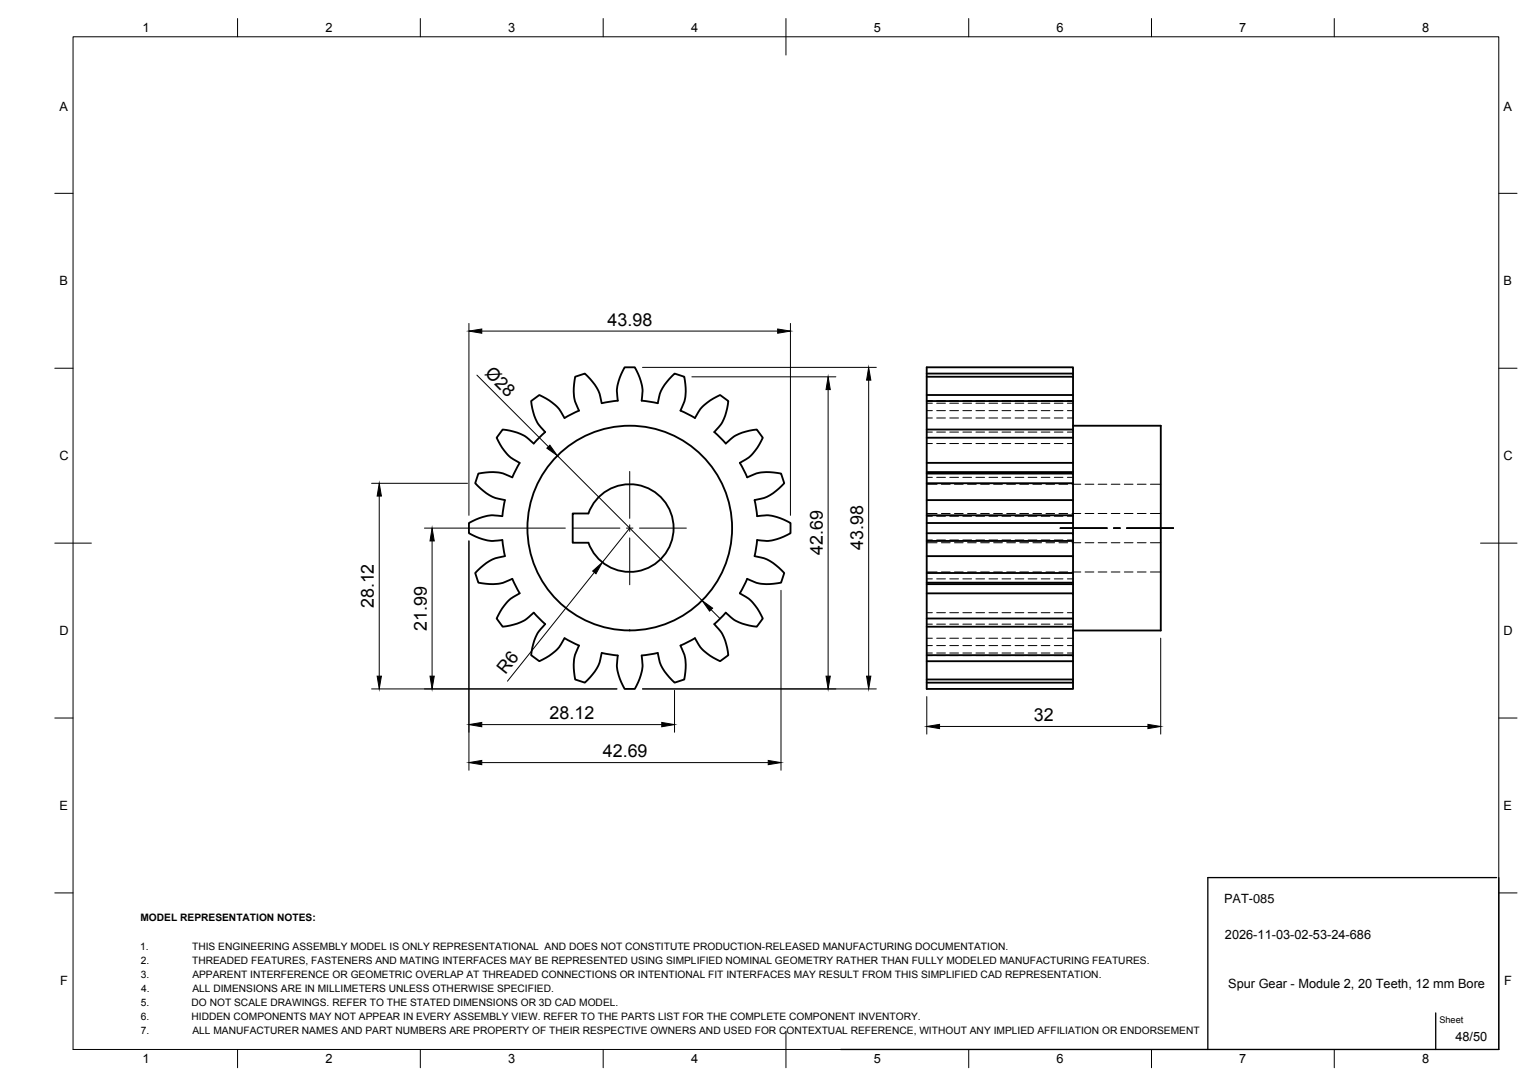
ISO-10303-21;
HEADER;
/* Generated by software containing ST-Developer
 * from STEP Tools, Inc. (www.steptools.com) 
 */

FILE_DESCRIPTION(
/* description */ ('Rack and pinion manual slide'),
/* implementation_level */ '2;1');

FILE_NAME(
/* name */ 'Spur Gear - Module 2, 20 Teeth, 12 mm Bore.step',
/* time_stamp */ '2026-10-28T03:22:49-07:00',
/* author */ (''),
/* organization */ (''),
/* preprocessor_version */ 'ST-DEVELOPER v20.2',
/* originating_system */ 'Autodesk Translation Framework v15.17.0.0',
/* authorisation */ '');

FILE_SCHEMA (('AUTOMOTIVE_DESIGN { 1 0 10303 214 3 1 1 }'));
ENDSEC;

DATA;
#10=MECHANICAL_DESIGN_GEOMETRIC_PRESENTATION_REPRESENTATION('',(#779),#34851);
#11=(
BOUNDED_SURFACE()
B_SPLINE_SURFACE(5,1,((#25778,#25779),(#25780,#25781),(#25782,#25783),(#25784,
#25785),(#25786,#25787),(#25788,#25789),(#25790,#25791),(#25792,#25793),
(#25794,#25795),(#25796,#25797),(#25798,#25799),(#25800,#25801),(#25802,
#25803),(#25804,#25805),(#25806,#25807),(#25808,#25809),(#25810,#25811),
(#25812,#25813),(#25814,#25815),(#25816,#25817),(#25818,#25819),(#25820,
#25821),(#25822,#25823),(#25824,#25825),(#25826,#25827),(#25828,#25829),
(#25830,#25831),(#25832,#25833),(#25834,#25835),(#25836,#25837),(#25838,
#25839),(#25840,#25841),(#25842,#25843),(#25844,#25845),(#25846,#25847),
(#25848,#25849),(#25850,#25851),(#25852,#25853),(#25854,#25855),(#25856,
#25857),(#25858,#25859),(#25860,#25861),(#25862,#25863),(#25864,#25865),
(#25866,#25867),(#25868,#25869),(#25870,#25871),(#25872,#25873),(#25874,
#25875),(#25876,#25877),(#25878,#25879),(#25880,#25881),(#25882,#25883),
(#25884,#25885),(#25886,#25887),(#25888,#25889),(#25890,#25891),(#25892,
#25893),(#25894,#25895),(#25896,#25897),(#25898,#25899),(#25900,#25901),
(#25902,#25903),(#25904,#25905),(#25906,#25907),(#25908,#25909),(#25910,
#25911),(#25912,#25913),(#25914,#25915),(#25916,#25917)),.UNSPECIFIED.,
 .F.,.F.,.F.)
B_SPLINE_SURFACE_WITH_KNOTS((6,1,1,1,1,1,1,1,1,1,1,1,1,1,1,1,1,1,1,1,1,
1,1,1,1,1,1,1,1,1,1,1,1,1,1,1,1,1,1,1,1,1,1,1,1,1,1,1,1,1,1,1,1,1,1,1,1,
1,1,1,1,1,1,1,1,6),(2,2),(-1.,-0.984615384615383,-0.969230769230768,-0.953846153846152,
-0.938461538461537,-0.923076923076922,-0.907692307692306,-0.892307692307691,
-0.876923076923076,-0.86153846153846,-0.846153846153845,-0.83076923076923,
-0.815384615384614,-0.799999999999999,-0.784615384615384,-0.769230769230768,
-0.753846153846153,-0.738461538461538,-0.723076923076922,-0.707692307692307,
-0.692307692307692,-0.676923076923076,-0.661538461538461,-0.646153846153846,
-0.63076923076923,-0.615384615384615,-0.6,-0.584615384615384,-0.569230769230769,
-0.553846153846154,-0.538461538461538,-0.523076923076923,-0.507692307692308,
-0.492307692307692,-0.476923076923077,-0.461538461538462,-0.446153846153846,
-0.430769230769231,-0.415384615384615,-0.4,-0.384615384615385,-0.369230769230769,
-0.353846153846154,-0.338461538461538,-0.323076923076923,-0.307692307692308,
-0.292307692307692,-0.276923076923077,-0.261538461538462,-0.246153846153846,
-0.230769230769231,-0.215384615384615,-0.2,-0.184615384615385,-0.169230769230769,
-0.153846153846154,-0.138461538461538,-0.123076923076923,-0.107692307692308,
-0.0923076923076923,-0.0769230769230769,-0.0615384615384615,-0.0461538461538462,
-0.0307692307692308,-0.0153846153846154,0.),(-1.,1.),.UNSPECIFIED.)
GEOMETRIC_REPRESENTATION_ITEM()
RATIONAL_B_SPLINE_SURFACE(((1.,1.),(1.,1.),(1.,1.),(1.,1.),(1.,1.),(1.,
1.),(1.,1.),(1.,1.),(1.,1.),(1.,1.),(1.,1.),(1.,1.),(1.,1.),(1.,1.),(1.,
1.),(1.,1.),(1.,1.),(1.,1.),(1.,1.),(1.,1.),(1.,1.),(1.,1.),(1.,1.),(1.,
1.),(1.,1.),(1.,1.),(1.,1.),(1.,1.),(1.,1.),(1.,1.),(1.,1.),(1.,1.),(1.,
1.),(1.,1.),(1.,1.),(1.,1.),(1.,1.),(1.,1.),(1.,1.),(1.,1.),(1.,1.),(1.,
1.),(1.,1.),(1.,1.),(1.,1.),(1.,1.),(1.,1.),(1.,1.),(1.,1.),(1.,1.),(1.,
1.),(1.,1.),(1.,1.),(1.,1.),(1.,1.),(1.,1.),(1.,1.),(1.,1.),(1.,1.),(1.,
1.),(1.,1.),(1.,1.),(1.,1.),(1.,1.),(1.,1.),(1.,1.),(1.,1.),(1.,1.),(1.,
1.),(1.,1.)))
REPRESENTATION_ITEM('')
SURFACE()
);
#12=(
BOUNDED_SURFACE()
B_SPLINE_SURFACE(5,1,((#25996,#25997),(#25998,#25999),(#26000,#26001),(#26002,
#26003),(#26004,#26005),(#26006,#26007),(#26008,#26009),(#26010,#26011),
(#26012,#26013),(#26014,#26015),(#26016,#26017),(#26018,#26019),(#26020,
#26021),(#26022,#26023),(#26024,#26025),(#26026,#26027),(#26028,#26029),
(#26030,#26031),(#26032,#26033),(#26034,#26035),(#26036,#26037),(#26038,
#26039),(#26040,#26041),(#26042,#26043),(#26044,#26045),(#26046,#26047),
(#26048,#26049),(#26050,#26051),(#26052,#26053),(#26054,#26055),(#26056,
#26057),(#26058,#26059),(#26060,#26061),(#26062,#26063),(#26064,#26065),
(#26066,#26067),(#26068,#26069),(#26070,#26071),(#26072,#26073),(#26074,
#26075),(#26076,#26077),(#26078,#26079),(#26080,#26081),(#26082,#26083),
(#26084,#26085),(#26086,#26087),(#26088,#26089),(#26090,#26091),(#26092,
#26093),(#26094,#26095),(#26096,#26097),(#26098,#26099),(#26100,#26101),
(#26102,#26103),(#26104,#26105),(#26106,#26107),(#26108,#26109),(#26110,
#26111),(#26112,#26113),(#26114,#26115),(#26116,#26117),(#26118,#26119),
(#26120,#26121),(#26122,#26123),(#26124,#26125),(#26126,#26127),(#26128,
#26129),(#26130,#26131),(#26132,#26133),(#26134,#26135)),.UNSPECIFIED.,
 .F.,.F.,.F.)
B_SPLINE_SURFACE_WITH_KNOTS((6,1,1,1,1,1,1,1,1,1,1,1,1,1,1,1,1,1,1,1,1,
1,1,1,1,1,1,1,1,1,1,1,1,1,1,1,1,1,1,1,1,1,1,1,1,1,1,1,1,1,1,1,1,1,1,1,1,
1,1,1,1,1,1,1,1,6),(2,2),(-1.,-0.984615384615383,-0.969230769230768,-0.953846153846152,
-0.938461538461537,-0.923076923076922,-0.907692307692306,-0.892307692307691,
-0.876923076923076,-0.86153846153846,-0.846153846153845,-0.83076923076923,
-0.815384615384614,-0.799999999999999,-0.784615384615384,-0.769230769230768,
-0.753846153846153,-0.738461538461538,-0.723076923076922,-0.707692307692307,
-0.692307692307692,-0.676923076923076,-0.661538461538461,-0.646153846153846,
-0.63076923076923,-0.615384615384615,-0.6,-0.584615384615384,-0.569230769230769,
-0.553846153846154,-0.538461538461538,-0.523076923076923,-0.507692307692308,
-0.492307692307692,-0.476923076923077,-0.461538461538462,-0.446153846153846,
-0.430769230769231,-0.415384615384615,-0.4,-0.384615384615385,-0.369230769230769,
-0.353846153846154,-0.338461538461538,-0.323076923076923,-0.307692307692308,
-0.292307692307692,-0.276923076923077,-0.261538461538462,-0.246153846153846,
-0.230769230769231,-0.215384615384615,-0.2,-0.184615384615385,-0.169230769230769,
-0.153846153846154,-0.138461538461538,-0.123076923076923,-0.107692307692308,
-0.0923076923076923,-0.0769230769230769,-0.0615384615384615,-0.0461538461538462,
-0.0307692307692308,-0.0153846153846154,0.),(-1.,1.),.UNSPECIFIED.)
GEOMETRIC_REPRESENTATION_ITEM()
RATIONAL_B_SPLINE_SURFACE(((1.,1.),(1.,1.),(1.,1.),(1.,1.),(1.,1.),(1.,
1.),(1.,1.),(1.,1.),(1.,1.),(1.,1.),(1.,1.),(1.,1.),(1.,1.),(1.,1.),(1.,
1.),(1.,1.),(1.,1.),(1.,1.),(1.,1.),(1.,1.),(1.,1.),(1.,1.),(1.,1.),(1.,
1.),(1.,1.),(1.,1.),(1.,1.),(1.,1.),(1.,1.),(1.,1.),(1.,1.),(1.,1.),(1.,
1.),(1.,1.),(1.,1.),(1.,1.),(1.,1.),(1.,1.),(1.,1.),(1.,1.),(1.,1.),(1.,
1.),(1.,1.),(1.,1.),(1.,1.),(1.,1.),(1.,1.),(1.,1.),(1.,1.),(1.,1.),(1.,
1.),(1.,1.),(1.,1.),(1.,1.),(1.,1.),(1.,1.),(1.,1.),(1.,1.),(1.,1.),(1.,
1.),(1.,1.),(1.,1.),(1.,1.),(1.,1.),(1.,1.),(1.,1.),(1.,1.),(1.,1.),(1.,
1.),(1.,1.)))
REPRESENTATION_ITEM('')
SURFACE()
);
#13=(
BOUNDED_SURFACE()
B_SPLINE_SURFACE(5,1,((#26212,#26213),(#26214,#26215),(#26216,#26217),(#26218,
#26219),(#26220,#26221),(#26222,#26223),(#26224,#26225),(#26226,#26227),
(#26228,#26229),(#26230,#26231),(#26232,#26233),(#26234,#26235),(#26236,
#26237),(#26238,#26239),(#26240,#26241),(#26242,#26243),(#26244,#26245),
(#26246,#26247),(#26248,#26249),(#26250,#26251),(#26252,#26253),(#26254,
#26255),(#26256,#26257),(#26258,#26259),(#26260,#26261),(#26262,#26263),
(#26264,#26265),(#26266,#26267),(#26268,#26269),(#26270,#26271),(#26272,
#26273),(#26274,#26275),(#26276,#26277),(#26278,#26279),(#26280,#26281),
(#26282,#26283),(#26284,#26285),(#26286,#26287),(#26288,#26289),(#26290,
#26291),(#26292,#26293),(#26294,#26295),(#26296,#26297),(#26298,#26299),
(#26300,#26301),(#26302,#26303),(#26304,#26305),(#26306,#26307),(#26308,
#26309),(#26310,#26311),(#26312,#26313),(#26314,#26315),(#26316,#26317),
(#26318,#26319),(#26320,#26321),(#26322,#26323),(#26324,#26325),(#26326,
#26327),(#26328,#26329),(#26330,#26331),(#26332,#26333),(#26334,#26335),
(#26336,#26337),(#26338,#26339),(#26340,#26341),(#26342,#26343),(#26344,
#26345),(#26346,#26347),(#26348,#26349),(#26350,#26351)),.UNSPECIFIED.,
 .F.,.F.,.F.)
B_SPLINE_SURFACE_WITH_KNOTS((6,1,1,1,1,1,1,1,1,1,1,1,1,1,1,1,1,1,1,1,1,
1,1,1,1,1,1,1,1,1,1,1,1,1,1,1,1,1,1,1,1,1,1,1,1,1,1,1,1,1,1,1,1,1,1,1,1,
1,1,1,1,1,1,1,1,6),(2,2),(-1.,-0.984615384615383,-0.969230769230768,-0.953846153846152,
-0.938461538461537,-0.923076923076922,-0.907692307692306,-0.892307692307691,
-0.876923076923076,-0.86153846153846,-0.846153846153845,-0.83076923076923,
-0.815384615384614,-0.799999999999999,-0.784615384615384,-0.769230769230768,
-0.753846153846153,-0.738461538461538,-0.723076923076922,-0.707692307692307,
-0.692307692307692,-0.676923076923076,-0.661538461538461,-0.646153846153846,
-0.63076923076923,-0.615384615384615,-0.6,-0.584615384615384,-0.569230769230769,
-0.553846153846154,-0.538461538461538,-0.523076923076923,-0.507692307692308,
-0.492307692307692,-0.476923076923077,-0.461538461538462,-0.446153846153846,
-0.430769230769231,-0.415384615384615,-0.4,-0.384615384615385,-0.369230769230769,
-0.353846153846154,-0.338461538461538,-0.323076923076923,-0.307692307692308,
-0.292307692307692,-0.276923076923077,-0.261538461538462,-0.246153846153846,
-0.230769230769231,-0.215384615384615,-0.2,-0.184615384615385,-0.169230769230769,
-0.153846153846154,-0.138461538461538,-0.123076923076923,-0.107692307692308,
-0.0923076923076923,-0.0769230769230769,-0.0615384615384615,-0.0461538461538462,
-0.0307692307692308,-0.0153846153846154,0.),(-1.,1.),.UNSPECIFIED.)
GEOMETRIC_REPRESENTATION_ITEM()
RATIONAL_B_SPLINE_SURFACE(((1.,1.),(1.,1.),(1.,1.),(1.,1.),(1.,1.),(1.,
1.),(1.,1.),(1.,1.),(1.,1.),(1.,1.),(1.,1.),(1.,1.),(1.,1.),(1.,1.),(1.,
1.),(1.,1.),(1.,1.),(1.,1.),(1.,1.),(1.,1.),(1.,1.),(1.,1.),(1.,1.),(1.,
1.),(1.,1.),(1.,1.),(1.,1.),(1.,1.),(1.,1.),(1.,1.),(1.,1.),(1.,1.),(1.,
1.),(1.,1.),(1.,1.),(1.,1.),(1.,1.),(1.,1.),(1.,1.),(1.,1.),(1.,1.),(1.,
1.),(1.,1.),(1.,1.),(1.,1.),(1.,1.),(1.,1.),(1.,1.),(1.,1.),(1.,1.),(1.,
1.),(1.,1.),(1.,1.),(1.,1.),(1.,1.),(1.,1.),(1.,1.),(1.,1.),(1.,1.),(1.,
1.),(1.,1.),(1.,1.),(1.,1.),(1.,1.),(1.,1.),(1.,1.),(1.,1.),(1.,1.),(1.,
1.),(1.,1.)))
REPRESENTATION_ITEM('')
SURFACE()
);
#14=(
BOUNDED_SURFACE()
B_SPLINE_SURFACE(5,1,((#26428,#26429),(#26430,#26431),(#26432,#26433),(#26434,
#26435),(#26436,#26437),(#26438,#26439),(#26440,#26441),(#26442,#26443),
(#26444,#26445),(#26446,#26447),(#26448,#26449),(#26450,#26451),(#26452,
#26453),(#26454,#26455),(#26456,#26457),(#26458,#26459),(#26460,#26461),
(#26462,#26463),(#26464,#26465),(#26466,#26467),(#26468,#26469),(#26470,
#26471),(#26472,#26473),(#26474,#26475),(#26476,#26477),(#26478,#26479),
(#26480,#26481),(#26482,#26483),(#26484,#26485),(#26486,#26487),(#26488,
#26489),(#26490,#26491),(#26492,#26493),(#26494,#26495),(#26496,#26497),
(#26498,#26499),(#26500,#26501),(#26502,#26503),(#26504,#26505),(#26506,
#26507),(#26508,#26509),(#26510,#26511),(#26512,#26513),(#26514,#26515),
(#26516,#26517),(#26518,#26519),(#26520,#26521),(#26522,#26523),(#26524,
#26525),(#26526,#26527),(#26528,#26529),(#26530,#26531),(#26532,#26533),
(#26534,#26535),(#26536,#26537),(#26538,#26539),(#26540,#26541),(#26542,
#26543),(#26544,#26545),(#26546,#26547),(#26548,#26549),(#26550,#26551),
(#26552,#26553),(#26554,#26555),(#26556,#26557),(#26558,#26559),(#26560,
#26561),(#26562,#26563),(#26564,#26565),(#26566,#26567)),.UNSPECIFIED.,
 .F.,.F.,.F.)
B_SPLINE_SURFACE_WITH_KNOTS((6,1,1,1,1,1,1,1,1,1,1,1,1,1,1,1,1,1,1,1,1,
1,1,1,1,1,1,1,1,1,1,1,1,1,1,1,1,1,1,1,1,1,1,1,1,1,1,1,1,1,1,1,1,1,1,1,1,
1,1,1,1,1,1,1,1,6),(2,2),(-1.,-0.984615384615383,-0.969230769230768,-0.953846153846152,
-0.938461538461537,-0.923076923076922,-0.907692307692306,-0.892307692307691,
-0.876923076923076,-0.86153846153846,-0.846153846153845,-0.83076923076923,
-0.815384615384614,-0.799999999999999,-0.784615384615384,-0.769230769230768,
-0.753846153846153,-0.738461538461538,-0.723076923076922,-0.707692307692307,
-0.692307692307692,-0.676923076923076,-0.661538461538461,-0.646153846153846,
-0.63076923076923,-0.615384615384615,-0.6,-0.584615384615384,-0.569230769230769,
-0.553846153846154,-0.538461538461538,-0.523076923076923,-0.507692307692308,
-0.492307692307692,-0.476923076923077,-0.461538461538462,-0.446153846153846,
-0.430769230769231,-0.415384615384615,-0.4,-0.384615384615385,-0.369230769230769,
-0.353846153846154,-0.338461538461538,-0.323076923076923,-0.307692307692308,
-0.292307692307692,-0.276923076923077,-0.261538461538462,-0.246153846153846,
-0.230769230769231,-0.215384615384615,-0.2,-0.184615384615385,-0.169230769230769,
-0.153846153846154,-0.138461538461538,-0.123076923076923,-0.107692307692308,
-0.0923076923076923,-0.0769230769230769,-0.0615384615384615,-0.0461538461538462,
-0.0307692307692308,-0.0153846153846154,0.),(-1.,1.),.UNSPECIFIED.)
GEOMETRIC_REPRESENTATION_ITEM()
RATIONAL_B_SPLINE_SURFACE(((1.,1.),(1.,1.),(1.,1.),(1.,1.),(1.,1.),(1.,
1.),(1.,1.),(1.,1.),(1.,1.),(1.,1.),(1.,1.),(1.,1.),(1.,1.),(1.,1.),(1.,
1.),(1.,1.),(1.,1.),(1.,1.),(1.,1.),(1.,1.),(1.,1.),(1.,1.),(1.,1.),(1.,
1.),(1.,1.),(1.,1.),(1.,1.),(1.,1.),(1.,1.),(1.,1.),(1.,1.),(1.,1.),(1.,
1.),(1.,1.),(1.,1.),(1.,1.),(1.,1.),(1.,1.),(1.,1.),(1.,1.),(1.,1.),(1.,
1.),(1.,1.),(1.,1.),(1.,1.),(1.,1.),(1.,1.),(1.,1.),(1.,1.),(1.,1.),(1.,
1.),(1.,1.),(1.,1.),(1.,1.),(1.,1.),(1.,1.),(1.,1.),(1.,1.),(1.,1.),(1.,
1.),(1.,1.),(1.,1.),(1.,1.),(1.,1.),(1.,1.),(1.,1.),(1.,1.),(1.,1.),(1.,
1.),(1.,1.)))
REPRESENTATION_ITEM('')
SURFACE()
);
#15=(
BOUNDED_SURFACE()
B_SPLINE_SURFACE(5,1,((#26644,#26645),(#26646,#26647),(#26648,#26649),(#26650,
#26651),(#26652,#26653),(#26654,#26655),(#26656,#26657),(#26658,#26659),
(#26660,#26661),(#26662,#26663),(#26664,#26665),(#26666,#26667),(#26668,
#26669),(#26670,#26671),(#26672,#26673),(#26674,#26675),(#26676,#26677),
(#26678,#26679),(#26680,#26681),(#26682,#26683),(#26684,#26685),(#26686,
#26687),(#26688,#26689),(#26690,#26691),(#26692,#26693),(#26694,#26695),
(#26696,#26697),(#26698,#26699),(#26700,#26701),(#26702,#26703),(#26704,
#26705),(#26706,#26707),(#26708,#26709),(#26710,#26711),(#26712,#26713),
(#26714,#26715),(#26716,#26717),(#26718,#26719),(#26720,#26721),(#26722,
#26723),(#26724,#26725),(#26726,#26727),(#26728,#26729),(#26730,#26731),
(#26732,#26733),(#26734,#26735),(#26736,#26737),(#26738,#26739),(#26740,
#26741),(#26742,#26743),(#26744,#26745),(#26746,#26747),(#26748,#26749),
(#26750,#26751),(#26752,#26753),(#26754,#26755),(#26756,#26757),(#26758,
#26759),(#26760,#26761),(#26762,#26763),(#26764,#26765),(#26766,#26767),
(#26768,#26769),(#26770,#26771),(#26772,#26773),(#26774,#26775),(#26776,
#26777),(#26778,#26779),(#26780,#26781),(#26782,#26783)),.UNSPECIFIED.,
 .F.,.F.,.F.)
B_SPLINE_SURFACE_WITH_KNOTS((6,1,1,1,1,1,1,1,1,1,1,1,1,1,1,1,1,1,1,1,1,
1,1,1,1,1,1,1,1,1,1,1,1,1,1,1,1,1,1,1,1,1,1,1,1,1,1,1,1,1,1,1,1,1,1,1,1,
1,1,1,1,1,1,1,1,6),(2,2),(-1.,-0.984615384615383,-0.969230769230768,-0.953846153846152,
-0.938461538461537,-0.923076923076922,-0.907692307692306,-0.892307692307691,
-0.876923076923076,-0.86153846153846,-0.846153846153845,-0.83076923076923,
-0.815384615384614,-0.799999999999999,-0.784615384615384,-0.769230769230768,
-0.753846153846153,-0.738461538461538,-0.723076923076922,-0.707692307692307,
-0.692307692307692,-0.676923076923076,-0.661538461538461,-0.646153846153846,
-0.63076923076923,-0.615384615384615,-0.6,-0.584615384615384,-0.569230769230769,
-0.553846153846154,-0.538461538461538,-0.523076923076923,-0.507692307692308,
-0.492307692307692,-0.476923076923077,-0.461538461538462,-0.446153846153846,
-0.430769230769231,-0.415384615384615,-0.4,-0.384615384615385,-0.369230769230769,
-0.353846153846154,-0.338461538461538,-0.323076923076923,-0.307692307692308,
-0.292307692307692,-0.276923076923077,-0.261538461538462,-0.246153846153846,
-0.230769230769231,-0.215384615384615,-0.2,-0.184615384615385,-0.169230769230769,
-0.153846153846154,-0.138461538461538,-0.123076923076923,-0.107692307692308,
-0.0923076923076923,-0.0769230769230769,-0.0615384615384615,-0.0461538461538462,
-0.0307692307692308,-0.0153846153846154,0.),(-1.,1.),.UNSPECIFIED.)
GEOMETRIC_REPRESENTATION_ITEM()
RATIONAL_B_SPLINE_SURFACE(((1.,1.),(1.,1.),(1.,1.),(1.,1.),(1.,1.),(1.,
1.),(1.,1.),(1.,1.),(1.,1.),(1.,1.),(1.,1.),(1.,1.),(1.,1.),(1.,1.),(1.,
1.),(1.,1.),(1.,1.),(1.,1.),(1.,1.),(1.,1.),(1.,1.),(1.,1.),(1.,1.),(1.,
1.),(1.,1.),(1.,1.),(1.,1.),(1.,1.),(1.,1.),(1.,1.),(1.,1.),(1.,1.),(1.,
1.),(1.,1.),(1.,1.),(1.,1.),(1.,1.),(1.,1.),(1.,1.),(1.,1.),(1.,1.),(1.,
1.),(1.,1.),(1.,1.),(1.,1.),(1.,1.),(1.,1.),(1.,1.),(1.,1.),(1.,1.),(1.,
1.),(1.,1.),(1.,1.),(1.,1.),(1.,1.),(1.,1.),(1.,1.),(1.,1.),(1.,1.),(1.,
1.),(1.,1.),(1.,1.),(1.,1.),(1.,1.),(1.,1.),(1.,1.),(1.,1.),(1.,1.),(1.,
1.),(1.,1.)))
REPRESENTATION_ITEM('')
SURFACE()
);
#16=(
BOUNDED_SURFACE()
B_SPLINE_SURFACE(5,1,((#26860,#26861),(#26862,#26863),(#26864,#26865),(#26866,
#26867),(#26868,#26869),(#26870,#26871),(#26872,#26873),(#26874,#26875),
(#26876,#26877),(#26878,#26879),(#26880,#26881),(#26882,#26883),(#26884,
#26885),(#26886,#26887),(#26888,#26889),(#26890,#26891),(#26892,#26893),
(#26894,#26895),(#26896,#26897),(#26898,#26899),(#26900,#26901),(#26902,
#26903),(#26904,#26905),(#26906,#26907),(#26908,#26909),(#26910,#26911),
(#26912,#26913),(#26914,#26915),(#26916,#26917),(#26918,#26919),(#26920,
#26921),(#26922,#26923),(#26924,#26925),(#26926,#26927),(#26928,#26929),
(#26930,#26931),(#26932,#26933),(#26934,#26935),(#26936,#26937),(#26938,
#26939),(#26940,#26941),(#26942,#26943),(#26944,#26945),(#26946,#26947),
(#26948,#26949),(#26950,#26951),(#26952,#26953),(#26954,#26955),(#26956,
#26957),(#26958,#26959),(#26960,#26961),(#26962,#26963),(#26964,#26965),
(#26966,#26967),(#26968,#26969),(#26970,#26971),(#26972,#26973),(#26974,
#26975),(#26976,#26977),(#26978,#26979),(#26980,#26981),(#26982,#26983),
(#26984,#26985),(#26986,#26987),(#26988,#26989),(#26990,#26991),(#26992,
#26993),(#26994,#26995),(#26996,#26997),(#26998,#26999)),.UNSPECIFIED.,
 .F.,.F.,.F.)
B_SPLINE_SURFACE_WITH_KNOTS((6,1,1,1,1,1,1,1,1,1,1,1,1,1,1,1,1,1,1,1,1,
1,1,1,1,1,1,1,1,1,1,1,1,1,1,1,1,1,1,1,1,1,1,1,1,1,1,1,1,1,1,1,1,1,1,1,1,
1,1,1,1,1,1,1,1,6),(2,2),(-1.,-0.984615384615383,-0.969230769230768,-0.953846153846152,
-0.938461538461537,-0.923076923076922,-0.907692307692306,-0.892307692307691,
-0.876923076923076,-0.86153846153846,-0.846153846153845,-0.83076923076923,
-0.815384615384614,-0.799999999999999,-0.784615384615384,-0.769230769230768,
-0.753846153846153,-0.738461538461538,-0.723076923076922,-0.707692307692307,
-0.692307692307692,-0.676923076923076,-0.661538461538461,-0.646153846153846,
-0.63076923076923,-0.615384615384615,-0.6,-0.584615384615384,-0.569230769230769,
-0.553846153846154,-0.538461538461538,-0.523076923076923,-0.507692307692308,
-0.492307692307692,-0.476923076923077,-0.461538461538462,-0.446153846153846,
-0.430769230769231,-0.415384615384615,-0.4,-0.384615384615385,-0.369230769230769,
-0.353846153846154,-0.338461538461538,-0.323076923076923,-0.307692307692308,
-0.292307692307692,-0.276923076923077,-0.261538461538462,-0.246153846153846,
-0.230769230769231,-0.215384615384615,-0.2,-0.184615384615385,-0.169230769230769,
-0.153846153846154,-0.138461538461538,-0.123076923076923,-0.107692307692308,
-0.0923076923076923,-0.0769230769230769,-0.0615384615384615,-0.0461538461538462,
-0.0307692307692308,-0.0153846153846154,0.),(-1.,1.),.UNSPECIFIED.)
GEOMETRIC_REPRESENTATION_ITEM()
RATIONAL_B_SPLINE_SURFACE(((1.,1.),(1.,1.),(1.,1.),(1.,1.),(1.,1.),(1.,
1.),(1.,1.),(1.,1.),(1.,1.),(1.,1.),(1.,1.),(1.,1.),(1.,1.),(1.,1.),(1.,
1.),(1.,1.),(1.,1.),(1.,1.),(1.,1.),(1.,1.),(1.,1.),(1.,1.),(1.,1.),(1.,
1.),(1.,1.),(1.,1.),(1.,1.),(1.,1.),(1.,1.),(1.,1.),(1.,1.),(1.,1.),(1.,
1.),(1.,1.),(1.,1.),(1.,1.),(1.,1.),(1.,1.),(1.,1.),(1.,1.),(1.,1.),(1.,
1.),(1.,1.),(1.,1.),(1.,1.),(1.,1.),(1.,1.),(1.,1.),(1.,1.),(1.,1.),(1.,
1.),(1.,1.),(1.,1.),(1.,1.),(1.,1.),(1.,1.),(1.,1.),(1.,1.),(1.,1.),(1.,
1.),(1.,1.),(1.,1.),(1.,1.),(1.,1.),(1.,1.),(1.,1.),(1.,1.),(1.,1.),(1.,
1.),(1.,1.)))
REPRESENTATION_ITEM('')
SURFACE()
);
#17=(
BOUNDED_SURFACE()
B_SPLINE_SURFACE(5,1,((#27076,#27077),(#27078,#27079),(#27080,#27081),(#27082,
#27083),(#27084,#27085),(#27086,#27087),(#27088,#27089),(#27090,#27091),
(#27092,#27093),(#27094,#27095),(#27096,#27097),(#27098,#27099),(#27100,
#27101),(#27102,#27103),(#27104,#27105),(#27106,#27107),(#27108,#27109),
(#27110,#27111),(#27112,#27113),(#27114,#27115),(#27116,#27117),(#27118,
#27119),(#27120,#27121),(#27122,#27123),(#27124,#27125),(#27126,#27127),
(#27128,#27129),(#27130,#27131),(#27132,#27133),(#27134,#27135),(#27136,
#27137),(#27138,#27139),(#27140,#27141),(#27142,#27143),(#27144,#27145),
(#27146,#27147),(#27148,#27149),(#27150,#27151),(#27152,#27153),(#27154,
#27155),(#27156,#27157),(#27158,#27159),(#27160,#27161),(#27162,#27163),
(#27164,#27165),(#27166,#27167),(#27168,#27169),(#27170,#27171),(#27172,
#27173),(#27174,#27175),(#27176,#27177),(#27178,#27179),(#27180,#27181),
(#27182,#27183),(#27184,#27185),(#27186,#27187),(#27188,#27189),(#27190,
#27191),(#27192,#27193),(#27194,#27195),(#27196,#27197),(#27198,#27199),
(#27200,#27201),(#27202,#27203),(#27204,#27205),(#27206,#27207),(#27208,
#27209),(#27210,#27211),(#27212,#27213),(#27214,#27215)),.UNSPECIFIED.,
 .F.,.F.,.F.)
B_SPLINE_SURFACE_WITH_KNOTS((6,1,1,1,1,1,1,1,1,1,1,1,1,1,1,1,1,1,1,1,1,
1,1,1,1,1,1,1,1,1,1,1,1,1,1,1,1,1,1,1,1,1,1,1,1,1,1,1,1,1,1,1,1,1,1,1,1,
1,1,1,1,1,1,1,1,6),(2,2),(-1.,-0.984615384615383,-0.969230769230768,-0.953846153846152,
-0.938461538461537,-0.923076923076922,-0.907692307692306,-0.892307692307691,
-0.876923076923076,-0.86153846153846,-0.846153846153845,-0.83076923076923,
-0.815384615384614,-0.799999999999999,-0.784615384615384,-0.769230769230768,
-0.753846153846153,-0.738461538461538,-0.723076923076922,-0.707692307692307,
-0.692307692307692,-0.676923076923076,-0.661538461538461,-0.646153846153846,
-0.63076923076923,-0.615384615384615,-0.6,-0.584615384615384,-0.569230769230769,
-0.553846153846154,-0.538461538461538,-0.523076923076923,-0.507692307692308,
-0.492307692307692,-0.476923076923077,-0.461538461538462,-0.446153846153846,
-0.430769230769231,-0.415384615384615,-0.4,-0.384615384615385,-0.369230769230769,
-0.353846153846154,-0.338461538461538,-0.323076923076923,-0.307692307692308,
-0.292307692307692,-0.276923076923077,-0.261538461538462,-0.246153846153846,
-0.230769230769231,-0.215384615384615,-0.2,-0.184615384615385,-0.169230769230769,
-0.153846153846154,-0.138461538461538,-0.123076923076923,-0.107692307692308,
-0.0923076923076923,-0.0769230769230769,-0.0615384615384615,-0.0461538461538462,
-0.0307692307692308,-0.0153846153846154,0.),(-1.,1.),.UNSPECIFIED.)
GEOMETRIC_REPRESENTATION_ITEM()
RATIONAL_B_SPLINE_SURFACE(((1.,1.),(1.,1.),(1.,1.),(1.,1.),(1.,1.),(1.,
1.),(1.,1.),(1.,1.),(1.,1.),(1.,1.),(1.,1.),(1.,1.),(1.,1.),(1.,1.),(1.,
1.),(1.,1.),(1.,1.),(1.,1.),(1.,1.),(1.,1.),(1.,1.),(1.,1.),(1.,1.),(1.,
1.),(1.,1.),(1.,1.),(1.,1.),(1.,1.),(1.,1.),(1.,1.),(1.,1.),(1.,1.),(1.,
1.),(1.,1.),(1.,1.),(1.,1.),(1.,1.),(1.,1.),(1.,1.),(1.,1.),(1.,1.),(1.,
1.),(1.,1.),(1.,1.),(1.,1.),(1.,1.),(1.,1.),(1.,1.),(1.,1.),(1.,1.),(1.,
1.),(1.,1.),(1.,1.),(1.,1.),(1.,1.),(1.,1.),(1.,1.),(1.,1.),(1.,1.),(1.,
1.),(1.,1.),(1.,1.),(1.,1.),(1.,1.),(1.,1.),(1.,1.),(1.,1.),(1.,1.),(1.,
1.),(1.,1.)))
REPRESENTATION_ITEM('')
SURFACE()
);
#18=(
BOUNDED_SURFACE()
B_SPLINE_SURFACE(5,1,((#27292,#27293),(#27294,#27295),(#27296,#27297),(#27298,
#27299),(#27300,#27301),(#27302,#27303),(#27304,#27305),(#27306,#27307),
(#27308,#27309),(#27310,#27311),(#27312,#27313),(#27314,#27315),(#27316,
#27317),(#27318,#27319),(#27320,#27321),(#27322,#27323),(#27324,#27325),
(#27326,#27327),(#27328,#27329),(#27330,#27331),(#27332,#27333),(#27334,
#27335),(#27336,#27337),(#27338,#27339),(#27340,#27341),(#27342,#27343),
(#27344,#27345),(#27346,#27347),(#27348,#27349),(#27350,#27351),(#27352,
#27353),(#27354,#27355),(#27356,#27357),(#27358,#27359),(#27360,#27361),
(#27362,#27363),(#27364,#27365),(#27366,#27367),(#27368,#27369),(#27370,
#27371),(#27372,#27373),(#27374,#27375),(#27376,#27377),(#27378,#27379),
(#27380,#27381),(#27382,#27383),(#27384,#27385),(#27386,#27387),(#27388,
#27389),(#27390,#27391),(#27392,#27393),(#27394,#27395),(#27396,#27397),
(#27398,#27399),(#27400,#27401),(#27402,#27403),(#27404,#27405),(#27406,
#27407),(#27408,#27409),(#27410,#27411),(#27412,#27413),(#27414,#27415),
(#27416,#27417),(#27418,#27419),(#27420,#27421),(#27422,#27423),(#27424,
#27425),(#27426,#27427),(#27428,#27429),(#27430,#27431)),.UNSPECIFIED.,
 .F.,.F.,.F.)
B_SPLINE_SURFACE_WITH_KNOTS((6,1,1,1,1,1,1,1,1,1,1,1,1,1,1,1,1,1,1,1,1,
1,1,1,1,1,1,1,1,1,1,1,1,1,1,1,1,1,1,1,1,1,1,1,1,1,1,1,1,1,1,1,1,1,1,1,1,
1,1,1,1,1,1,1,1,6),(2,2),(-1.,-0.984615384615383,-0.969230769230768,-0.953846153846152,
-0.938461538461537,-0.923076923076922,-0.907692307692306,-0.892307692307691,
-0.876923076923076,-0.86153846153846,-0.846153846153845,-0.83076923076923,
-0.815384615384614,-0.799999999999999,-0.784615384615384,-0.769230769230768,
-0.753846153846153,-0.738461538461538,-0.723076923076922,-0.707692307692307,
-0.692307692307692,-0.676923076923076,-0.661538461538461,-0.646153846153846,
-0.63076923076923,-0.615384615384615,-0.6,-0.584615384615384,-0.569230769230769,
-0.553846153846154,-0.538461538461538,-0.523076923076923,-0.507692307692308,
-0.492307692307692,-0.476923076923077,-0.461538461538462,-0.446153846153846,
-0.430769230769231,-0.415384615384615,-0.4,-0.384615384615385,-0.369230769230769,
-0.353846153846154,-0.338461538461538,-0.323076923076923,-0.307692307692308,
-0.292307692307692,-0.276923076923077,-0.261538461538462,-0.246153846153846,
-0.230769230769231,-0.215384615384615,-0.2,-0.184615384615385,-0.169230769230769,
-0.153846153846154,-0.138461538461538,-0.123076923076923,-0.107692307692308,
-0.0923076923076923,-0.0769230769230769,-0.0615384615384615,-0.0461538461538462,
-0.0307692307692308,-0.0153846153846154,0.),(-1.,1.),.UNSPECIFIED.)
GEOMETRIC_REPRESENTATION_ITEM()
RATIONAL_B_SPLINE_SURFACE(((1.,1.),(1.,1.),(1.,1.),(1.,1.),(1.,1.),(1.,
1.),(1.,1.),(1.,1.),(1.,1.),(1.,1.),(1.,1.),(1.,1.),(1.,1.),(1.,1.),(1.,
1.),(1.,1.),(1.,1.),(1.,1.),(1.,1.),(1.,1.),(1.,1.),(1.,1.),(1.,1.),(1.,
1.),(1.,1.),(1.,1.),(1.,1.),(1.,1.),(1.,1.),(1.,1.),(1.,1.),(1.,1.),(1.,
1.),(1.,1.),(1.,1.),(1.,1.),(1.,1.),(1.,1.),(1.,1.),(1.,1.),(1.,1.),(1.,
1.),(1.,1.),(1.,1.),(1.,1.),(1.,1.),(1.,1.),(1.,1.),(1.,1.),(1.,1.),(1.,
1.),(1.,1.),(1.,1.),(1.,1.),(1.,1.),(1.,1.),(1.,1.),(1.,1.),(1.,1.),(1.,
1.),(1.,1.),(1.,1.),(1.,1.),(1.,1.),(1.,1.),(1.,1.),(1.,1.),(1.,1.),(1.,
1.),(1.,1.)))
REPRESENTATION_ITEM('')
SURFACE()
);
#19=(
BOUNDED_SURFACE()
B_SPLINE_SURFACE(5,1,((#27508,#27509),(#27510,#27511),(#27512,#27513),(#27514,
#27515),(#27516,#27517),(#27518,#27519),(#27520,#27521),(#27522,#27523),
(#27524,#27525),(#27526,#27527),(#27528,#27529),(#27530,#27531),(#27532,
#27533),(#27534,#27535),(#27536,#27537),(#27538,#27539),(#27540,#27541),
(#27542,#27543),(#27544,#27545),(#27546,#27547),(#27548,#27549),(#27550,
#27551),(#27552,#27553),(#27554,#27555),(#27556,#27557),(#27558,#27559),
(#27560,#27561),(#27562,#27563),(#27564,#27565),(#27566,#27567),(#27568,
#27569),(#27570,#27571),(#27572,#27573),(#27574,#27575),(#27576,#27577),
(#27578,#27579),(#27580,#27581),(#27582,#27583),(#27584,#27585),(#27586,
#27587),(#27588,#27589),(#27590,#27591),(#27592,#27593),(#27594,#27595),
(#27596,#27597),(#27598,#27599),(#27600,#27601),(#27602,#27603),(#27604,
#27605),(#27606,#27607),(#27608,#27609),(#27610,#27611),(#27612,#27613),
(#27614,#27615),(#27616,#27617),(#27618,#27619),(#27620,#27621),(#27622,
#27623),(#27624,#27625),(#27626,#27627),(#27628,#27629),(#27630,#27631),
(#27632,#27633),(#27634,#27635),(#27636,#27637),(#27638,#27639),(#27640,
#27641),(#27642,#27643),(#27644,#27645),(#27646,#27647)),.UNSPECIFIED.,
 .F.,.F.,.F.)
B_SPLINE_SURFACE_WITH_KNOTS((6,1,1,1,1,1,1,1,1,1,1,1,1,1,1,1,1,1,1,1,1,
1,1,1,1,1,1,1,1,1,1,1,1,1,1,1,1,1,1,1,1,1,1,1,1,1,1,1,1,1,1,1,1,1,1,1,1,
1,1,1,1,1,1,1,1,6),(2,2),(-1.,-0.984615384615383,-0.969230769230768,-0.953846153846152,
-0.938461538461537,-0.923076923076922,-0.907692307692306,-0.892307692307691,
-0.876923076923076,-0.86153846153846,-0.846153846153845,-0.83076923076923,
-0.815384615384614,-0.799999999999999,-0.784615384615384,-0.769230769230768,
-0.753846153846153,-0.738461538461538,-0.723076923076922,-0.707692307692307,
-0.692307692307692,-0.676923076923076,-0.661538461538461,-0.646153846153846,
-0.63076923076923,-0.615384615384615,-0.6,-0.584615384615384,-0.569230769230769,
-0.553846153846154,-0.538461538461538,-0.523076923076923,-0.507692307692308,
-0.492307692307692,-0.476923076923077,-0.461538461538462,-0.446153846153846,
-0.430769230769231,-0.415384615384615,-0.4,-0.384615384615385,-0.369230769230769,
-0.353846153846154,-0.338461538461538,-0.323076923076923,-0.307692307692308,
-0.292307692307692,-0.276923076923077,-0.261538461538462,-0.246153846153846,
-0.230769230769231,-0.215384615384615,-0.2,-0.184615384615385,-0.169230769230769,
-0.153846153846154,-0.138461538461538,-0.123076923076923,-0.107692307692308,
-0.0923076923076923,-0.0769230769230769,-0.0615384615384615,-0.0461538461538462,
-0.0307692307692308,-0.0153846153846154,0.),(-1.,1.),.UNSPECIFIED.)
GEOMETRIC_REPRESENTATION_ITEM()
RATIONAL_B_SPLINE_SURFACE(((1.,1.),(1.,1.),(1.,1.),(1.,1.),(1.,1.),(1.,
1.),(1.,1.),(1.,1.),(1.,1.),(1.,1.),(1.,1.),(1.,1.),(1.,1.),(1.,1.),(1.,
1.),(1.,1.),(1.,1.),(1.,1.),(1.,1.),(1.,1.),(1.,1.),(1.,1.),(1.,1.),(1.,
1.),(1.,1.),(1.,1.),(1.,1.),(1.,1.),(1.,1.),(1.,1.),(1.,1.),(1.,1.),(1.,
1.),(1.,1.),(1.,1.),(1.,1.),(1.,1.),(1.,1.),(1.,1.),(1.,1.),(1.,1.),(1.,
1.),(1.,1.),(1.,1.),(1.,1.),(1.,1.),(1.,1.),(1.,1.),(1.,1.),(1.,1.),(1.,
1.),(1.,1.),(1.,1.),(1.,1.),(1.,1.),(1.,1.),(1.,1.),(1.,1.),(1.,1.),(1.,
1.),(1.,1.),(1.,1.),(1.,1.),(1.,1.),(1.,1.),(1.,1.),(1.,1.),(1.,1.),(1.,
1.),(1.,1.)))
REPRESENTATION_ITEM('')
SURFACE()
);
#20=(
BOUNDED_SURFACE()
B_SPLINE_SURFACE(5,1,((#27724,#27725),(#27726,#27727),(#27728,#27729),(#27730,
#27731),(#27732,#27733),(#27734,#27735),(#27736,#27737),(#27738,#27739),
(#27740,#27741),(#27742,#27743),(#27744,#27745),(#27746,#27747),(#27748,
#27749),(#27750,#27751),(#27752,#27753),(#27754,#27755),(#27756,#27757),
(#27758,#27759),(#27760,#27761),(#27762,#27763),(#27764,#27765),(#27766,
#27767),(#27768,#27769),(#27770,#27771),(#27772,#27773),(#27774,#27775),
(#27776,#27777),(#27778,#27779),(#27780,#27781),(#27782,#27783),(#27784,
#27785),(#27786,#27787),(#27788,#27789),(#27790,#27791),(#27792,#27793),
(#27794,#27795),(#27796,#27797),(#27798,#27799),(#27800,#27801),(#27802,
#27803),(#27804,#27805),(#27806,#27807),(#27808,#27809),(#27810,#27811),
(#27812,#27813),(#27814,#27815),(#27816,#27817),(#27818,#27819),(#27820,
#27821),(#27822,#27823),(#27824,#27825),(#27826,#27827),(#27828,#27829),
(#27830,#27831),(#27832,#27833),(#27834,#27835),(#27836,#27837),(#27838,
#27839),(#27840,#27841),(#27842,#27843),(#27844,#27845),(#27846,#27847),
(#27848,#27849),(#27850,#27851),(#27852,#27853),(#27854,#27855),(#27856,
#27857),(#27858,#27859),(#27860,#27861),(#27862,#27863)),.UNSPECIFIED.,
 .F.,.F.,.F.)
B_SPLINE_SURFACE_WITH_KNOTS((6,1,1,1,1,1,1,1,1,1,1,1,1,1,1,1,1,1,1,1,1,
1,1,1,1,1,1,1,1,1,1,1,1,1,1,1,1,1,1,1,1,1,1,1,1,1,1,1,1,1,1,1,1,1,1,1,1,
1,1,1,1,1,1,1,1,6),(2,2),(-1.,-0.984615384615383,-0.969230769230768,-0.953846153846152,
-0.938461538461537,-0.923076923076922,-0.907692307692306,-0.892307692307691,
-0.876923076923076,-0.86153846153846,-0.846153846153845,-0.83076923076923,
-0.815384615384614,-0.799999999999999,-0.784615384615384,-0.769230769230768,
-0.753846153846153,-0.738461538461538,-0.723076923076922,-0.707692307692307,
-0.692307692307692,-0.676923076923076,-0.661538461538461,-0.646153846153846,
-0.63076923076923,-0.615384615384615,-0.6,-0.584615384615384,-0.569230769230769,
-0.553846153846154,-0.538461538461538,-0.523076923076923,-0.507692307692308,
-0.492307692307692,-0.476923076923077,-0.461538461538462,-0.446153846153846,
-0.430769230769231,-0.415384615384615,-0.4,-0.384615384615385,-0.369230769230769,
-0.353846153846154,-0.338461538461538,-0.323076923076923,-0.307692307692308,
-0.292307692307692,-0.276923076923077,-0.261538461538462,-0.246153846153846,
-0.230769230769231,-0.215384615384615,-0.2,-0.184615384615385,-0.169230769230769,
-0.153846153846154,-0.138461538461538,-0.123076923076923,-0.107692307692308,
-0.0923076923076923,-0.0769230769230769,-0.0615384615384615,-0.0461538461538462,
-0.0307692307692308,-0.0153846153846154,0.),(-1.,1.),.UNSPECIFIED.)
GEOMETRIC_REPRESENTATION_ITEM()
RATIONAL_B_SPLINE_SURFACE(((1.,1.),(1.,1.),(1.,1.),(1.,1.),(1.,1.),(1.,
1.),(1.,1.),(1.,1.),(1.,1.),(1.,1.),(1.,1.),(1.,1.),(1.,1.),(1.,1.),(1.,
1.),(1.,1.),(1.,1.),(1.,1.),(1.,1.),(1.,1.),(1.,1.),(1.,1.),(1.,1.),(1.,
1.),(1.,1.),(1.,1.),(1.,1.),(1.,1.),(1.,1.),(1.,1.),(1.,1.),(1.,1.),(1.,
1.),(1.,1.),(1.,1.),(1.,1.),(1.,1.),(1.,1.),(1.,1.),(1.,1.),(1.,1.),(1.,
1.),(1.,1.),(1.,1.),(1.,1.),(1.,1.),(1.,1.),(1.,1.),(1.,1.),(1.,1.),(1.,
1.),(1.,1.),(1.,1.),(1.,1.),(1.,1.),(1.,1.),(1.,1.),(1.,1.),(1.,1.),(1.,
1.),(1.,1.),(1.,1.),(1.,1.),(1.,1.),(1.,1.),(1.,1.),(1.,1.),(1.,1.),(1.,
1.),(1.,1.)))
REPRESENTATION_ITEM('')
SURFACE()
);
#21=(
BOUNDED_SURFACE()
B_SPLINE_SURFACE(5,1,((#27940,#27941),(#27942,#27943),(#27944,#27945),(#27946,
#27947),(#27948,#27949),(#27950,#27951),(#27952,#27953),(#27954,#27955),
(#27956,#27957),(#27958,#27959),(#27960,#27961),(#27962,#27963),(#27964,
#27965),(#27966,#27967),(#27968,#27969),(#27970,#27971),(#27972,#27973),
(#27974,#27975),(#27976,#27977),(#27978,#27979),(#27980,#27981),(#27982,
#27983),(#27984,#27985),(#27986,#27987),(#27988,#27989),(#27990,#27991),
(#27992,#27993),(#27994,#27995),(#27996,#27997),(#27998,#27999),(#28000,
#28001),(#28002,#28003),(#28004,#28005),(#28006,#28007),(#28008,#28009),
(#28010,#28011),(#28012,#28013),(#28014,#28015),(#28016,#28017),(#28018,
#28019),(#28020,#28021),(#28022,#28023),(#28024,#28025),(#28026,#28027),
(#28028,#28029),(#28030,#28031),(#28032,#28033),(#28034,#28035),(#28036,
#28037),(#28038,#28039),(#28040,#28041),(#28042,#28043),(#28044,#28045),
(#28046,#28047),(#28048,#28049),(#28050,#28051),(#28052,#28053),(#28054,
#28055),(#28056,#28057),(#28058,#28059),(#28060,#28061),(#28062,#28063),
(#28064,#28065),(#28066,#28067),(#28068,#28069),(#28070,#28071),(#28072,
#28073),(#28074,#28075),(#28076,#28077),(#28078,#28079)),.UNSPECIFIED.,
 .F.,.F.,.F.)
B_SPLINE_SURFACE_WITH_KNOTS((6,1,1,1,1,1,1,1,1,1,1,1,1,1,1,1,1,1,1,1,1,
1,1,1,1,1,1,1,1,1,1,1,1,1,1,1,1,1,1,1,1,1,1,1,1,1,1,1,1,1,1,1,1,1,1,1,1,
1,1,1,1,1,1,1,1,6),(2,2),(-1.,-0.984615384615383,-0.969230769230768,-0.953846153846152,
-0.938461538461537,-0.923076923076922,-0.907692307692306,-0.892307692307691,
-0.876923076923076,-0.86153846153846,-0.846153846153845,-0.83076923076923,
-0.815384615384614,-0.799999999999999,-0.784615384615384,-0.769230769230768,
-0.753846153846153,-0.738461538461538,-0.723076923076922,-0.707692307692307,
-0.692307692307692,-0.676923076923076,-0.661538461538461,-0.646153846153846,
-0.63076923076923,-0.615384615384615,-0.6,-0.584615384615384,-0.569230769230769,
-0.553846153846154,-0.538461538461538,-0.523076923076923,-0.507692307692308,
-0.492307692307692,-0.476923076923077,-0.461538461538462,-0.446153846153846,
-0.430769230769231,-0.415384615384615,-0.4,-0.384615384615385,-0.369230769230769,
-0.353846153846154,-0.338461538461538,-0.323076923076923,-0.307692307692308,
-0.292307692307692,-0.276923076923077,-0.261538461538462,-0.246153846153846,
-0.230769230769231,-0.215384615384615,-0.2,-0.184615384615385,-0.169230769230769,
-0.153846153846154,-0.138461538461538,-0.123076923076923,-0.107692307692308,
-0.0923076923076923,-0.0769230769230769,-0.0615384615384615,-0.0461538461538462,
-0.0307692307692308,-0.0153846153846154,0.),(-1.,1.),.UNSPECIFIED.)
GEOMETRIC_REPRESENTATION_ITEM()
RATIONAL_B_SPLINE_SURFACE(((1.,1.),(1.,1.),(1.,1.),(1.,1.),(1.,1.),(1.,
1.),(1.,1.),(1.,1.),(1.,1.),(1.,1.),(1.,1.),(1.,1.),(1.,1.),(1.,1.),(1.,
1.),(1.,1.),(1.,1.),(1.,1.),(1.,1.),(1.,1.),(1.,1.),(1.,1.),(1.,1.),(1.,
1.),(1.,1.),(1.,1.),(1.,1.),(1.,1.),(1.,1.),(1.,1.),(1.,1.),(1.,1.),(1.,
1.),(1.,1.),(1.,1.),(1.,1.),(1.,1.),(1.,1.),(1.,1.),(1.,1.),(1.,1.),(1.,
1.),(1.,1.),(1.,1.),(1.,1.),(1.,1.),(1.,1.),(1.,1.),(1.,1.),(1.,1.),(1.,
1.),(1.,1.),(1.,1.),(1.,1.),(1.,1.),(1.,1.),(1.,1.),(1.,1.),(1.,1.),(1.,
1.),(1.,1.),(1.,1.),(1.,1.),(1.,1.),(1.,1.),(1.,1.),(1.,1.),(1.,1.),(1.,
1.),(1.,1.)))
REPRESENTATION_ITEM('')
SURFACE()
);
#22=(
BOUNDED_SURFACE()
B_SPLINE_SURFACE(5,1,((#28156,#28157),(#28158,#28159),(#28160,#28161),(#28162,
#28163),(#28164,#28165),(#28166,#28167),(#28168,#28169),(#28170,#28171),
(#28172,#28173),(#28174,#28175),(#28176,#28177),(#28178,#28179),(#28180,
#28181),(#28182,#28183),(#28184,#28185),(#28186,#28187),(#28188,#28189),
(#28190,#28191),(#28192,#28193),(#28194,#28195),(#28196,#28197),(#28198,
#28199),(#28200,#28201),(#28202,#28203),(#28204,#28205),(#28206,#28207),
(#28208,#28209),(#28210,#28211),(#28212,#28213),(#28214,#28215),(#28216,
#28217),(#28218,#28219),(#28220,#28221),(#28222,#28223),(#28224,#28225),
(#28226,#28227),(#28228,#28229),(#28230,#28231),(#28232,#28233),(#28234,
#28235),(#28236,#28237),(#28238,#28239),(#28240,#28241),(#28242,#28243),
(#28244,#28245),(#28246,#28247),(#28248,#28249),(#28250,#28251),(#28252,
#28253),(#28254,#28255),(#28256,#28257),(#28258,#28259),(#28260,#28261),
(#28262,#28263),(#28264,#28265),(#28266,#28267),(#28268,#28269),(#28270,
#28271),(#28272,#28273),(#28274,#28275),(#28276,#28277),(#28278,#28279),
(#28280,#28281),(#28282,#28283),(#28284,#28285),(#28286,#28287),(#28288,
#28289),(#28290,#28291),(#28292,#28293),(#28294,#28295)),.UNSPECIFIED.,
 .F.,.F.,.F.)
B_SPLINE_SURFACE_WITH_KNOTS((6,1,1,1,1,1,1,1,1,1,1,1,1,1,1,1,1,1,1,1,1,
1,1,1,1,1,1,1,1,1,1,1,1,1,1,1,1,1,1,1,1,1,1,1,1,1,1,1,1,1,1,1,1,1,1,1,1,
1,1,1,1,1,1,1,1,6),(2,2),(-1.,-0.984615384615383,-0.969230769230768,-0.953846153846152,
-0.938461538461537,-0.923076923076922,-0.907692307692306,-0.892307692307691,
-0.876923076923076,-0.86153846153846,-0.846153846153845,-0.83076923076923,
-0.815384615384614,-0.799999999999999,-0.784615384615384,-0.769230769230768,
-0.753846153846153,-0.738461538461538,-0.723076923076922,-0.707692307692307,
-0.692307692307692,-0.676923076923076,-0.661538461538461,-0.646153846153846,
-0.63076923076923,-0.615384615384615,-0.6,-0.584615384615384,-0.569230769230769,
-0.553846153846154,-0.538461538461538,-0.523076923076923,-0.507692307692308,
-0.492307692307692,-0.476923076923077,-0.461538461538462,-0.446153846153846,
-0.430769230769231,-0.415384615384615,-0.4,-0.384615384615385,-0.369230769230769,
-0.353846153846154,-0.338461538461538,-0.323076923076923,-0.307692307692308,
-0.292307692307692,-0.276923076923077,-0.261538461538462,-0.246153846153846,
-0.230769230769231,-0.215384615384615,-0.2,-0.184615384615385,-0.169230769230769,
-0.153846153846154,-0.138461538461538,-0.123076923076923,-0.107692307692308,
-0.0923076923076923,-0.0769230769230769,-0.0615384615384615,-0.0461538461538462,
-0.0307692307692308,-0.0153846153846154,0.),(-1.,1.),.UNSPECIFIED.)
GEOMETRIC_REPRESENTATION_ITEM()
RATIONAL_B_SPLINE_SURFACE(((1.,1.),(1.,1.),(1.,1.),(1.,1.),(1.,1.),(1.,
1.),(1.,1.),(1.,1.),(1.,1.),(1.,1.),(1.,1.),(1.,1.),(1.,1.),(1.,1.),(1.,
1.),(1.,1.),(1.,1.),(1.,1.),(1.,1.),(1.,1.),(1.,1.),(1.,1.),(1.,1.),(1.,
1.),(1.,1.),(1.,1.),(1.,1.),(1.,1.),(1.,1.),(1.,1.),(1.,1.),(1.,1.),(1.,
1.),(1.,1.),(1.,1.),(1.,1.),(1.,1.),(1.,1.),(1.,1.),(1.,1.),(1.,1.),(1.,
1.),(1.,1.),(1.,1.),(1.,1.),(1.,1.),(1.,1.),(1.,1.),(1.,1.),(1.,1.),(1.,
1.),(1.,1.),(1.,1.),(1.,1.),(1.,1.),(1.,1.),(1.,1.),(1.,1.),(1.,1.),(1.,
1.),(1.,1.),(1.,1.),(1.,1.),(1.,1.),(1.,1.),(1.,1.),(1.,1.),(1.,1.),(1.,
1.),(1.,1.)))
REPRESENTATION_ITEM('')
SURFACE()
);
#23=(
BOUNDED_SURFACE()
B_SPLINE_SURFACE(5,1,((#28372,#28373),(#28374,#28375),(#28376,#28377),(#28378,
#28379),(#28380,#28381),(#28382,#28383),(#28384,#28385),(#28386,#28387),
(#28388,#28389),(#28390,#28391),(#28392,#28393),(#28394,#28395),(#28396,
#28397),(#28398,#28399),(#28400,#28401),(#28402,#28403),(#28404,#28405),
(#28406,#28407),(#28408,#28409),(#28410,#28411),(#28412,#28413),(#28414,
#28415),(#28416,#28417),(#28418,#28419),(#28420,#28421),(#28422,#28423),
(#28424,#28425),(#28426,#28427),(#28428,#28429),(#28430,#28431),(#28432,
#28433),(#28434,#28435),(#28436,#28437),(#28438,#28439),(#28440,#28441),
(#28442,#28443),(#28444,#28445),(#28446,#28447),(#28448,#28449),(#28450,
#28451),(#28452,#28453),(#28454,#28455),(#28456,#28457),(#28458,#28459),
(#28460,#28461),(#28462,#28463),(#28464,#28465),(#28466,#28467),(#28468,
#28469),(#28470,#28471),(#28472,#28473),(#28474,#28475),(#28476,#28477),
(#28478,#28479),(#28480,#28481),(#28482,#28483),(#28484,#28485),(#28486,
#28487),(#28488,#28489),(#28490,#28491),(#28492,#28493),(#28494,#28495),
(#28496,#28497),(#28498,#28499),(#28500,#28501),(#28502,#28503),(#28504,
#28505),(#28506,#28507),(#28508,#28509),(#28510,#28511)),.UNSPECIFIED.,
 .F.,.F.,.F.)
B_SPLINE_SURFACE_WITH_KNOTS((6,1,1,1,1,1,1,1,1,1,1,1,1,1,1,1,1,1,1,1,1,
1,1,1,1,1,1,1,1,1,1,1,1,1,1,1,1,1,1,1,1,1,1,1,1,1,1,1,1,1,1,1,1,1,1,1,1,
1,1,1,1,1,1,1,1,6),(2,2),(-1.,-0.984615384615383,-0.969230769230768,-0.953846153846152,
-0.938461538461537,-0.923076923076922,-0.907692307692306,-0.892307692307691,
-0.876923076923076,-0.86153846153846,-0.846153846153845,-0.83076923076923,
-0.815384615384614,-0.799999999999999,-0.784615384615384,-0.769230769230768,
-0.753846153846153,-0.738461538461538,-0.723076923076922,-0.707692307692307,
-0.692307692307692,-0.676923076923076,-0.661538461538461,-0.646153846153846,
-0.63076923076923,-0.615384615384615,-0.6,-0.584615384615384,-0.569230769230769,
-0.553846153846154,-0.538461538461538,-0.523076923076923,-0.507692307692308,
-0.492307692307692,-0.476923076923077,-0.461538461538462,-0.446153846153846,
-0.430769230769231,-0.415384615384615,-0.4,-0.384615384615385,-0.369230769230769,
-0.353846153846154,-0.338461538461538,-0.323076923076923,-0.307692307692308,
-0.292307692307692,-0.276923076923077,-0.261538461538462,-0.246153846153846,
-0.230769230769231,-0.215384615384615,-0.2,-0.184615384615385,-0.169230769230769,
-0.153846153846154,-0.138461538461538,-0.123076923076923,-0.107692307692308,
-0.0923076923076923,-0.0769230769230769,-0.0615384615384615,-0.0461538461538462,
-0.0307692307692308,-0.0153846153846154,0.),(-1.,1.),.UNSPECIFIED.)
GEOMETRIC_REPRESENTATION_ITEM()
RATIONAL_B_SPLINE_SURFACE(((1.,1.),(1.,1.),(1.,1.),(1.,1.),(1.,1.),(1.,
1.),(1.,1.),(1.,1.),(1.,1.),(1.,1.),(1.,1.),(1.,1.),(1.,1.),(1.,1.),(1.,
1.),(1.,1.),(1.,1.),(1.,1.),(1.,1.),(1.,1.),(1.,1.),(1.,1.),(1.,1.),(1.,
1.),(1.,1.),(1.,1.),(1.,1.),(1.,1.),(1.,1.),(1.,1.),(1.,1.),(1.,1.),(1.,
1.),(1.,1.),(1.,1.),(1.,1.),(1.,1.),(1.,1.),(1.,1.),(1.,1.),(1.,1.),(1.,
1.),(1.,1.),(1.,1.),(1.,1.),(1.,1.),(1.,1.),(1.,1.),(1.,1.),(1.,1.),(1.,
1.),(1.,1.),(1.,1.),(1.,1.),(1.,1.),(1.,1.),(1.,1.),(1.,1.),(1.,1.),(1.,
1.),(1.,1.),(1.,1.),(1.,1.),(1.,1.),(1.,1.),(1.,1.),(1.,1.),(1.,1.),(1.,
1.),(1.,1.)))
REPRESENTATION_ITEM('')
SURFACE()
);
#24=(
BOUNDED_SURFACE()
B_SPLINE_SURFACE(5,1,((#28588,#28589),(#28590,#28591),(#28592,#28593),(#28594,
#28595),(#28596,#28597),(#28598,#28599),(#28600,#28601),(#28602,#28603),
(#28604,#28605),(#28606,#28607),(#28608,#28609),(#28610,#28611),(#28612,
#28613),(#28614,#28615),(#28616,#28617),(#28618,#28619),(#28620,#28621),
(#28622,#28623),(#28624,#28625),(#28626,#28627),(#28628,#28629),(#28630,
#28631),(#28632,#28633),(#28634,#28635),(#28636,#28637),(#28638,#28639),
(#28640,#28641),(#28642,#28643),(#28644,#28645),(#28646,#28647),(#28648,
#28649),(#28650,#28651),(#28652,#28653),(#28654,#28655),(#28656,#28657),
(#28658,#28659),(#28660,#28661),(#28662,#28663),(#28664,#28665),(#28666,
#28667),(#28668,#28669),(#28670,#28671),(#28672,#28673),(#28674,#28675),
(#28676,#28677),(#28678,#28679),(#28680,#28681),(#28682,#28683),(#28684,
#28685),(#28686,#28687),(#28688,#28689),(#28690,#28691),(#28692,#28693),
(#28694,#28695),(#28696,#28697),(#28698,#28699),(#28700,#28701),(#28702,
#28703),(#28704,#28705),(#28706,#28707),(#28708,#28709),(#28710,#28711),
(#28712,#28713),(#28714,#28715),(#28716,#28717),(#28718,#28719),(#28720,
#28721),(#28722,#28723),(#28724,#28725),(#28726,#28727)),.UNSPECIFIED.,
 .F.,.F.,.F.)
B_SPLINE_SURFACE_WITH_KNOTS((6,1,1,1,1,1,1,1,1,1,1,1,1,1,1,1,1,1,1,1,1,
1,1,1,1,1,1,1,1,1,1,1,1,1,1,1,1,1,1,1,1,1,1,1,1,1,1,1,1,1,1,1,1,1,1,1,1,
1,1,1,1,1,1,1,1,6),(2,2),(-1.,-0.984615384615383,-0.969230769230768,-0.953846153846152,
-0.938461538461537,-0.923076923076922,-0.907692307692306,-0.892307692307691,
-0.876923076923076,-0.86153846153846,-0.846153846153845,-0.83076923076923,
-0.815384615384614,-0.799999999999999,-0.784615384615384,-0.769230769230768,
-0.753846153846153,-0.738461538461538,-0.723076923076922,-0.707692307692307,
-0.692307692307692,-0.676923076923076,-0.661538461538461,-0.646153846153846,
-0.63076923076923,-0.615384615384615,-0.6,-0.584615384615384,-0.569230769230769,
-0.553846153846154,-0.538461538461538,-0.523076923076923,-0.507692307692308,
-0.492307692307692,-0.476923076923077,-0.461538461538462,-0.446153846153846,
-0.430769230769231,-0.415384615384615,-0.4,-0.384615384615385,-0.369230769230769,
-0.353846153846154,-0.338461538461538,-0.323076923076923,-0.307692307692308,
-0.292307692307692,-0.276923076923077,-0.261538461538462,-0.246153846153846,
-0.230769230769231,-0.215384615384615,-0.2,-0.184615384615385,-0.169230769230769,
-0.153846153846154,-0.138461538461538,-0.123076923076923,-0.107692307692308,
-0.0923076923076923,-0.0769230769230769,-0.0615384615384615,-0.0461538461538462,
-0.0307692307692308,-0.0153846153846154,0.),(-1.,1.),.UNSPECIFIED.)
GEOMETRIC_REPRESENTATION_ITEM()
RATIONAL_B_SPLINE_SURFACE(((1.,1.),(1.,1.),(1.,1.),(1.,1.),(1.,1.),(1.,
1.),(1.,1.),(1.,1.),(1.,1.),(1.,1.),(1.,1.),(1.,1.),(1.,1.),(1.,1.),(1.,
1.),(1.,1.),(1.,1.),(1.,1.),(1.,1.),(1.,1.),(1.,1.),(1.,1.),(1.,1.),(1.,
1.),(1.,1.),(1.,1.),(1.,1.),(1.,1.),(1.,1.),(1.,1.),(1.,1.),(1.,1.),(1.,
1.),(1.,1.),(1.,1.),(1.,1.),(1.,1.),(1.,1.),(1.,1.),(1.,1.),(1.,1.),(1.,
1.),(1.,1.),(1.,1.),(1.,1.),(1.,1.),(1.,1.),(1.,1.),(1.,1.),(1.,1.),(1.,
1.),(1.,1.),(1.,1.),(1.,1.),(1.,1.),(1.,1.),(1.,1.),(1.,1.),(1.,1.),(1.,
1.),(1.,1.),(1.,1.),(1.,1.),(1.,1.),(1.,1.),(1.,1.),(1.,1.),(1.,1.),(1.,
1.),(1.,1.)))
REPRESENTATION_ITEM('')
SURFACE()
);
#25=(
BOUNDED_SURFACE()
B_SPLINE_SURFACE(5,1,((#28804,#28805),(#28806,#28807),(#28808,#28809),(#28810,
#28811),(#28812,#28813),(#28814,#28815),(#28816,#28817),(#28818,#28819),
(#28820,#28821),(#28822,#28823),(#28824,#28825),(#28826,#28827),(#28828,
#28829),(#28830,#28831),(#28832,#28833),(#28834,#28835),(#28836,#28837),
(#28838,#28839),(#28840,#28841),(#28842,#28843),(#28844,#28845),(#28846,
#28847),(#28848,#28849),(#28850,#28851),(#28852,#28853),(#28854,#28855),
(#28856,#28857),(#28858,#28859),(#28860,#28861),(#28862,#28863),(#28864,
#28865),(#28866,#28867),(#28868,#28869),(#28870,#28871),(#28872,#28873),
(#28874,#28875),(#28876,#28877),(#28878,#28879),(#28880,#28881),(#28882,
#28883),(#28884,#28885),(#28886,#28887),(#28888,#28889),(#28890,#28891),
(#28892,#28893),(#28894,#28895),(#28896,#28897),(#28898,#28899),(#28900,
#28901),(#28902,#28903),(#28904,#28905),(#28906,#28907),(#28908,#28909),
(#28910,#28911),(#28912,#28913),(#28914,#28915),(#28916,#28917),(#28918,
#28919),(#28920,#28921),(#28922,#28923),(#28924,#28925),(#28926,#28927),
(#28928,#28929),(#28930,#28931),(#28932,#28933),(#28934,#28935),(#28936,
#28937),(#28938,#28939),(#28940,#28941),(#28942,#28943)),.UNSPECIFIED.,
 .F.,.F.,.F.)
B_SPLINE_SURFACE_WITH_KNOTS((6,1,1,1,1,1,1,1,1,1,1,1,1,1,1,1,1,1,1,1,1,
1,1,1,1,1,1,1,1,1,1,1,1,1,1,1,1,1,1,1,1,1,1,1,1,1,1,1,1,1,1,1,1,1,1,1,1,
1,1,1,1,1,1,1,1,6),(2,2),(-1.,-0.984615384615383,-0.969230769230768,-0.953846153846152,
-0.938461538461537,-0.923076923076922,-0.907692307692306,-0.892307692307691,
-0.876923076923076,-0.86153846153846,-0.846153846153845,-0.83076923076923,
-0.815384615384614,-0.799999999999999,-0.784615384615384,-0.769230769230768,
-0.753846153846153,-0.738461538461538,-0.723076923076922,-0.707692307692307,
-0.692307692307692,-0.676923076923076,-0.661538461538461,-0.646153846153846,
-0.63076923076923,-0.615384615384615,-0.6,-0.584615384615384,-0.569230769230769,
-0.553846153846154,-0.538461538461538,-0.523076923076923,-0.507692307692308,
-0.492307692307692,-0.476923076923077,-0.461538461538462,-0.446153846153846,
-0.430769230769231,-0.415384615384615,-0.4,-0.384615384615385,-0.369230769230769,
-0.353846153846154,-0.338461538461538,-0.323076923076923,-0.307692307692308,
-0.292307692307692,-0.276923076923077,-0.261538461538462,-0.246153846153846,
-0.230769230769231,-0.215384615384615,-0.2,-0.184615384615385,-0.169230769230769,
-0.153846153846154,-0.138461538461538,-0.123076923076923,-0.107692307692308,
-0.0923076923076923,-0.0769230769230769,-0.0615384615384615,-0.0461538461538462,
-0.0307692307692308,-0.0153846153846154,0.),(-1.,1.),.UNSPECIFIED.)
GEOMETRIC_REPRESENTATION_ITEM()
RATIONAL_B_SPLINE_SURFACE(((1.,1.),(1.,1.),(1.,1.),(1.,1.),(1.,1.),(1.,
1.),(1.,1.),(1.,1.),(1.,1.),(1.,1.),(1.,1.),(1.,1.),(1.,1.),(1.,1.),(1.,
1.),(1.,1.),(1.,1.),(1.,1.),(1.,1.),(1.,1.),(1.,1.),(1.,1.),(1.,1.),(1.,
1.),(1.,1.),(1.,1.),(1.,1.),(1.,1.),(1.,1.),(1.,1.),(1.,1.),(1.,1.),(1.,
1.),(1.,1.),(1.,1.),(1.,1.),(1.,1.),(1.,1.),(1.,1.),(1.,1.),(1.,1.),(1.,
1.),(1.,1.),(1.,1.),(1.,1.),(1.,1.),(1.,1.),(1.,1.),(1.,1.),(1.,1.),(1.,
1.),(1.,1.),(1.,1.),(1.,1.),(1.,1.),(1.,1.),(1.,1.),(1.,1.),(1.,1.),(1.,
1.),(1.,1.),(1.,1.),(1.,1.),(1.,1.),(1.,1.),(1.,1.),(1.,1.),(1.,1.),(1.,
1.),(1.,1.)))
REPRESENTATION_ITEM('')
SURFACE()
);
#26=(
BOUNDED_SURFACE()
B_SPLINE_SURFACE(5,1,((#29020,#29021),(#29022,#29023),(#29024,#29025),(#29026,
#29027),(#29028,#29029),(#29030,#29031),(#29032,#29033),(#29034,#29035),
(#29036,#29037),(#29038,#29039),(#29040,#29041),(#29042,#29043),(#29044,
#29045),(#29046,#29047),(#29048,#29049),(#29050,#29051),(#29052,#29053),
(#29054,#29055),(#29056,#29057),(#29058,#29059),(#29060,#29061),(#29062,
#29063),(#29064,#29065),(#29066,#29067),(#29068,#29069),(#29070,#29071),
(#29072,#29073),(#29074,#29075),(#29076,#29077),(#29078,#29079),(#29080,
#29081),(#29082,#29083),(#29084,#29085),(#29086,#29087),(#29088,#29089),
(#29090,#29091),(#29092,#29093),(#29094,#29095),(#29096,#29097),(#29098,
#29099),(#29100,#29101),(#29102,#29103),(#29104,#29105),(#29106,#29107),
(#29108,#29109),(#29110,#29111),(#29112,#29113),(#29114,#29115),(#29116,
#29117),(#29118,#29119),(#29120,#29121),(#29122,#29123),(#29124,#29125),
(#29126,#29127),(#29128,#29129),(#29130,#29131),(#29132,#29133),(#29134,
#29135),(#29136,#29137),(#29138,#29139),(#29140,#29141),(#29142,#29143),
(#29144,#29145),(#29146,#29147),(#29148,#29149),(#29150,#29151),(#29152,
#29153),(#29154,#29155),(#29156,#29157),(#29158,#29159)),.UNSPECIFIED.,
 .F.,.F.,.F.)
B_SPLINE_SURFACE_WITH_KNOTS((6,1,1,1,1,1,1,1,1,1,1,1,1,1,1,1,1,1,1,1,1,
1,1,1,1,1,1,1,1,1,1,1,1,1,1,1,1,1,1,1,1,1,1,1,1,1,1,1,1,1,1,1,1,1,1,1,1,
1,1,1,1,1,1,1,1,6),(2,2),(-1.,-0.984615384615383,-0.969230769230768,-0.953846153846152,
-0.938461538461537,-0.923076923076922,-0.907692307692306,-0.892307692307691,
-0.876923076923076,-0.86153846153846,-0.846153846153845,-0.83076923076923,
-0.815384615384614,-0.799999999999999,-0.784615384615384,-0.769230769230768,
-0.753846153846153,-0.738461538461538,-0.723076923076922,-0.707692307692307,
-0.692307692307692,-0.676923076923076,-0.661538461538461,-0.646153846153846,
-0.63076923076923,-0.615384615384615,-0.6,-0.584615384615384,-0.569230769230769,
-0.553846153846154,-0.538461538461538,-0.523076923076923,-0.507692307692308,
-0.492307692307692,-0.476923076923077,-0.461538461538462,-0.446153846153846,
-0.430769230769231,-0.415384615384615,-0.4,-0.384615384615385,-0.369230769230769,
-0.353846153846154,-0.338461538461538,-0.323076923076923,-0.307692307692308,
-0.292307692307692,-0.276923076923077,-0.261538461538462,-0.246153846153846,
-0.230769230769231,-0.215384615384615,-0.2,-0.184615384615385,-0.169230769230769,
-0.153846153846154,-0.138461538461538,-0.123076923076923,-0.107692307692308,
-0.0923076923076923,-0.0769230769230769,-0.0615384615384615,-0.0461538461538462,
-0.0307692307692308,-0.0153846153846154,0.),(-1.,1.),.UNSPECIFIED.)
GEOMETRIC_REPRESENTATION_ITEM()
RATIONAL_B_SPLINE_SURFACE(((1.,1.),(1.,1.),(1.,1.),(1.,1.),(1.,1.),(1.,
1.),(1.,1.),(1.,1.),(1.,1.),(1.,1.),(1.,1.),(1.,1.),(1.,1.),(1.,1.),(1.,
1.),(1.,1.),(1.,1.),(1.,1.),(1.,1.),(1.,1.),(1.,1.),(1.,1.),(1.,1.),(1.,
1.),(1.,1.),(1.,1.),(1.,1.),(1.,1.),(1.,1.),(1.,1.),(1.,1.),(1.,1.),(1.,
1.),(1.,1.),(1.,1.),(1.,1.),(1.,1.),(1.,1.),(1.,1.),(1.,1.),(1.,1.),(1.,
1.),(1.,1.),(1.,1.),(1.,1.),(1.,1.),(1.,1.),(1.,1.),(1.,1.),(1.,1.),(1.,
1.),(1.,1.),(1.,1.),(1.,1.),(1.,1.),(1.,1.),(1.,1.),(1.,1.),(1.,1.),(1.,
1.),(1.,1.),(1.,1.),(1.,1.),(1.,1.),(1.,1.),(1.,1.),(1.,1.),(1.,1.),(1.,
1.),(1.,1.)))
REPRESENTATION_ITEM('')
SURFACE()
);
#27=(
BOUNDED_SURFACE()
B_SPLINE_SURFACE(5,1,((#29236,#29237),(#29238,#29239),(#29240,#29241),(#29242,
#29243),(#29244,#29245),(#29246,#29247),(#29248,#29249),(#29250,#29251),
(#29252,#29253),(#29254,#29255),(#29256,#29257),(#29258,#29259),(#29260,
#29261),(#29262,#29263),(#29264,#29265),(#29266,#29267),(#29268,#29269),
(#29270,#29271),(#29272,#29273),(#29274,#29275),(#29276,#29277),(#29278,
#29279),(#29280,#29281),(#29282,#29283),(#29284,#29285),(#29286,#29287),
(#29288,#29289),(#29290,#29291),(#29292,#29293),(#29294,#29295),(#29296,
#29297),(#29298,#29299),(#29300,#29301),(#29302,#29303),(#29304,#29305),
(#29306,#29307),(#29308,#29309),(#29310,#29311),(#29312,#29313),(#29314,
#29315),(#29316,#29317),(#29318,#29319),(#29320,#29321),(#29322,#29323),
(#29324,#29325),(#29326,#29327),(#29328,#29329),(#29330,#29331),(#29332,
#29333),(#29334,#29335),(#29336,#29337),(#29338,#29339),(#29340,#29341),
(#29342,#29343),(#29344,#29345),(#29346,#29347),(#29348,#29349),(#29350,
#29351),(#29352,#29353),(#29354,#29355),(#29356,#29357),(#29358,#29359),
(#29360,#29361),(#29362,#29363),(#29364,#29365),(#29366,#29367),(#29368,
#29369),(#29370,#29371),(#29372,#29373),(#29374,#29375)),.UNSPECIFIED.,
 .F.,.F.,.F.)
B_SPLINE_SURFACE_WITH_KNOTS((6,1,1,1,1,1,1,1,1,1,1,1,1,1,1,1,1,1,1,1,1,
1,1,1,1,1,1,1,1,1,1,1,1,1,1,1,1,1,1,1,1,1,1,1,1,1,1,1,1,1,1,1,1,1,1,1,1,
1,1,1,1,1,1,1,1,6),(2,2),(-1.,-0.984615384615383,-0.969230769230768,-0.953846153846152,
-0.938461538461537,-0.923076923076922,-0.907692307692306,-0.892307692307691,
-0.876923076923076,-0.86153846153846,-0.846153846153845,-0.83076923076923,
-0.815384615384614,-0.799999999999999,-0.784615384615384,-0.769230769230768,
-0.753846153846153,-0.738461538461538,-0.723076923076922,-0.707692307692307,
-0.692307692307692,-0.676923076923076,-0.661538461538461,-0.646153846153846,
-0.63076923076923,-0.615384615384615,-0.6,-0.584615384615384,-0.569230769230769,
-0.553846153846154,-0.538461538461538,-0.523076923076923,-0.507692307692308,
-0.492307692307692,-0.476923076923077,-0.461538461538462,-0.446153846153846,
-0.430769230769231,-0.415384615384615,-0.4,-0.384615384615385,-0.369230769230769,
-0.353846153846154,-0.338461538461538,-0.323076923076923,-0.307692307692308,
-0.292307692307692,-0.276923076923077,-0.261538461538462,-0.246153846153846,
-0.230769230769231,-0.215384615384615,-0.2,-0.184615384615385,-0.169230769230769,
-0.153846153846154,-0.138461538461538,-0.123076923076923,-0.107692307692308,
-0.0923076923076923,-0.0769230769230769,-0.0615384615384615,-0.0461538461538462,
-0.0307692307692308,-0.0153846153846154,0.),(-1.,1.),.UNSPECIFIED.)
GEOMETRIC_REPRESENTATION_ITEM()
RATIONAL_B_SPLINE_SURFACE(((1.,1.),(1.,1.),(1.,1.),(1.,1.),(1.,1.),(1.,
1.),(1.,1.),(1.,1.),(1.,1.),(1.,1.),(1.,1.),(1.,1.),(1.,1.),(1.,1.),(1.,
1.),(1.,1.),(1.,1.),(1.,1.),(1.,1.),(1.,1.),(1.,1.),(1.,1.),(1.,1.),(1.,
1.),(1.,1.),(1.,1.),(1.,1.),(1.,1.),(1.,1.),(1.,1.),(1.,1.),(1.,1.),(1.,
1.),(1.,1.),(1.,1.),(1.,1.),(1.,1.),(1.,1.),(1.,1.),(1.,1.),(1.,1.),(1.,
1.),(1.,1.),(1.,1.),(1.,1.),(1.,1.),(1.,1.),(1.,1.),(1.,1.),(1.,1.),(1.,
1.),(1.,1.),(1.,1.),(1.,1.),(1.,1.),(1.,1.),(1.,1.),(1.,1.),(1.,1.),(1.,
1.),(1.,1.),(1.,1.),(1.,1.),(1.,1.),(1.,1.),(1.,1.),(1.,1.),(1.,1.),(1.,
1.),(1.,1.)))
REPRESENTATION_ITEM('')
SURFACE()
);
#28=(
BOUNDED_SURFACE()
B_SPLINE_SURFACE(5,1,((#29452,#29453),(#29454,#29455),(#29456,#29457),(#29458,
#29459),(#29460,#29461),(#29462,#29463),(#29464,#29465),(#29466,#29467),
(#29468,#29469),(#29470,#29471),(#29472,#29473),(#29474,#29475),(#29476,
#29477),(#29478,#29479),(#29480,#29481),(#29482,#29483),(#29484,#29485),
(#29486,#29487),(#29488,#29489),(#29490,#29491),(#29492,#29493),(#29494,
#29495),(#29496,#29497),(#29498,#29499),(#29500,#29501),(#29502,#29503),
(#29504,#29505),(#29506,#29507),(#29508,#29509),(#29510,#29511),(#29512,
#29513),(#29514,#29515),(#29516,#29517),(#29518,#29519),(#29520,#29521),
(#29522,#29523),(#29524,#29525),(#29526,#29527),(#29528,#29529),(#29530,
#29531),(#29532,#29533),(#29534,#29535),(#29536,#29537),(#29538,#29539),
(#29540,#29541),(#29542,#29543),(#29544,#29545),(#29546,#29547),(#29548,
#29549),(#29550,#29551),(#29552,#29553),(#29554,#29555),(#29556,#29557),
(#29558,#29559),(#29560,#29561),(#29562,#29563),(#29564,#29565),(#29566,
#29567),(#29568,#29569),(#29570,#29571),(#29572,#29573),(#29574,#29575),
(#29576,#29577),(#29578,#29579),(#29580,#29581),(#29582,#29583),(#29584,
#29585),(#29586,#29587),(#29588,#29589),(#29590,#29591)),.UNSPECIFIED.,
 .F.,.F.,.F.)
B_SPLINE_SURFACE_WITH_KNOTS((6,1,1,1,1,1,1,1,1,1,1,1,1,1,1,1,1,1,1,1,1,
1,1,1,1,1,1,1,1,1,1,1,1,1,1,1,1,1,1,1,1,1,1,1,1,1,1,1,1,1,1,1,1,1,1,1,1,
1,1,1,1,1,1,1,1,6),(2,2),(-1.,-0.984615384615383,-0.969230769230768,-0.953846153846152,
-0.938461538461537,-0.923076923076922,-0.907692307692306,-0.892307692307691,
-0.876923076923076,-0.86153846153846,-0.846153846153845,-0.83076923076923,
-0.815384615384614,-0.799999999999999,-0.784615384615384,-0.769230769230768,
-0.753846153846153,-0.738461538461538,-0.723076923076922,-0.707692307692307,
-0.692307692307692,-0.676923076923076,-0.661538461538461,-0.646153846153846,
-0.63076923076923,-0.615384615384615,-0.6,-0.584615384615384,-0.569230769230769,
-0.553846153846154,-0.538461538461538,-0.523076923076923,-0.507692307692308,
-0.492307692307692,-0.476923076923077,-0.461538461538462,-0.446153846153846,
-0.430769230769231,-0.415384615384615,-0.4,-0.384615384615385,-0.369230769230769,
-0.353846153846154,-0.338461538461538,-0.323076923076923,-0.307692307692308,
-0.292307692307692,-0.276923076923077,-0.261538461538462,-0.246153846153846,
-0.230769230769231,-0.215384615384615,-0.2,-0.184615384615385,-0.169230769230769,
-0.153846153846154,-0.138461538461538,-0.123076923076923,-0.107692307692308,
-0.0923076923076923,-0.0769230769230769,-0.0615384615384615,-0.0461538461538462,
-0.0307692307692308,-0.0153846153846154,0.),(-1.,1.),.UNSPECIFIED.)
GEOMETRIC_REPRESENTATION_ITEM()
RATIONAL_B_SPLINE_SURFACE(((1.,1.),(1.,1.),(1.,1.),(1.,1.),(1.,1.),(1.,
1.),(1.,1.),(1.,1.),(1.,1.),(1.,1.),(1.,1.),(1.,1.),(1.,1.),(1.,1.),(1.,
1.),(1.,1.),(1.,1.),(1.,1.),(1.,1.),(1.,1.),(1.,1.),(1.,1.),(1.,1.),(1.,
1.),(1.,1.),(1.,1.),(1.,1.),(1.,1.),(1.,1.),(1.,1.),(1.,1.),(1.,1.),(1.,
1.),(1.,1.),(1.,1.),(1.,1.),(1.,1.),(1.,1.),(1.,1.),(1.,1.),(1.,1.),(1.,
1.),(1.,1.),(1.,1.),(1.,1.),(1.,1.),(1.,1.),(1.,1.),(1.,1.),(1.,1.),(1.,
1.),(1.,1.),(1.,1.),(1.,1.),(1.,1.),(1.,1.),(1.,1.),(1.,1.),(1.,1.),(1.,
1.),(1.,1.),(1.,1.),(1.,1.),(1.,1.),(1.,1.),(1.,1.),(1.,1.),(1.,1.),(1.,
1.),(1.,1.)))
REPRESENTATION_ITEM('')
SURFACE()
);
#29=(
BOUNDED_SURFACE()
B_SPLINE_SURFACE(5,1,((#29668,#29669),(#29670,#29671),(#29672,#29673),(#29674,
#29675),(#29676,#29677),(#29678,#29679),(#29680,#29681),(#29682,#29683),
(#29684,#29685),(#29686,#29687),(#29688,#29689),(#29690,#29691),(#29692,
#29693),(#29694,#29695),(#29696,#29697),(#29698,#29699),(#29700,#29701),
(#29702,#29703),(#29704,#29705),(#29706,#29707),(#29708,#29709),(#29710,
#29711),(#29712,#29713),(#29714,#29715),(#29716,#29717),(#29718,#29719),
(#29720,#29721),(#29722,#29723),(#29724,#29725),(#29726,#29727),(#29728,
#29729),(#29730,#29731),(#29732,#29733),(#29734,#29735),(#29736,#29737),
(#29738,#29739),(#29740,#29741),(#29742,#29743),(#29744,#29745),(#29746,
#29747),(#29748,#29749),(#29750,#29751),(#29752,#29753),(#29754,#29755),
(#29756,#29757),(#29758,#29759),(#29760,#29761),(#29762,#29763),(#29764,
#29765),(#29766,#29767),(#29768,#29769),(#29770,#29771),(#29772,#29773),
(#29774,#29775),(#29776,#29777),(#29778,#29779),(#29780,#29781),(#29782,
#29783),(#29784,#29785),(#29786,#29787),(#29788,#29789),(#29790,#29791),
(#29792,#29793),(#29794,#29795),(#29796,#29797),(#29798,#29799),(#29800,
#29801),(#29802,#29803),(#29804,#29805),(#29806,#29807)),.UNSPECIFIED.,
 .F.,.F.,.F.)
B_SPLINE_SURFACE_WITH_KNOTS((6,1,1,1,1,1,1,1,1,1,1,1,1,1,1,1,1,1,1,1,1,
1,1,1,1,1,1,1,1,1,1,1,1,1,1,1,1,1,1,1,1,1,1,1,1,1,1,1,1,1,1,1,1,1,1,1,1,
1,1,1,1,1,1,1,1,6),(2,2),(-1.,-0.984615384615383,-0.969230769230768,-0.953846153846152,
-0.938461538461537,-0.923076923076922,-0.907692307692306,-0.892307692307691,
-0.876923076923076,-0.86153846153846,-0.846153846153845,-0.83076923076923,
-0.815384615384614,-0.799999999999999,-0.784615384615384,-0.769230769230768,
-0.753846153846153,-0.738461538461538,-0.723076923076922,-0.707692307692307,
-0.692307692307692,-0.676923076923076,-0.661538461538461,-0.646153846153846,
-0.63076923076923,-0.615384615384615,-0.6,-0.584615384615384,-0.569230769230769,
-0.553846153846154,-0.538461538461538,-0.523076923076923,-0.507692307692308,
-0.492307692307692,-0.476923076923077,-0.461538461538462,-0.446153846153846,
-0.430769230769231,-0.415384615384615,-0.4,-0.384615384615385,-0.369230769230769,
-0.353846153846154,-0.338461538461538,-0.323076923076923,-0.307692307692308,
-0.292307692307692,-0.276923076923077,-0.261538461538462,-0.246153846153846,
-0.230769230769231,-0.215384615384615,-0.2,-0.184615384615385,-0.169230769230769,
-0.153846153846154,-0.138461538461538,-0.123076923076923,-0.107692307692308,
-0.0923076923076923,-0.0769230769230769,-0.0615384615384615,-0.0461538461538462,
-0.0307692307692308,-0.0153846153846154,0.),(-1.,1.),.UNSPECIFIED.)
GEOMETRIC_REPRESENTATION_ITEM()
RATIONAL_B_SPLINE_SURFACE(((1.,1.),(1.,1.),(1.,1.),(1.,1.),(1.,1.),(1.,
1.),(1.,1.),(1.,1.),(1.,1.),(1.,1.),(1.,1.),(1.,1.),(1.,1.),(1.,1.),(1.,
1.),(1.,1.),(1.,1.),(1.,1.),(1.,1.),(1.,1.),(1.,1.),(1.,1.),(1.,1.),(1.,
1.),(1.,1.),(1.,1.),(1.,1.),(1.,1.),(1.,1.),(1.,1.),(1.,1.),(1.,1.),(1.,
1.),(1.,1.),(1.,1.),(1.,1.),(1.,1.),(1.,1.),(1.,1.),(1.,1.),(1.,1.),(1.,
1.),(1.,1.),(1.,1.),(1.,1.),(1.,1.),(1.,1.),(1.,1.),(1.,1.),(1.,1.),(1.,
1.),(1.,1.),(1.,1.),(1.,1.),(1.,1.),(1.,1.),(1.,1.),(1.,1.),(1.,1.),(1.,
1.),(1.,1.),(1.,1.),(1.,1.),(1.,1.),(1.,1.),(1.,1.),(1.,1.),(1.,1.),(1.,
1.),(1.,1.)))
REPRESENTATION_ITEM('')
SURFACE()
);
#30=(
BOUNDED_SURFACE()
B_SPLINE_SURFACE(5,1,((#29884,#29885),(#29886,#29887),(#29888,#29889),(#29890,
#29891),(#29892,#29893),(#29894,#29895),(#29896,#29897),(#29898,#29899),
(#29900,#29901),(#29902,#29903),(#29904,#29905),(#29906,#29907),(#29908,
#29909),(#29910,#29911),(#29912,#29913),(#29914,#29915),(#29916,#29917),
(#29918,#29919),(#29920,#29921),(#29922,#29923),(#29924,#29925),(#29926,
#29927),(#29928,#29929),(#29930,#29931),(#29932,#29933),(#29934,#29935),
(#29936,#29937),(#29938,#29939),(#29940,#29941),(#29942,#29943),(#29944,
#29945),(#29946,#29947),(#29948,#29949),(#29950,#29951),(#29952,#29953),
(#29954,#29955),(#29956,#29957),(#29958,#29959),(#29960,#29961),(#29962,
#29963),(#29964,#29965),(#29966,#29967),(#29968,#29969),(#29970,#29971),
(#29972,#29973),(#29974,#29975),(#29976,#29977),(#29978,#29979),(#29980,
#29981),(#29982,#29983),(#29984,#29985),(#29986,#29987),(#29988,#29989),
(#29990,#29991),(#29992,#29993),(#29994,#29995),(#29996,#29997),(#29998,
#29999),(#30000,#30001),(#30002,#30003),(#30004,#30005),(#30006,#30007),
(#30008,#30009),(#30010,#30011),(#30012,#30013),(#30014,#30015),(#30016,
#30017),(#30018,#30019),(#30020,#30021),(#30022,#30023)),.UNSPECIFIED.,
 .F.,.F.,.F.)
B_SPLINE_SURFACE_WITH_KNOTS((6,1,1,1,1,1,1,1,1,1,1,1,1,1,1,1,1,1,1,1,1,
1,1,1,1,1,1,1,1,1,1,1,1,1,1,1,1,1,1,1,1,1,1,1,1,1,1,1,1,1,1,1,1,1,1,1,1,
1,1,1,1,1,1,1,1,6),(2,2),(-1.,-0.984615384615383,-0.969230769230768,-0.953846153846152,
-0.938461538461537,-0.923076923076922,-0.907692307692306,-0.892307692307691,
-0.876923076923076,-0.86153846153846,-0.846153846153845,-0.83076923076923,
-0.815384615384614,-0.799999999999999,-0.784615384615384,-0.769230769230768,
-0.753846153846153,-0.738461538461538,-0.723076923076922,-0.707692307692307,
-0.692307692307692,-0.676923076923076,-0.661538461538461,-0.646153846153846,
-0.63076923076923,-0.615384615384615,-0.6,-0.584615384615384,-0.569230769230769,
-0.553846153846154,-0.538461538461538,-0.523076923076923,-0.507692307692308,
-0.492307692307692,-0.476923076923077,-0.461538461538462,-0.446153846153846,
-0.430769230769231,-0.415384615384615,-0.4,-0.384615384615385,-0.369230769230769,
-0.353846153846154,-0.338461538461538,-0.323076923076923,-0.307692307692308,
-0.292307692307692,-0.276923076923077,-0.261538461538462,-0.246153846153846,
-0.230769230769231,-0.215384615384615,-0.2,-0.184615384615385,-0.169230769230769,
-0.153846153846154,-0.138461538461538,-0.123076923076923,-0.107692307692308,
-0.0923076923076923,-0.0769230769230769,-0.0615384615384615,-0.0461538461538462,
-0.0307692307692308,-0.0153846153846154,0.),(-1.,1.),.UNSPECIFIED.)
GEOMETRIC_REPRESENTATION_ITEM()
RATIONAL_B_SPLINE_SURFACE(((1.,1.),(1.,1.),(1.,1.),(1.,1.),(1.,1.),(1.,
1.),(1.,1.),(1.,1.),(1.,1.),(1.,1.),(1.,1.),(1.,1.),(1.,1.),(1.,1.),(1.,
1.),(1.,1.),(1.,1.),(1.,1.),(1.,1.),(1.,1.),(1.,1.),(1.,1.),(1.,1.),(1.,
1.),(1.,1.),(1.,1.),(1.,1.),(1.,1.),(1.,1.),(1.,1.),(1.,1.),(1.,1.),(1.,
1.),(1.,1.),(1.,1.),(1.,1.),(1.,1.),(1.,1.),(1.,1.),(1.,1.),(1.,1.),(1.,
1.),(1.,1.),(1.,1.),(1.,1.),(1.,1.),(1.,1.),(1.,1.),(1.,1.),(1.,1.),(1.,
1.),(1.,1.),(1.,1.),(1.,1.),(1.,1.),(1.,1.),(1.,1.),(1.,1.),(1.,1.),(1.,
1.),(1.,1.),(1.,1.),(1.,1.),(1.,1.),(1.,1.),(1.,1.),(1.,1.),(1.,1.),(1.,
1.),(1.,1.)))
REPRESENTATION_ITEM('')
SURFACE()
);
#31=(
BOUNDED_SURFACE()
B_SPLINE_SURFACE(5,1,((#30100,#30101),(#30102,#30103),(#30104,#30105),(#30106,
#30107),(#30108,#30109),(#30110,#30111),(#30112,#30113),(#30114,#30115),
(#30116,#30117),(#30118,#30119),(#30120,#30121),(#30122,#30123),(#30124,
#30125),(#30126,#30127),(#30128,#30129),(#30130,#30131),(#30132,#30133),
(#30134,#30135),(#30136,#30137),(#30138,#30139),(#30140,#30141),(#30142,
#30143),(#30144,#30145),(#30146,#30147),(#30148,#30149),(#30150,#30151),
(#30152,#30153),(#30154,#30155),(#30156,#30157),(#30158,#30159),(#30160,
#30161),(#30162,#30163),(#30164,#30165),(#30166,#30167),(#30168,#30169),
(#30170,#30171),(#30172,#30173),(#30174,#30175),(#30176,#30177),(#30178,
#30179),(#30180,#30181),(#30182,#30183),(#30184,#30185),(#30186,#30187),
(#30188,#30189),(#30190,#30191),(#30192,#30193),(#30194,#30195),(#30196,
#30197),(#30198,#30199),(#30200,#30201),(#30202,#30203),(#30204,#30205),
(#30206,#30207),(#30208,#30209),(#30210,#30211),(#30212,#30213),(#30214,
#30215),(#30216,#30217),(#30218,#30219),(#30220,#30221),(#30222,#30223),
(#30224,#30225),(#30226,#30227),(#30228,#30229),(#30230,#30231),(#30232,
#30233),(#30234,#30235),(#30236,#30237),(#30238,#30239)),.UNSPECIFIED.,
 .F.,.F.,.F.)
B_SPLINE_SURFACE_WITH_KNOTS((6,1,1,1,1,1,1,1,1,1,1,1,1,1,1,1,1,1,1,1,1,
1,1,1,1,1,1,1,1,1,1,1,1,1,1,1,1,1,1,1,1,1,1,1,1,1,1,1,1,1,1,1,1,1,1,1,1,
1,1,1,1,1,1,1,1,6),(2,2),(-1.,-0.984615384615383,-0.969230769230768,-0.953846153846152,
-0.938461538461537,-0.923076923076922,-0.907692307692306,-0.892307692307691,
-0.876923076923076,-0.86153846153846,-0.846153846153845,-0.83076923076923,
-0.815384615384614,-0.799999999999999,-0.784615384615384,-0.769230769230768,
-0.753846153846153,-0.738461538461538,-0.723076923076922,-0.707692307692307,
-0.692307692307692,-0.676923076923076,-0.661538461538461,-0.646153846153846,
-0.63076923076923,-0.615384615384615,-0.6,-0.584615384615384,-0.569230769230769,
-0.553846153846154,-0.538461538461538,-0.523076923076923,-0.507692307692308,
-0.492307692307692,-0.476923076923077,-0.461538461538462,-0.446153846153846,
-0.430769230769231,-0.415384615384615,-0.4,-0.384615384615385,-0.369230769230769,
-0.353846153846154,-0.338461538461538,-0.323076923076923,-0.307692307692308,
-0.292307692307692,-0.276923076923077,-0.261538461538462,-0.246153846153846,
-0.230769230769231,-0.215384615384615,-0.2,-0.184615384615385,-0.169230769230769,
-0.153846153846154,-0.138461538461538,-0.123076923076923,-0.107692307692308,
-0.0923076923076923,-0.0769230769230769,-0.0615384615384615,-0.0461538461538462,
-0.0307692307692308,-0.0153846153846154,0.),(-1.,1.),.UNSPECIFIED.)
GEOMETRIC_REPRESENTATION_ITEM()
RATIONAL_B_SPLINE_SURFACE(((1.,1.),(1.,1.),(1.,1.),(1.,1.),(1.,1.),(1.,
1.),(1.,1.),(1.,1.),(1.,1.),(1.,1.),(1.,1.),(1.,1.),(1.,1.),(1.,1.),(1.,
1.),(1.,1.),(1.,1.),(1.,1.),(1.,1.),(1.,1.),(1.,1.),(1.,1.),(1.,1.),(1.,
1.),(1.,1.),(1.,1.),(1.,1.),(1.,1.),(1.,1.),(1.,1.),(1.,1.),(1.,1.),(1.,
1.),(1.,1.),(1.,1.),(1.,1.),(1.,1.),(1.,1.),(1.,1.),(1.,1.),(1.,1.),(1.,
1.),(1.,1.),(1.,1.),(1.,1.),(1.,1.),(1.,1.),(1.,1.),(1.,1.),(1.,1.),(1.,
1.),(1.,1.),(1.,1.),(1.,1.),(1.,1.),(1.,1.),(1.,1.),(1.,1.),(1.,1.),(1.,
1.),(1.,1.),(1.,1.),(1.,1.),(1.,1.),(1.,1.),(1.,1.),(1.,1.),(1.,1.),(1.,
1.),(1.,1.)))
REPRESENTATION_ITEM('')
SURFACE()
);
#32=(
BOUNDED_SURFACE()
B_SPLINE_SURFACE(5,1,((#30316,#30317),(#30318,#30319),(#30320,#30321),(#30322,
#30323),(#30324,#30325),(#30326,#30327),(#30328,#30329),(#30330,#30331),
(#30332,#30333),(#30334,#30335),(#30336,#30337),(#30338,#30339),(#30340,
#30341),(#30342,#30343),(#30344,#30345),(#30346,#30347),(#30348,#30349),
(#30350,#30351),(#30352,#30353),(#30354,#30355),(#30356,#30357),(#30358,
#30359),(#30360,#30361),(#30362,#30363),(#30364,#30365),(#30366,#30367),
(#30368,#30369),(#30370,#30371),(#30372,#30373),(#30374,#30375),(#30376,
#30377),(#30378,#30379),(#30380,#30381),(#30382,#30383),(#30384,#30385),
(#30386,#30387),(#30388,#30389),(#30390,#30391),(#30392,#30393),(#30394,
#30395),(#30396,#30397),(#30398,#30399),(#30400,#30401),(#30402,#30403),
(#30404,#30405),(#30406,#30407),(#30408,#30409),(#30410,#30411),(#30412,
#30413),(#30414,#30415),(#30416,#30417),(#30418,#30419),(#30420,#30421),
(#30422,#30423),(#30424,#30425),(#30426,#30427),(#30428,#30429),(#30430,
#30431),(#30432,#30433),(#30434,#30435),(#30436,#30437),(#30438,#30439),
(#30440,#30441),(#30442,#30443),(#30444,#30445),(#30446,#30447),(#30448,
#30449),(#30450,#30451),(#30452,#30453),(#30454,#30455)),.UNSPECIFIED.,
 .F.,.F.,.F.)
B_SPLINE_SURFACE_WITH_KNOTS((6,1,1,1,1,1,1,1,1,1,1,1,1,1,1,1,1,1,1,1,1,
1,1,1,1,1,1,1,1,1,1,1,1,1,1,1,1,1,1,1,1,1,1,1,1,1,1,1,1,1,1,1,1,1,1,1,1,
1,1,1,1,1,1,1,1,6),(2,2),(-1.,-0.984615384615383,-0.969230769230768,-0.953846153846152,
-0.938461538461537,-0.923076923076922,-0.907692307692306,-0.892307692307691,
-0.876923076923076,-0.86153846153846,-0.846153846153845,-0.83076923076923,
-0.815384615384614,-0.799999999999999,-0.784615384615384,-0.769230769230768,
-0.753846153846153,-0.738461538461538,-0.723076923076922,-0.707692307692307,
-0.692307692307692,-0.676923076923076,-0.661538461538461,-0.646153846153846,
-0.63076923076923,-0.615384615384615,-0.6,-0.584615384615384,-0.569230769230769,
-0.553846153846154,-0.538461538461538,-0.523076923076923,-0.507692307692308,
-0.492307692307692,-0.476923076923077,-0.461538461538462,-0.446153846153846,
-0.430769230769231,-0.415384615384615,-0.4,-0.384615384615385,-0.369230769230769,
-0.353846153846154,-0.338461538461538,-0.323076923076923,-0.307692307692308,
-0.292307692307692,-0.276923076923077,-0.261538461538462,-0.246153846153846,
-0.230769230769231,-0.215384615384615,-0.2,-0.184615384615385,-0.169230769230769,
-0.153846153846154,-0.138461538461538,-0.123076923076923,-0.107692307692308,
-0.0923076923076923,-0.0769230769230769,-0.0615384615384615,-0.0461538461538462,
-0.0307692307692308,-0.0153846153846154,0.),(-1.,1.),.UNSPECIFIED.)
GEOMETRIC_REPRESENTATION_ITEM()
RATIONAL_B_SPLINE_SURFACE(((1.,1.),(1.,1.),(1.,1.),(1.,1.),(1.,1.),(1.,
1.),(1.,1.),(1.,1.),(1.,1.),(1.,1.),(1.,1.),(1.,1.),(1.,1.),(1.,1.),(1.,
1.),(1.,1.),(1.,1.),(1.,1.),(1.,1.),(1.,1.),(1.,1.),(1.,1.),(1.,1.),(1.,
1.),(1.,1.),(1.,1.),(1.,1.),(1.,1.),(1.,1.),(1.,1.),(1.,1.),(1.,1.),(1.,
1.),(1.,1.),(1.,1.),(1.,1.),(1.,1.),(1.,1.),(1.,1.),(1.,1.),(1.,1.),(1.,
1.),(1.,1.),(1.,1.),(1.,1.),(1.,1.),(1.,1.),(1.,1.),(1.,1.),(1.,1.),(1.,
1.),(1.,1.),(1.,1.),(1.,1.),(1.,1.),(1.,1.),(1.,1.),(1.,1.),(1.,1.),(1.,
1.),(1.,1.),(1.,1.),(1.,1.),(1.,1.),(1.,1.),(1.,1.),(1.,1.),(1.,1.),(1.,
1.),(1.,1.)))
REPRESENTATION_ITEM('')
SURFACE()
);
#33=(
BOUNDED_SURFACE()
B_SPLINE_SURFACE(5,1,((#30532,#30533),(#30534,#30535),(#30536,#30537),(#30538,
#30539),(#30540,#30541),(#30542,#30543),(#30544,#30545),(#30546,#30547),
(#30548,#30549),(#30550,#30551),(#30552,#30553),(#30554,#30555),(#30556,
#30557),(#30558,#30559),(#30560,#30561),(#30562,#30563),(#30564,#30565),
(#30566,#30567),(#30568,#30569),(#30570,#30571),(#30572,#30573),(#30574,
#30575),(#30576,#30577),(#30578,#30579),(#30580,#30581),(#30582,#30583),
(#30584,#30585),(#30586,#30587),(#30588,#30589),(#30590,#30591),(#30592,
#30593),(#30594,#30595),(#30596,#30597),(#30598,#30599),(#30600,#30601),
(#30602,#30603),(#30604,#30605),(#30606,#30607),(#30608,#30609),(#30610,
#30611),(#30612,#30613),(#30614,#30615),(#30616,#30617),(#30618,#30619),
(#30620,#30621),(#30622,#30623),(#30624,#30625),(#30626,#30627),(#30628,
#30629),(#30630,#30631),(#30632,#30633),(#30634,#30635),(#30636,#30637),
(#30638,#30639),(#30640,#30641),(#30642,#30643),(#30644,#30645),(#30646,
#30647),(#30648,#30649),(#30650,#30651),(#30652,#30653),(#30654,#30655),
(#30656,#30657),(#30658,#30659),(#30660,#30661),(#30662,#30663),(#30664,
#30665),(#30666,#30667),(#30668,#30669),(#30670,#30671)),.UNSPECIFIED.,
 .F.,.F.,.F.)
B_SPLINE_SURFACE_WITH_KNOTS((6,1,1,1,1,1,1,1,1,1,1,1,1,1,1,1,1,1,1,1,1,
1,1,1,1,1,1,1,1,1,1,1,1,1,1,1,1,1,1,1,1,1,1,1,1,1,1,1,1,1,1,1,1,1,1,1,1,
1,1,1,1,1,1,1,1,6),(2,2),(-1.,-0.984615384615383,-0.969230769230768,-0.953846153846152,
-0.938461538461537,-0.923076923076922,-0.907692307692306,-0.892307692307691,
-0.876923076923076,-0.86153846153846,-0.846153846153845,-0.83076923076923,
-0.815384615384614,-0.799999999999999,-0.784615384615384,-0.769230769230768,
-0.753846153846153,-0.738461538461538,-0.723076923076922,-0.707692307692307,
-0.692307692307692,-0.676923076923076,-0.661538461538461,-0.646153846153846,
-0.63076923076923,-0.615384615384615,-0.6,-0.584615384615384,-0.569230769230769,
-0.553846153846154,-0.538461538461538,-0.523076923076923,-0.507692307692308,
-0.492307692307692,-0.476923076923077,-0.461538461538462,-0.446153846153846,
-0.430769230769231,-0.415384615384615,-0.4,-0.384615384615385,-0.369230769230769,
-0.353846153846154,-0.338461538461538,-0.323076923076923,-0.307692307692308,
-0.292307692307692,-0.276923076923077,-0.261538461538462,-0.246153846153846,
-0.230769230769231,-0.215384615384615,-0.2,-0.184615384615385,-0.169230769230769,
-0.153846153846154,-0.138461538461538,-0.123076923076923,-0.107692307692308,
-0.0923076923076923,-0.0769230769230769,-0.0615384615384615,-0.0461538461538462,
-0.0307692307692308,-0.0153846153846154,0.),(-1.,1.),.UNSPECIFIED.)
GEOMETRIC_REPRESENTATION_ITEM()
RATIONAL_B_SPLINE_SURFACE(((1.,1.),(1.,1.),(1.,1.),(1.,1.),(1.,1.),(1.,
1.),(1.,1.),(1.,1.),(1.,1.),(1.,1.),(1.,1.),(1.,1.),(1.,1.),(1.,1.),(1.,
1.),(1.,1.),(1.,1.),(1.,1.),(1.,1.),(1.,1.),(1.,1.),(1.,1.),(1.,1.),(1.,
1.),(1.,1.),(1.,1.),(1.,1.),(1.,1.),(1.,1.),(1.,1.),(1.,1.),(1.,1.),(1.,
1.),(1.,1.),(1.,1.),(1.,1.),(1.,1.),(1.,1.),(1.,1.),(1.,1.),(1.,1.),(1.,
1.),(1.,1.),(1.,1.),(1.,1.),(1.,1.),(1.,1.),(1.,1.),(1.,1.),(1.,1.),(1.,
1.),(1.,1.),(1.,1.),(1.,1.),(1.,1.),(1.,1.),(1.,1.),(1.,1.),(1.,1.),(1.,
1.),(1.,1.),(1.,1.),(1.,1.),(1.,1.),(1.,1.),(1.,1.),(1.,1.),(1.,1.),(1.,
1.),(1.,1.)))
REPRESENTATION_ITEM('')
SURFACE()
);
#34=(
BOUNDED_SURFACE()
B_SPLINE_SURFACE(5,1,((#30748,#30749),(#30750,#30751),(#30752,#30753),(#30754,
#30755),(#30756,#30757),(#30758,#30759),(#30760,#30761),(#30762,#30763),
(#30764,#30765),(#30766,#30767),(#30768,#30769),(#30770,#30771),(#30772,
#30773),(#30774,#30775),(#30776,#30777),(#30778,#30779),(#30780,#30781),
(#30782,#30783),(#30784,#30785),(#30786,#30787),(#30788,#30789),(#30790,
#30791),(#30792,#30793),(#30794,#30795),(#30796,#30797),(#30798,#30799),
(#30800,#30801),(#30802,#30803),(#30804,#30805),(#30806,#30807),(#30808,
#30809),(#30810,#30811),(#30812,#30813),(#30814,#30815),(#30816,#30817),
(#30818,#30819),(#30820,#30821),(#30822,#30823),(#30824,#30825),(#30826,
#30827),(#30828,#30829),(#30830,#30831),(#30832,#30833),(#30834,#30835),
(#30836,#30837),(#30838,#30839),(#30840,#30841),(#30842,#30843),(#30844,
#30845),(#30846,#30847),(#30848,#30849),(#30850,#30851),(#30852,#30853),
(#30854,#30855),(#30856,#30857),(#30858,#30859),(#30860,#30861),(#30862,
#30863),(#30864,#30865),(#30866,#30867),(#30868,#30869),(#30870,#30871),
(#30872,#30873),(#30874,#30875),(#30876,#30877),(#30878,#30879),(#30880,
#30881),(#30882,#30883),(#30884,#30885),(#30886,#30887)),.UNSPECIFIED.,
 .F.,.F.,.F.)
B_SPLINE_SURFACE_WITH_KNOTS((6,1,1,1,1,1,1,1,1,1,1,1,1,1,1,1,1,1,1,1,1,
1,1,1,1,1,1,1,1,1,1,1,1,1,1,1,1,1,1,1,1,1,1,1,1,1,1,1,1,1,1,1,1,1,1,1,1,
1,1,1,1,1,1,1,1,6),(2,2),(-1.,-0.984615384615383,-0.969230769230768,-0.953846153846152,
-0.938461538461537,-0.923076923076922,-0.907692307692306,-0.892307692307691,
-0.876923076923076,-0.86153846153846,-0.846153846153845,-0.83076923076923,
-0.815384615384614,-0.799999999999999,-0.784615384615384,-0.769230769230768,
-0.753846153846153,-0.738461538461538,-0.723076923076922,-0.707692307692307,
-0.692307692307692,-0.676923076923076,-0.661538461538461,-0.646153846153846,
-0.63076923076923,-0.615384615384615,-0.6,-0.584615384615384,-0.569230769230769,
-0.553846153846154,-0.538461538461538,-0.523076923076923,-0.507692307692308,
-0.492307692307692,-0.476923076923077,-0.461538461538462,-0.446153846153846,
-0.430769230769231,-0.415384615384615,-0.4,-0.384615384615385,-0.369230769230769,
-0.353846153846154,-0.338461538461538,-0.323076923076923,-0.307692307692308,
-0.292307692307692,-0.276923076923077,-0.261538461538462,-0.246153846153846,
-0.230769230769231,-0.215384615384615,-0.2,-0.184615384615385,-0.169230769230769,
-0.153846153846154,-0.138461538461538,-0.123076923076923,-0.107692307692308,
-0.0923076923076923,-0.0769230769230769,-0.0615384615384615,-0.0461538461538462,
-0.0307692307692308,-0.0153846153846154,0.),(-1.,1.),.UNSPECIFIED.)
GEOMETRIC_REPRESENTATION_ITEM()
RATIONAL_B_SPLINE_SURFACE(((1.,1.),(1.,1.),(1.,1.),(1.,1.),(1.,1.),(1.,
1.),(1.,1.),(1.,1.),(1.,1.),(1.,1.),(1.,1.),(1.,1.),(1.,1.),(1.,1.),(1.,
1.),(1.,1.),(1.,1.),(1.,1.),(1.,1.),(1.,1.),(1.,1.),(1.,1.),(1.,1.),(1.,
1.),(1.,1.),(1.,1.),(1.,1.),(1.,1.),(1.,1.),(1.,1.),(1.,1.),(1.,1.),(1.,
1.),(1.,1.),(1.,1.),(1.,1.),(1.,1.),(1.,1.),(1.,1.),(1.,1.),(1.,1.),(1.,
1.),(1.,1.),(1.,1.),(1.,1.),(1.,1.),(1.,1.),(1.,1.),(1.,1.),(1.,1.),(1.,
1.),(1.,1.),(1.,1.),(1.,1.),(1.,1.),(1.,1.),(1.,1.),(1.,1.),(1.,1.),(1.,
1.),(1.,1.),(1.,1.),(1.,1.),(1.,1.),(1.,1.),(1.,1.),(1.,1.),(1.,1.),(1.,
1.),(1.,1.)))
REPRESENTATION_ITEM('')
SURFACE()
);
#35=(
BOUNDED_SURFACE()
B_SPLINE_SURFACE(5,1,((#30964,#30965),(#30966,#30967),(#30968,#30969),(#30970,
#30971),(#30972,#30973),(#30974,#30975),(#30976,#30977),(#30978,#30979),
(#30980,#30981),(#30982,#30983),(#30984,#30985),(#30986,#30987),(#30988,
#30989),(#30990,#30991),(#30992,#30993),(#30994,#30995),(#30996,#30997),
(#30998,#30999),(#31000,#31001),(#31002,#31003),(#31004,#31005),(#31006,
#31007),(#31008,#31009),(#31010,#31011),(#31012,#31013),(#31014,#31015),
(#31016,#31017),(#31018,#31019),(#31020,#31021),(#31022,#31023),(#31024,
#31025),(#31026,#31027),(#31028,#31029),(#31030,#31031),(#31032,#31033),
(#31034,#31035),(#31036,#31037),(#31038,#31039),(#31040,#31041),(#31042,
#31043),(#31044,#31045),(#31046,#31047),(#31048,#31049),(#31050,#31051),
(#31052,#31053),(#31054,#31055),(#31056,#31057),(#31058,#31059),(#31060,
#31061),(#31062,#31063),(#31064,#31065),(#31066,#31067),(#31068,#31069),
(#31070,#31071),(#31072,#31073),(#31074,#31075),(#31076,#31077),(#31078,
#31079),(#31080,#31081),(#31082,#31083),(#31084,#31085),(#31086,#31087),
(#31088,#31089),(#31090,#31091),(#31092,#31093),(#31094,#31095),(#31096,
#31097),(#31098,#31099),(#31100,#31101),(#31102,#31103)),.UNSPECIFIED.,
 .F.,.F.,.F.)
B_SPLINE_SURFACE_WITH_KNOTS((6,1,1,1,1,1,1,1,1,1,1,1,1,1,1,1,1,1,1,1,1,
1,1,1,1,1,1,1,1,1,1,1,1,1,1,1,1,1,1,1,1,1,1,1,1,1,1,1,1,1,1,1,1,1,1,1,1,
1,1,1,1,1,1,1,1,6),(2,2),(-1.,-0.984615384615383,-0.969230769230768,-0.953846153846152,
-0.938461538461537,-0.923076923076922,-0.907692307692306,-0.892307692307691,
-0.876923076923076,-0.86153846153846,-0.846153846153845,-0.83076923076923,
-0.815384615384614,-0.799999999999999,-0.784615384615384,-0.769230769230768,
-0.753846153846153,-0.738461538461538,-0.723076923076922,-0.707692307692307,
-0.692307692307692,-0.676923076923076,-0.661538461538461,-0.646153846153846,
-0.63076923076923,-0.615384615384615,-0.6,-0.584615384615384,-0.569230769230769,
-0.553846153846154,-0.538461538461538,-0.523076923076923,-0.507692307692308,
-0.492307692307692,-0.476923076923077,-0.461538461538462,-0.446153846153846,
-0.430769230769231,-0.415384615384615,-0.4,-0.384615384615385,-0.369230769230769,
-0.353846153846154,-0.338461538461538,-0.323076923076923,-0.307692307692308,
-0.292307692307692,-0.276923076923077,-0.261538461538462,-0.246153846153846,
-0.230769230769231,-0.215384615384615,-0.2,-0.184615384615385,-0.169230769230769,
-0.153846153846154,-0.138461538461538,-0.123076923076923,-0.107692307692308,
-0.0923076923076923,-0.0769230769230769,-0.0615384615384615,-0.0461538461538462,
-0.0307692307692308,-0.0153846153846154,0.),(-1.,1.),.UNSPECIFIED.)
GEOMETRIC_REPRESENTATION_ITEM()
RATIONAL_B_SPLINE_SURFACE(((1.,1.),(1.,1.),(1.,1.),(1.,1.),(1.,1.),(1.,
1.),(1.,1.),(1.,1.),(1.,1.),(1.,1.),(1.,1.),(1.,1.),(1.,1.),(1.,1.),(1.,
1.),(1.,1.),(1.,1.),(1.,1.),(1.,1.),(1.,1.),(1.,1.),(1.,1.),(1.,1.),(1.,
1.),(1.,1.),(1.,1.),(1.,1.),(1.,1.),(1.,1.),(1.,1.),(1.,1.),(1.,1.),(1.,
1.),(1.,1.),(1.,1.),(1.,1.),(1.,1.),(1.,1.),(1.,1.),(1.,1.),(1.,1.),(1.,
1.),(1.,1.),(1.,1.),(1.,1.),(1.,1.),(1.,1.),(1.,1.),(1.,1.),(1.,1.),(1.,
1.),(1.,1.),(1.,1.),(1.,1.),(1.,1.),(1.,1.),(1.,1.),(1.,1.),(1.,1.),(1.,
1.),(1.,1.),(1.,1.),(1.,1.),(1.,1.),(1.,1.),(1.,1.),(1.,1.),(1.,1.),(1.,
1.),(1.,1.)))
REPRESENTATION_ITEM('')
SURFACE()
);
#36=(
BOUNDED_SURFACE()
B_SPLINE_SURFACE(5,1,((#31180,#31181),(#31182,#31183),(#31184,#31185),(#31186,
#31187),(#31188,#31189),(#31190,#31191),(#31192,#31193),(#31194,#31195),
(#31196,#31197),(#31198,#31199),(#31200,#31201),(#31202,#31203),(#31204,
#31205),(#31206,#31207),(#31208,#31209),(#31210,#31211),(#31212,#31213),
(#31214,#31215),(#31216,#31217),(#31218,#31219),(#31220,#31221),(#31222,
#31223),(#31224,#31225),(#31226,#31227),(#31228,#31229),(#31230,#31231),
(#31232,#31233),(#31234,#31235),(#31236,#31237),(#31238,#31239),(#31240,
#31241),(#31242,#31243),(#31244,#31245),(#31246,#31247),(#31248,#31249),
(#31250,#31251),(#31252,#31253),(#31254,#31255),(#31256,#31257),(#31258,
#31259),(#31260,#31261),(#31262,#31263),(#31264,#31265),(#31266,#31267),
(#31268,#31269),(#31270,#31271),(#31272,#31273),(#31274,#31275),(#31276,
#31277),(#31278,#31279),(#31280,#31281),(#31282,#31283),(#31284,#31285),
(#31286,#31287),(#31288,#31289),(#31290,#31291),(#31292,#31293),(#31294,
#31295),(#31296,#31297),(#31298,#31299),(#31300,#31301),(#31302,#31303),
(#31304,#31305),(#31306,#31307),(#31308,#31309),(#31310,#31311),(#31312,
#31313),(#31314,#31315),(#31316,#31317),(#31318,#31319)),.UNSPECIFIED.,
 .F.,.F.,.F.)
B_SPLINE_SURFACE_WITH_KNOTS((6,1,1,1,1,1,1,1,1,1,1,1,1,1,1,1,1,1,1,1,1,
1,1,1,1,1,1,1,1,1,1,1,1,1,1,1,1,1,1,1,1,1,1,1,1,1,1,1,1,1,1,1,1,1,1,1,1,
1,1,1,1,1,1,1,1,6),(2,2),(-1.,-0.984615384615383,-0.969230769230768,-0.953846153846152,
-0.938461538461537,-0.923076923076922,-0.907692307692306,-0.892307692307691,
-0.876923076923076,-0.86153846153846,-0.846153846153845,-0.83076923076923,
-0.815384615384614,-0.799999999999999,-0.784615384615384,-0.769230769230768,
-0.753846153846153,-0.738461538461538,-0.723076923076922,-0.707692307692307,
-0.692307692307692,-0.676923076923076,-0.661538461538461,-0.646153846153846,
-0.63076923076923,-0.615384615384615,-0.6,-0.584615384615384,-0.569230769230769,
-0.553846153846154,-0.538461538461538,-0.523076923076923,-0.507692307692308,
-0.492307692307692,-0.476923076923077,-0.461538461538462,-0.446153846153846,
-0.430769230769231,-0.415384615384615,-0.4,-0.384615384615385,-0.369230769230769,
-0.353846153846154,-0.338461538461538,-0.323076923076923,-0.307692307692308,
-0.292307692307692,-0.276923076923077,-0.261538461538462,-0.246153846153846,
-0.230769230769231,-0.215384615384615,-0.2,-0.184615384615385,-0.169230769230769,
-0.153846153846154,-0.138461538461538,-0.123076923076923,-0.107692307692308,
-0.0923076923076923,-0.0769230769230769,-0.0615384615384615,-0.0461538461538462,
-0.0307692307692308,-0.0153846153846154,0.),(-1.,1.),.UNSPECIFIED.)
GEOMETRIC_REPRESENTATION_ITEM()
RATIONAL_B_SPLINE_SURFACE(((1.,1.),(1.,1.),(1.,1.),(1.,1.),(1.,1.),(1.,
1.),(1.,1.),(1.,1.),(1.,1.),(1.,1.),(1.,1.),(1.,1.),(1.,1.),(1.,1.),(1.,
1.),(1.,1.),(1.,1.),(1.,1.),(1.,1.),(1.,1.),(1.,1.),(1.,1.),(1.,1.),(1.,
1.),(1.,1.),(1.,1.),(1.,1.),(1.,1.),(1.,1.),(1.,1.),(1.,1.),(1.,1.),(1.,
1.),(1.,1.),(1.,1.),(1.,1.),(1.,1.),(1.,1.),(1.,1.),(1.,1.),(1.,1.),(1.,
1.),(1.,1.),(1.,1.),(1.,1.),(1.,1.),(1.,1.),(1.,1.),(1.,1.),(1.,1.),(1.,
1.),(1.,1.),(1.,1.),(1.,1.),(1.,1.),(1.,1.),(1.,1.),(1.,1.),(1.,1.),(1.,
1.),(1.,1.),(1.,1.),(1.,1.),(1.,1.),(1.,1.),(1.,1.),(1.,1.),(1.,1.),(1.,
1.),(1.,1.)))
REPRESENTATION_ITEM('')
SURFACE()
);
#37=(
BOUNDED_SURFACE()
B_SPLINE_SURFACE(5,1,((#31396,#31397),(#31398,#31399),(#31400,#31401),(#31402,
#31403),(#31404,#31405),(#31406,#31407),(#31408,#31409),(#31410,#31411),
(#31412,#31413),(#31414,#31415),(#31416,#31417),(#31418,#31419),(#31420,
#31421),(#31422,#31423),(#31424,#31425),(#31426,#31427),(#31428,#31429),
(#31430,#31431),(#31432,#31433),(#31434,#31435),(#31436,#31437),(#31438,
#31439),(#31440,#31441),(#31442,#31443),(#31444,#31445),(#31446,#31447),
(#31448,#31449),(#31450,#31451),(#31452,#31453),(#31454,#31455),(#31456,
#31457),(#31458,#31459),(#31460,#31461),(#31462,#31463),(#31464,#31465),
(#31466,#31467),(#31468,#31469),(#31470,#31471),(#31472,#31473),(#31474,
#31475),(#31476,#31477),(#31478,#31479),(#31480,#31481),(#31482,#31483),
(#31484,#31485),(#31486,#31487),(#31488,#31489),(#31490,#31491),(#31492,
#31493),(#31494,#31495),(#31496,#31497),(#31498,#31499),(#31500,#31501),
(#31502,#31503),(#31504,#31505),(#31506,#31507),(#31508,#31509),(#31510,
#31511),(#31512,#31513),(#31514,#31515),(#31516,#31517),(#31518,#31519),
(#31520,#31521),(#31522,#31523),(#31524,#31525),(#31526,#31527),(#31528,
#31529),(#31530,#31531),(#31532,#31533),(#31534,#31535)),.UNSPECIFIED.,
 .F.,.F.,.F.)
B_SPLINE_SURFACE_WITH_KNOTS((6,1,1,1,1,1,1,1,1,1,1,1,1,1,1,1,1,1,1,1,1,
1,1,1,1,1,1,1,1,1,1,1,1,1,1,1,1,1,1,1,1,1,1,1,1,1,1,1,1,1,1,1,1,1,1,1,1,
1,1,1,1,1,1,1,1,6),(2,2),(-1.,-0.984615384615383,-0.969230769230768,-0.953846153846152,
-0.938461538461537,-0.923076923076922,-0.907692307692306,-0.892307692307691,
-0.876923076923076,-0.86153846153846,-0.846153846153845,-0.83076923076923,
-0.815384615384614,-0.799999999999999,-0.784615384615384,-0.769230769230768,
-0.753846153846153,-0.738461538461538,-0.723076923076922,-0.707692307692307,
-0.692307692307692,-0.676923076923076,-0.661538461538461,-0.646153846153846,
-0.63076923076923,-0.615384615384615,-0.6,-0.584615384615384,-0.569230769230769,
-0.553846153846154,-0.538461538461538,-0.523076923076923,-0.507692307692308,
-0.492307692307692,-0.476923076923077,-0.461538461538462,-0.446153846153846,
-0.430769230769231,-0.415384615384615,-0.4,-0.384615384615385,-0.369230769230769,
-0.353846153846154,-0.338461538461538,-0.323076923076923,-0.307692307692308,
-0.292307692307692,-0.276923076923077,-0.261538461538462,-0.246153846153846,
-0.230769230769231,-0.215384615384615,-0.2,-0.184615384615385,-0.169230769230769,
-0.153846153846154,-0.138461538461538,-0.123076923076923,-0.107692307692308,
-0.0923076923076923,-0.0769230769230769,-0.0615384615384615,-0.0461538461538462,
-0.0307692307692308,-0.0153846153846154,0.),(-1.,1.),.UNSPECIFIED.)
GEOMETRIC_REPRESENTATION_ITEM()
RATIONAL_B_SPLINE_SURFACE(((1.,1.),(1.,1.),(1.,1.),(1.,1.),(1.,1.),(1.,
1.),(1.,1.),(1.,1.),(1.,1.),(1.,1.),(1.,1.),(1.,1.),(1.,1.),(1.,1.),(1.,
1.),(1.,1.),(1.,1.),(1.,1.),(1.,1.),(1.,1.),(1.,1.),(1.,1.),(1.,1.),(1.,
1.),(1.,1.),(1.,1.),(1.,1.),(1.,1.),(1.,1.),(1.,1.),(1.,1.),(1.,1.),(1.,
1.),(1.,1.),(1.,1.),(1.,1.),(1.,1.),(1.,1.),(1.,1.),(1.,1.),(1.,1.),(1.,
1.),(1.,1.),(1.,1.),(1.,1.),(1.,1.),(1.,1.),(1.,1.),(1.,1.),(1.,1.),(1.,
1.),(1.,1.),(1.,1.),(1.,1.),(1.,1.),(1.,1.),(1.,1.),(1.,1.),(1.,1.),(1.,
1.),(1.,1.),(1.,1.),(1.,1.),(1.,1.),(1.,1.),(1.,1.),(1.,1.),(1.,1.),(1.,
1.),(1.,1.)))
REPRESENTATION_ITEM('')
SURFACE()
);
#38=(
BOUNDED_SURFACE()
B_SPLINE_SURFACE(5,1,((#31612,#31613),(#31614,#31615),(#31616,#31617),(#31618,
#31619),(#31620,#31621),(#31622,#31623),(#31624,#31625),(#31626,#31627),
(#31628,#31629),(#31630,#31631),(#31632,#31633),(#31634,#31635),(#31636,
#31637),(#31638,#31639),(#31640,#31641),(#31642,#31643),(#31644,#31645),
(#31646,#31647),(#31648,#31649),(#31650,#31651),(#31652,#31653),(#31654,
#31655),(#31656,#31657),(#31658,#31659),(#31660,#31661),(#31662,#31663),
(#31664,#31665),(#31666,#31667),(#31668,#31669),(#31670,#31671),(#31672,
#31673),(#31674,#31675),(#31676,#31677),(#31678,#31679),(#31680,#31681),
(#31682,#31683),(#31684,#31685),(#31686,#31687),(#31688,#31689),(#31690,
#31691),(#31692,#31693),(#31694,#31695),(#31696,#31697),(#31698,#31699),
(#31700,#31701),(#31702,#31703),(#31704,#31705),(#31706,#31707),(#31708,
#31709),(#31710,#31711),(#31712,#31713),(#31714,#31715),(#31716,#31717),
(#31718,#31719),(#31720,#31721),(#31722,#31723),(#31724,#31725),(#31726,
#31727),(#31728,#31729),(#31730,#31731),(#31732,#31733),(#31734,#31735),
(#31736,#31737),(#31738,#31739),(#31740,#31741),(#31742,#31743),(#31744,
#31745),(#31746,#31747),(#31748,#31749),(#31750,#31751)),.UNSPECIFIED.,
 .F.,.F.,.F.)
B_SPLINE_SURFACE_WITH_KNOTS((6,1,1,1,1,1,1,1,1,1,1,1,1,1,1,1,1,1,1,1,1,
1,1,1,1,1,1,1,1,1,1,1,1,1,1,1,1,1,1,1,1,1,1,1,1,1,1,1,1,1,1,1,1,1,1,1,1,
1,1,1,1,1,1,1,1,6),(2,2),(-1.,-0.984615384615383,-0.969230769230768,-0.953846153846152,
-0.938461538461537,-0.923076923076922,-0.907692307692306,-0.892307692307691,
-0.876923076923076,-0.86153846153846,-0.846153846153845,-0.83076923076923,
-0.815384615384614,-0.799999999999999,-0.784615384615384,-0.769230769230768,
-0.753846153846153,-0.738461538461538,-0.723076923076922,-0.707692307692307,
-0.692307692307692,-0.676923076923076,-0.661538461538461,-0.646153846153846,
-0.63076923076923,-0.615384615384615,-0.6,-0.584615384615384,-0.569230769230769,
-0.553846153846154,-0.538461538461538,-0.523076923076923,-0.507692307692308,
-0.492307692307692,-0.476923076923077,-0.461538461538462,-0.446153846153846,
-0.430769230769231,-0.415384615384615,-0.4,-0.384615384615385,-0.369230769230769,
-0.353846153846154,-0.338461538461538,-0.323076923076923,-0.307692307692308,
-0.292307692307692,-0.276923076923077,-0.261538461538462,-0.246153846153846,
-0.230769230769231,-0.215384615384615,-0.2,-0.184615384615385,-0.169230769230769,
-0.153846153846154,-0.138461538461538,-0.123076923076923,-0.107692307692308,
-0.0923076923076923,-0.0769230769230769,-0.0615384615384615,-0.0461538461538462,
-0.0307692307692308,-0.0153846153846154,0.),(-1.,1.),.UNSPECIFIED.)
GEOMETRIC_REPRESENTATION_ITEM()
RATIONAL_B_SPLINE_SURFACE(((1.,1.),(1.,1.),(1.,1.),(1.,1.),(1.,1.),(1.,
1.),(1.,1.),(1.,1.),(1.,1.),(1.,1.),(1.,1.),(1.,1.),(1.,1.),(1.,1.),(1.,
1.),(1.,1.),(1.,1.),(1.,1.),(1.,1.),(1.,1.),(1.,1.),(1.,1.),(1.,1.),(1.,
1.),(1.,1.),(1.,1.),(1.,1.),(1.,1.),(1.,1.),(1.,1.),(1.,1.),(1.,1.),(1.,
1.),(1.,1.),(1.,1.),(1.,1.),(1.,1.),(1.,1.),(1.,1.),(1.,1.),(1.,1.),(1.,
1.),(1.,1.),(1.,1.),(1.,1.),(1.,1.),(1.,1.),(1.,1.),(1.,1.),(1.,1.),(1.,
1.),(1.,1.),(1.,1.),(1.,1.),(1.,1.),(1.,1.),(1.,1.),(1.,1.),(1.,1.),(1.,
1.),(1.,1.),(1.,1.),(1.,1.),(1.,1.),(1.,1.),(1.,1.),(1.,1.),(1.,1.),(1.,
1.),(1.,1.)))
REPRESENTATION_ITEM('')
SURFACE()
);
#39=(
BOUNDED_SURFACE()
B_SPLINE_SURFACE(5,1,((#31828,#31829),(#31830,#31831),(#31832,#31833),(#31834,
#31835),(#31836,#31837),(#31838,#31839),(#31840,#31841),(#31842,#31843),
(#31844,#31845),(#31846,#31847),(#31848,#31849),(#31850,#31851),(#31852,
#31853),(#31854,#31855),(#31856,#31857),(#31858,#31859),(#31860,#31861),
(#31862,#31863),(#31864,#31865),(#31866,#31867),(#31868,#31869),(#31870,
#31871),(#31872,#31873),(#31874,#31875),(#31876,#31877),(#31878,#31879),
(#31880,#31881),(#31882,#31883),(#31884,#31885),(#31886,#31887),(#31888,
#31889),(#31890,#31891),(#31892,#31893),(#31894,#31895),(#31896,#31897),
(#31898,#31899),(#31900,#31901),(#31902,#31903),(#31904,#31905),(#31906,
#31907),(#31908,#31909),(#31910,#31911),(#31912,#31913),(#31914,#31915),
(#31916,#31917),(#31918,#31919),(#31920,#31921),(#31922,#31923),(#31924,
#31925),(#31926,#31927),(#31928,#31929),(#31930,#31931),(#31932,#31933),
(#31934,#31935),(#31936,#31937),(#31938,#31939),(#31940,#31941),(#31942,
#31943),(#31944,#31945),(#31946,#31947),(#31948,#31949),(#31950,#31951),
(#31952,#31953),(#31954,#31955),(#31956,#31957),(#31958,#31959),(#31960,
#31961),(#31962,#31963),(#31964,#31965),(#31966,#31967)),.UNSPECIFIED.,
 .F.,.F.,.F.)
B_SPLINE_SURFACE_WITH_KNOTS((6,1,1,1,1,1,1,1,1,1,1,1,1,1,1,1,1,1,1,1,1,
1,1,1,1,1,1,1,1,1,1,1,1,1,1,1,1,1,1,1,1,1,1,1,1,1,1,1,1,1,1,1,1,1,1,1,1,
1,1,1,1,1,1,1,1,6),(2,2),(-1.,-0.984615384615383,-0.969230769230768,-0.953846153846152,
-0.938461538461537,-0.923076923076922,-0.907692307692306,-0.892307692307691,
-0.876923076923076,-0.86153846153846,-0.846153846153845,-0.83076923076923,
-0.815384615384614,-0.799999999999999,-0.784615384615384,-0.769230769230768,
-0.753846153846153,-0.738461538461538,-0.723076923076922,-0.707692307692307,
-0.692307692307692,-0.676923076923076,-0.661538461538461,-0.646153846153846,
-0.63076923076923,-0.615384615384615,-0.6,-0.584615384615384,-0.569230769230769,
-0.553846153846154,-0.538461538461538,-0.523076923076923,-0.507692307692308,
-0.492307692307692,-0.476923076923077,-0.461538461538462,-0.446153846153846,
-0.430769230769231,-0.415384615384615,-0.4,-0.384615384615385,-0.369230769230769,
-0.353846153846154,-0.338461538461538,-0.323076923076923,-0.307692307692308,
-0.292307692307692,-0.276923076923077,-0.261538461538462,-0.246153846153846,
-0.230769230769231,-0.215384615384615,-0.2,-0.184615384615385,-0.169230769230769,
-0.153846153846154,-0.138461538461538,-0.123076923076923,-0.107692307692308,
-0.0923076923076923,-0.0769230769230769,-0.0615384615384615,-0.0461538461538462,
-0.0307692307692308,-0.0153846153846154,0.),(-1.,1.),.UNSPECIFIED.)
GEOMETRIC_REPRESENTATION_ITEM()
RATIONAL_B_SPLINE_SURFACE(((1.,1.),(1.,1.),(1.,1.),(1.,1.),(1.,1.),(1.,
1.),(1.,1.),(1.,1.),(1.,1.),(1.,1.),(1.,1.),(1.,1.),(1.,1.),(1.,1.),(1.,
1.),(1.,1.),(1.,1.),(1.,1.),(1.,1.),(1.,1.),(1.,1.),(1.,1.),(1.,1.),(1.,
1.),(1.,1.),(1.,1.),(1.,1.),(1.,1.),(1.,1.),(1.,1.),(1.,1.),(1.,1.),(1.,
1.),(1.,1.),(1.,1.),(1.,1.),(1.,1.),(1.,1.),(1.,1.),(1.,1.),(1.,1.),(1.,
1.),(1.,1.),(1.,1.),(1.,1.),(1.,1.),(1.,1.),(1.,1.),(1.,1.),(1.,1.),(1.,
1.),(1.,1.),(1.,1.),(1.,1.),(1.,1.),(1.,1.),(1.,1.),(1.,1.),(1.,1.),(1.,
1.),(1.,1.),(1.,1.),(1.,1.),(1.,1.),(1.,1.),(1.,1.),(1.,1.),(1.,1.),(1.,
1.),(1.,1.)))
REPRESENTATION_ITEM('')
SURFACE()
);
#40=(
BOUNDED_SURFACE()
B_SPLINE_SURFACE(5,1,((#32044,#32045),(#32046,#32047),(#32048,#32049),(#32050,
#32051),(#32052,#32053),(#32054,#32055),(#32056,#32057),(#32058,#32059),
(#32060,#32061),(#32062,#32063),(#32064,#32065),(#32066,#32067),(#32068,
#32069),(#32070,#32071),(#32072,#32073),(#32074,#32075),(#32076,#32077),
(#32078,#32079),(#32080,#32081),(#32082,#32083),(#32084,#32085),(#32086,
#32087),(#32088,#32089),(#32090,#32091),(#32092,#32093),(#32094,#32095),
(#32096,#32097),(#32098,#32099),(#32100,#32101),(#32102,#32103),(#32104,
#32105),(#32106,#32107),(#32108,#32109),(#32110,#32111),(#32112,#32113),
(#32114,#32115),(#32116,#32117),(#32118,#32119),(#32120,#32121),(#32122,
#32123),(#32124,#32125),(#32126,#32127),(#32128,#32129),(#32130,#32131),
(#32132,#32133),(#32134,#32135),(#32136,#32137),(#32138,#32139),(#32140,
#32141),(#32142,#32143),(#32144,#32145),(#32146,#32147),(#32148,#32149),
(#32150,#32151),(#32152,#32153),(#32154,#32155),(#32156,#32157),(#32158,
#32159),(#32160,#32161),(#32162,#32163),(#32164,#32165),(#32166,#32167),
(#32168,#32169),(#32170,#32171),(#32172,#32173),(#32174,#32175),(#32176,
#32177),(#32178,#32179),(#32180,#32181),(#32182,#32183)),.UNSPECIFIED.,
 .F.,.F.,.F.)
B_SPLINE_SURFACE_WITH_KNOTS((6,1,1,1,1,1,1,1,1,1,1,1,1,1,1,1,1,1,1,1,1,
1,1,1,1,1,1,1,1,1,1,1,1,1,1,1,1,1,1,1,1,1,1,1,1,1,1,1,1,1,1,1,1,1,1,1,1,
1,1,1,1,1,1,1,1,6),(2,2),(-1.,-0.984615384615383,-0.969230769230768,-0.953846153846152,
-0.938461538461537,-0.923076923076922,-0.907692307692306,-0.892307692307691,
-0.876923076923076,-0.86153846153846,-0.846153846153845,-0.83076923076923,
-0.815384615384614,-0.799999999999999,-0.784615384615384,-0.769230769230768,
-0.753846153846153,-0.738461538461538,-0.723076923076922,-0.707692307692307,
-0.692307692307692,-0.676923076923076,-0.661538461538461,-0.646153846153846,
-0.63076923076923,-0.615384615384615,-0.6,-0.584615384615384,-0.569230769230769,
-0.553846153846154,-0.538461538461538,-0.523076923076923,-0.507692307692308,
-0.492307692307692,-0.476923076923077,-0.461538461538462,-0.446153846153846,
-0.430769230769231,-0.415384615384615,-0.4,-0.384615384615385,-0.369230769230769,
-0.353846153846154,-0.338461538461538,-0.323076923076923,-0.307692307692308,
-0.292307692307692,-0.276923076923077,-0.261538461538462,-0.246153846153846,
-0.230769230769231,-0.215384615384615,-0.2,-0.184615384615385,-0.169230769230769,
-0.153846153846154,-0.138461538461538,-0.123076923076923,-0.107692307692308,
-0.0923076923076923,-0.0769230769230769,-0.0615384615384615,-0.0461538461538462,
-0.0307692307692308,-0.0153846153846154,0.),(-1.,1.),.UNSPECIFIED.)
GEOMETRIC_REPRESENTATION_ITEM()
RATIONAL_B_SPLINE_SURFACE(((1.,1.),(1.,1.),(1.,1.),(1.,1.),(1.,1.),(1.,
1.),(1.,1.),(1.,1.),(1.,1.),(1.,1.),(1.,1.),(1.,1.),(1.,1.),(1.,1.),(1.,
1.),(1.,1.),(1.,1.),(1.,1.),(1.,1.),(1.,1.),(1.,1.),(1.,1.),(1.,1.),(1.,
1.),(1.,1.),(1.,1.),(1.,1.),(1.,1.),(1.,1.),(1.,1.),(1.,1.),(1.,1.),(1.,
1.),(1.,1.),(1.,1.),(1.,1.),(1.,1.),(1.,1.),(1.,1.),(1.,1.),(1.,1.),(1.,
1.),(1.,1.),(1.,1.),(1.,1.),(1.,1.),(1.,1.),(1.,1.),(1.,1.),(1.,1.),(1.,
1.),(1.,1.),(1.,1.),(1.,1.),(1.,1.),(1.,1.),(1.,1.),(1.,1.),(1.,1.),(1.,
1.),(1.,1.),(1.,1.),(1.,1.),(1.,1.),(1.,1.),(1.,1.),(1.,1.),(1.,1.),(1.,
1.),(1.,1.)))
REPRESENTATION_ITEM('')
SURFACE()
);
#41=(
BOUNDED_SURFACE()
B_SPLINE_SURFACE(5,1,((#32260,#32261),(#32262,#32263),(#32264,#32265),(#32266,
#32267),(#32268,#32269),(#32270,#32271),(#32272,#32273),(#32274,#32275),
(#32276,#32277),(#32278,#32279),(#32280,#32281),(#32282,#32283),(#32284,
#32285),(#32286,#32287),(#32288,#32289),(#32290,#32291),(#32292,#32293),
(#32294,#32295),(#32296,#32297),(#32298,#32299),(#32300,#32301),(#32302,
#32303),(#32304,#32305),(#32306,#32307),(#32308,#32309),(#32310,#32311),
(#32312,#32313),(#32314,#32315),(#32316,#32317),(#32318,#32319),(#32320,
#32321),(#32322,#32323),(#32324,#32325),(#32326,#32327),(#32328,#32329),
(#32330,#32331),(#32332,#32333),(#32334,#32335),(#32336,#32337),(#32338,
#32339),(#32340,#32341),(#32342,#32343),(#32344,#32345),(#32346,#32347),
(#32348,#32349),(#32350,#32351),(#32352,#32353),(#32354,#32355),(#32356,
#32357),(#32358,#32359),(#32360,#32361),(#32362,#32363),(#32364,#32365),
(#32366,#32367),(#32368,#32369),(#32370,#32371),(#32372,#32373),(#32374,
#32375),(#32376,#32377),(#32378,#32379),(#32380,#32381),(#32382,#32383),
(#32384,#32385),(#32386,#32387),(#32388,#32389),(#32390,#32391),(#32392,
#32393),(#32394,#32395),(#32396,#32397),(#32398,#32399)),.UNSPECIFIED.,
 .F.,.F.,.F.)
B_SPLINE_SURFACE_WITH_KNOTS((6,1,1,1,1,1,1,1,1,1,1,1,1,1,1,1,1,1,1,1,1,
1,1,1,1,1,1,1,1,1,1,1,1,1,1,1,1,1,1,1,1,1,1,1,1,1,1,1,1,1,1,1,1,1,1,1,1,
1,1,1,1,1,1,1,1,6),(2,2),(-1.,-0.984615384615383,-0.969230769230768,-0.953846153846152,
-0.938461538461537,-0.923076923076922,-0.907692307692306,-0.892307692307691,
-0.876923076923076,-0.86153846153846,-0.846153846153845,-0.83076923076923,
-0.815384615384614,-0.799999999999999,-0.784615384615384,-0.769230769230768,
-0.753846153846153,-0.738461538461538,-0.723076923076922,-0.707692307692307,
-0.692307692307692,-0.676923076923076,-0.661538461538461,-0.646153846153846,
-0.63076923076923,-0.615384615384615,-0.6,-0.584615384615384,-0.569230769230769,
-0.553846153846154,-0.538461538461538,-0.523076923076923,-0.507692307692308,
-0.492307692307692,-0.476923076923077,-0.461538461538462,-0.446153846153846,
-0.430769230769231,-0.415384615384615,-0.4,-0.384615384615385,-0.369230769230769,
-0.353846153846154,-0.338461538461538,-0.323076923076923,-0.307692307692308,
-0.292307692307692,-0.276923076923077,-0.261538461538462,-0.246153846153846,
-0.230769230769231,-0.215384615384615,-0.2,-0.184615384615385,-0.169230769230769,
-0.153846153846154,-0.138461538461538,-0.123076923076923,-0.107692307692308,
-0.0923076923076923,-0.0769230769230769,-0.0615384615384615,-0.0461538461538462,
-0.0307692307692308,-0.0153846153846154,0.),(-1.,1.),.UNSPECIFIED.)
GEOMETRIC_REPRESENTATION_ITEM()
RATIONAL_B_SPLINE_SURFACE(((1.,1.),(1.,1.),(1.,1.),(1.,1.),(1.,1.),(1.,
1.),(1.,1.),(1.,1.),(1.,1.),(1.,1.),(1.,1.),(1.,1.),(1.,1.),(1.,1.),(1.,
1.),(1.,1.),(1.,1.),(1.,1.),(1.,1.),(1.,1.),(1.,1.),(1.,1.),(1.,1.),(1.,
1.),(1.,1.),(1.,1.),(1.,1.),(1.,1.),(1.,1.),(1.,1.),(1.,1.),(1.,1.),(1.,
1.),(1.,1.),(1.,1.),(1.,1.),(1.,1.),(1.,1.),(1.,1.),(1.,1.),(1.,1.),(1.,
1.),(1.,1.),(1.,1.),(1.,1.),(1.,1.),(1.,1.),(1.,1.),(1.,1.),(1.,1.),(1.,
1.),(1.,1.),(1.,1.),(1.,1.),(1.,1.),(1.,1.),(1.,1.),(1.,1.),(1.,1.),(1.,
1.),(1.,1.),(1.,1.),(1.,1.),(1.,1.),(1.,1.),(1.,1.),(1.,1.),(1.,1.),(1.,
1.),(1.,1.)))
REPRESENTATION_ITEM('')
SURFACE()
);
#42=(
BOUNDED_SURFACE()
B_SPLINE_SURFACE(5,1,((#32476,#32477),(#32478,#32479),(#32480,#32481),(#32482,
#32483),(#32484,#32485),(#32486,#32487),(#32488,#32489),(#32490,#32491),
(#32492,#32493),(#32494,#32495),(#32496,#32497),(#32498,#32499),(#32500,
#32501),(#32502,#32503),(#32504,#32505),(#32506,#32507),(#32508,#32509),
(#32510,#32511),(#32512,#32513),(#32514,#32515),(#32516,#32517),(#32518,
#32519),(#32520,#32521),(#32522,#32523),(#32524,#32525),(#32526,#32527),
(#32528,#32529),(#32530,#32531),(#32532,#32533),(#32534,#32535),(#32536,
#32537),(#32538,#32539),(#32540,#32541),(#32542,#32543),(#32544,#32545),
(#32546,#32547),(#32548,#32549),(#32550,#32551),(#32552,#32553),(#32554,
#32555),(#32556,#32557),(#32558,#32559),(#32560,#32561),(#32562,#32563),
(#32564,#32565),(#32566,#32567),(#32568,#32569),(#32570,#32571),(#32572,
#32573),(#32574,#32575),(#32576,#32577),(#32578,#32579),(#32580,#32581),
(#32582,#32583),(#32584,#32585),(#32586,#32587),(#32588,#32589),(#32590,
#32591),(#32592,#32593),(#32594,#32595),(#32596,#32597),(#32598,#32599),
(#32600,#32601),(#32602,#32603),(#32604,#32605),(#32606,#32607),(#32608,
#32609),(#32610,#32611),(#32612,#32613),(#32614,#32615)),.UNSPECIFIED.,
 .F.,.F.,.F.)
B_SPLINE_SURFACE_WITH_KNOTS((6,1,1,1,1,1,1,1,1,1,1,1,1,1,1,1,1,1,1,1,1,
1,1,1,1,1,1,1,1,1,1,1,1,1,1,1,1,1,1,1,1,1,1,1,1,1,1,1,1,1,1,1,1,1,1,1,1,
1,1,1,1,1,1,1,1,6),(2,2),(-1.,-0.984615384615383,-0.969230769230768,-0.953846153846152,
-0.938461538461537,-0.923076923076922,-0.907692307692306,-0.892307692307691,
-0.876923076923076,-0.86153846153846,-0.846153846153845,-0.83076923076923,
-0.815384615384614,-0.799999999999999,-0.784615384615384,-0.769230769230768,
-0.753846153846153,-0.738461538461538,-0.723076923076922,-0.707692307692307,
-0.692307692307692,-0.676923076923076,-0.661538461538461,-0.646153846153846,
-0.63076923076923,-0.615384615384615,-0.6,-0.584615384615384,-0.569230769230769,
-0.553846153846154,-0.538461538461538,-0.523076923076923,-0.507692307692308,
-0.492307692307692,-0.476923076923077,-0.461538461538462,-0.446153846153846,
-0.430769230769231,-0.415384615384615,-0.4,-0.384615384615385,-0.369230769230769,
-0.353846153846154,-0.338461538461538,-0.323076923076923,-0.307692307692308,
-0.292307692307692,-0.276923076923077,-0.261538461538462,-0.246153846153846,
-0.230769230769231,-0.215384615384615,-0.2,-0.184615384615385,-0.169230769230769,
-0.153846153846154,-0.138461538461538,-0.123076923076923,-0.107692307692308,
-0.0923076923076923,-0.0769230769230769,-0.0615384615384615,-0.0461538461538462,
-0.0307692307692308,-0.0153846153846154,0.),(-1.,1.),.UNSPECIFIED.)
GEOMETRIC_REPRESENTATION_ITEM()
RATIONAL_B_SPLINE_SURFACE(((1.,1.),(1.,1.),(1.,1.),(1.,1.),(1.,1.),(1.,
1.),(1.,1.),(1.,1.),(1.,1.),(1.,1.),(1.,1.),(1.,1.),(1.,1.),(1.,1.),(1.,
1.),(1.,1.),(1.,1.),(1.,1.),(1.,1.),(1.,1.),(1.,1.),(1.,1.),(1.,1.),(1.,
1.),(1.,1.),(1.,1.),(1.,1.),(1.,1.),(1.,1.),(1.,1.),(1.,1.),(1.,1.),(1.,
1.),(1.,1.),(1.,1.),(1.,1.),(1.,1.),(1.,1.),(1.,1.),(1.,1.),(1.,1.),(1.,
1.),(1.,1.),(1.,1.),(1.,1.),(1.,1.),(1.,1.),(1.,1.),(1.,1.),(1.,1.),(1.,
1.),(1.,1.),(1.,1.),(1.,1.),(1.,1.),(1.,1.),(1.,1.),(1.,1.),(1.,1.),(1.,
1.),(1.,1.),(1.,1.),(1.,1.),(1.,1.),(1.,1.),(1.,1.),(1.,1.),(1.,1.),(1.,
1.),(1.,1.)))
REPRESENTATION_ITEM('')
SURFACE()
);
#43=(
BOUNDED_SURFACE()
B_SPLINE_SURFACE(5,1,((#32692,#32693),(#32694,#32695),(#32696,#32697),(#32698,
#32699),(#32700,#32701),(#32702,#32703),(#32704,#32705),(#32706,#32707),
(#32708,#32709),(#32710,#32711),(#32712,#32713),(#32714,#32715),(#32716,
#32717),(#32718,#32719),(#32720,#32721),(#32722,#32723),(#32724,#32725),
(#32726,#32727),(#32728,#32729),(#32730,#32731),(#32732,#32733),(#32734,
#32735),(#32736,#32737),(#32738,#32739),(#32740,#32741),(#32742,#32743),
(#32744,#32745),(#32746,#32747),(#32748,#32749),(#32750,#32751),(#32752,
#32753),(#32754,#32755),(#32756,#32757),(#32758,#32759),(#32760,#32761),
(#32762,#32763),(#32764,#32765),(#32766,#32767),(#32768,#32769),(#32770,
#32771),(#32772,#32773),(#32774,#32775),(#32776,#32777),(#32778,#32779),
(#32780,#32781),(#32782,#32783),(#32784,#32785),(#32786,#32787),(#32788,
#32789),(#32790,#32791),(#32792,#32793),(#32794,#32795),(#32796,#32797),
(#32798,#32799),(#32800,#32801),(#32802,#32803),(#32804,#32805),(#32806,
#32807),(#32808,#32809),(#32810,#32811),(#32812,#32813),(#32814,#32815),
(#32816,#32817),(#32818,#32819),(#32820,#32821),(#32822,#32823),(#32824,
#32825),(#32826,#32827),(#32828,#32829),(#32830,#32831)),.UNSPECIFIED.,
 .F.,.F.,.F.)
B_SPLINE_SURFACE_WITH_KNOTS((6,1,1,1,1,1,1,1,1,1,1,1,1,1,1,1,1,1,1,1,1,
1,1,1,1,1,1,1,1,1,1,1,1,1,1,1,1,1,1,1,1,1,1,1,1,1,1,1,1,1,1,1,1,1,1,1,1,
1,1,1,1,1,1,1,1,6),(2,2),(-1.,-0.984615384615383,-0.969230769230768,-0.953846153846152,
-0.938461538461537,-0.923076923076922,-0.907692307692306,-0.892307692307691,
-0.876923076923076,-0.86153846153846,-0.846153846153845,-0.83076923076923,
-0.815384615384614,-0.799999999999999,-0.784615384615384,-0.769230769230768,
-0.753846153846153,-0.738461538461538,-0.723076923076922,-0.707692307692307,
-0.692307692307692,-0.676923076923076,-0.661538461538461,-0.646153846153846,
-0.63076923076923,-0.615384615384615,-0.6,-0.584615384615384,-0.569230769230769,
-0.553846153846154,-0.538461538461538,-0.523076923076923,-0.507692307692308,
-0.492307692307692,-0.476923076923077,-0.461538461538462,-0.446153846153846,
-0.430769230769231,-0.415384615384615,-0.4,-0.384615384615385,-0.369230769230769,
-0.353846153846154,-0.338461538461538,-0.323076923076923,-0.307692307692308,
-0.292307692307692,-0.276923076923077,-0.261538461538462,-0.246153846153846,
-0.230769230769231,-0.215384615384615,-0.2,-0.184615384615385,-0.169230769230769,
-0.153846153846154,-0.138461538461538,-0.123076923076923,-0.107692307692308,
-0.0923076923076923,-0.0769230769230769,-0.0615384615384615,-0.0461538461538462,
-0.0307692307692308,-0.0153846153846154,0.),(-1.,1.),.UNSPECIFIED.)
GEOMETRIC_REPRESENTATION_ITEM()
RATIONAL_B_SPLINE_SURFACE(((1.,1.),(1.,1.),(1.,1.),(1.,1.),(1.,1.),(1.,
1.),(1.,1.),(1.,1.),(1.,1.),(1.,1.),(1.,1.),(1.,1.),(1.,1.),(1.,1.),(1.,
1.),(1.,1.),(1.,1.),(1.,1.),(1.,1.),(1.,1.),(1.,1.),(1.,1.),(1.,1.),(1.,
1.),(1.,1.),(1.,1.),(1.,1.),(1.,1.),(1.,1.),(1.,1.),(1.,1.),(1.,1.),(1.,
1.),(1.,1.),(1.,1.),(1.,1.),(1.,1.),(1.,1.),(1.,1.),(1.,1.),(1.,1.),(1.,
1.),(1.,1.),(1.,1.),(1.,1.),(1.,1.),(1.,1.),(1.,1.),(1.,1.),(1.,1.),(1.,
1.),(1.,1.),(1.,1.),(1.,1.),(1.,1.),(1.,1.),(1.,1.),(1.,1.),(1.,1.),(1.,
1.),(1.,1.),(1.,1.),(1.,1.),(1.,1.),(1.,1.),(1.,1.),(1.,1.),(1.,1.),(1.,
1.),(1.,1.)))
REPRESENTATION_ITEM('')
SURFACE()
);
#44=(
BOUNDED_SURFACE()
B_SPLINE_SURFACE(5,1,((#32908,#32909),(#32910,#32911),(#32912,#32913),(#32914,
#32915),(#32916,#32917),(#32918,#32919),(#32920,#32921),(#32922,#32923),
(#32924,#32925),(#32926,#32927),(#32928,#32929),(#32930,#32931),(#32932,
#32933),(#32934,#32935),(#32936,#32937),(#32938,#32939),(#32940,#32941),
(#32942,#32943),(#32944,#32945),(#32946,#32947),(#32948,#32949),(#32950,
#32951),(#32952,#32953),(#32954,#32955),(#32956,#32957),(#32958,#32959),
(#32960,#32961),(#32962,#32963),(#32964,#32965),(#32966,#32967),(#32968,
#32969),(#32970,#32971),(#32972,#32973),(#32974,#32975),(#32976,#32977),
(#32978,#32979),(#32980,#32981),(#32982,#32983),(#32984,#32985),(#32986,
#32987),(#32988,#32989),(#32990,#32991),(#32992,#32993),(#32994,#32995),
(#32996,#32997),(#32998,#32999),(#33000,#33001),(#33002,#33003),(#33004,
#33005),(#33006,#33007),(#33008,#33009),(#33010,#33011),(#33012,#33013),
(#33014,#33015),(#33016,#33017),(#33018,#33019),(#33020,#33021),(#33022,
#33023),(#33024,#33025),(#33026,#33027),(#33028,#33029),(#33030,#33031),
(#33032,#33033),(#33034,#33035),(#33036,#33037),(#33038,#33039),(#33040,
#33041),(#33042,#33043),(#33044,#33045),(#33046,#33047)),.UNSPECIFIED.,
 .F.,.F.,.F.)
B_SPLINE_SURFACE_WITH_KNOTS((6,1,1,1,1,1,1,1,1,1,1,1,1,1,1,1,1,1,1,1,1,
1,1,1,1,1,1,1,1,1,1,1,1,1,1,1,1,1,1,1,1,1,1,1,1,1,1,1,1,1,1,1,1,1,1,1,1,
1,1,1,1,1,1,1,1,6),(2,2),(-1.,-0.984615384615383,-0.969230769230768,-0.953846153846152,
-0.938461538461537,-0.923076923076922,-0.907692307692306,-0.892307692307691,
-0.876923076923076,-0.86153846153846,-0.846153846153845,-0.83076923076923,
-0.815384615384614,-0.799999999999999,-0.784615384615384,-0.769230769230768,
-0.753846153846153,-0.738461538461538,-0.723076923076922,-0.707692307692307,
-0.692307692307692,-0.676923076923076,-0.661538461538461,-0.646153846153846,
-0.63076923076923,-0.615384615384615,-0.6,-0.584615384615384,-0.569230769230769,
-0.553846153846154,-0.538461538461538,-0.523076923076923,-0.507692307692308,
-0.492307692307692,-0.476923076923077,-0.461538461538462,-0.446153846153846,
-0.430769230769231,-0.415384615384615,-0.4,-0.384615384615385,-0.369230769230769,
-0.353846153846154,-0.338461538461538,-0.323076923076923,-0.307692307692308,
-0.292307692307692,-0.276923076923077,-0.261538461538462,-0.246153846153846,
-0.230769230769231,-0.215384615384615,-0.2,-0.184615384615385,-0.169230769230769,
-0.153846153846154,-0.138461538461538,-0.123076923076923,-0.107692307692308,
-0.0923076923076923,-0.0769230769230769,-0.0615384615384615,-0.0461538461538462,
-0.0307692307692308,-0.0153846153846154,0.),(-1.,1.),.UNSPECIFIED.)
GEOMETRIC_REPRESENTATION_ITEM()
RATIONAL_B_SPLINE_SURFACE(((1.,1.),(1.,1.),(1.,1.),(1.,1.),(1.,1.),(1.,
1.),(1.,1.),(1.,1.),(1.,1.),(1.,1.),(1.,1.),(1.,1.),(1.,1.),(1.,1.),(1.,
1.),(1.,1.),(1.,1.),(1.,1.),(1.,1.),(1.,1.),(1.,1.),(1.,1.),(1.,1.),(1.,
1.),(1.,1.),(1.,1.),(1.,1.),(1.,1.),(1.,1.),(1.,1.),(1.,1.),(1.,1.),(1.,
1.),(1.,1.),(1.,1.),(1.,1.),(1.,1.),(1.,1.),(1.,1.),(1.,1.),(1.,1.),(1.,
1.),(1.,1.),(1.,1.),(1.,1.),(1.,1.),(1.,1.),(1.,1.),(1.,1.),(1.,1.),(1.,
1.),(1.,1.),(1.,1.),(1.,1.),(1.,1.),(1.,1.),(1.,1.),(1.,1.),(1.,1.),(1.,
1.),(1.,1.),(1.,1.),(1.,1.),(1.,1.),(1.,1.),(1.,1.),(1.,1.),(1.,1.),(1.,
1.),(1.,1.)))
REPRESENTATION_ITEM('')
SURFACE()
);
#45=(
BOUNDED_SURFACE()
B_SPLINE_SURFACE(5,1,((#33124,#33125),(#33126,#33127),(#33128,#33129),(#33130,
#33131),(#33132,#33133),(#33134,#33135),(#33136,#33137),(#33138,#33139),
(#33140,#33141),(#33142,#33143),(#33144,#33145),(#33146,#33147),(#33148,
#33149),(#33150,#33151),(#33152,#33153),(#33154,#33155),(#33156,#33157),
(#33158,#33159),(#33160,#33161),(#33162,#33163),(#33164,#33165),(#33166,
#33167),(#33168,#33169),(#33170,#33171),(#33172,#33173),(#33174,#33175),
(#33176,#33177),(#33178,#33179),(#33180,#33181),(#33182,#33183),(#33184,
#33185),(#33186,#33187),(#33188,#33189),(#33190,#33191),(#33192,#33193),
(#33194,#33195),(#33196,#33197),(#33198,#33199),(#33200,#33201),(#33202,
#33203),(#33204,#33205),(#33206,#33207),(#33208,#33209),(#33210,#33211),
(#33212,#33213),(#33214,#33215),(#33216,#33217),(#33218,#33219),(#33220,
#33221),(#33222,#33223),(#33224,#33225),(#33226,#33227),(#33228,#33229),
(#33230,#33231),(#33232,#33233),(#33234,#33235),(#33236,#33237),(#33238,
#33239),(#33240,#33241),(#33242,#33243),(#33244,#33245),(#33246,#33247),
(#33248,#33249),(#33250,#33251),(#33252,#33253),(#33254,#33255),(#33256,
#33257),(#33258,#33259),(#33260,#33261),(#33262,#33263)),.UNSPECIFIED.,
 .F.,.F.,.F.)
B_SPLINE_SURFACE_WITH_KNOTS((6,1,1,1,1,1,1,1,1,1,1,1,1,1,1,1,1,1,1,1,1,
1,1,1,1,1,1,1,1,1,1,1,1,1,1,1,1,1,1,1,1,1,1,1,1,1,1,1,1,1,1,1,1,1,1,1,1,
1,1,1,1,1,1,1,1,6),(2,2),(-1.,-0.984615384615383,-0.969230769230768,-0.953846153846152,
-0.938461538461537,-0.923076923076922,-0.907692307692306,-0.892307692307691,
-0.876923076923076,-0.86153846153846,-0.846153846153845,-0.83076923076923,
-0.815384615384614,-0.799999999999999,-0.784615384615384,-0.769230769230768,
-0.753846153846153,-0.738461538461538,-0.723076923076922,-0.707692307692307,
-0.692307692307692,-0.676923076923076,-0.661538461538461,-0.646153846153846,
-0.63076923076923,-0.615384615384615,-0.6,-0.584615384615384,-0.569230769230769,
-0.553846153846154,-0.538461538461538,-0.523076923076923,-0.507692307692308,
-0.492307692307692,-0.476923076923077,-0.461538461538462,-0.446153846153846,
-0.430769230769231,-0.415384615384615,-0.4,-0.384615384615385,-0.369230769230769,
-0.353846153846154,-0.338461538461538,-0.323076923076923,-0.307692307692308,
-0.292307692307692,-0.276923076923077,-0.261538461538462,-0.246153846153846,
-0.230769230769231,-0.215384615384615,-0.2,-0.184615384615385,-0.169230769230769,
-0.153846153846154,-0.138461538461538,-0.123076923076923,-0.107692307692308,
-0.0923076923076923,-0.0769230769230769,-0.0615384615384615,-0.0461538461538462,
-0.0307692307692308,-0.0153846153846154,0.),(-1.,1.),.UNSPECIFIED.)
GEOMETRIC_REPRESENTATION_ITEM()
RATIONAL_B_SPLINE_SURFACE(((1.,1.),(1.,1.),(1.,1.),(1.,1.),(1.,1.),(1.,
1.),(1.,1.),(1.,1.),(1.,1.),(1.,1.),(1.,1.),(1.,1.),(1.,1.),(1.,1.),(1.,
1.),(1.,1.),(1.,1.),(1.,1.),(1.,1.),(1.,1.),(1.,1.),(1.,1.),(1.,1.),(1.,
1.),(1.,1.),(1.,1.),(1.,1.),(1.,1.),(1.,1.),(1.,1.),(1.,1.),(1.,1.),(1.,
1.),(1.,1.),(1.,1.),(1.,1.),(1.,1.),(1.,1.),(1.,1.),(1.,1.),(1.,1.),(1.,
1.),(1.,1.),(1.,1.),(1.,1.),(1.,1.),(1.,1.),(1.,1.),(1.,1.),(1.,1.),(1.,
1.),(1.,1.),(1.,1.),(1.,1.),(1.,1.),(1.,1.),(1.,1.),(1.,1.),(1.,1.),(1.,
1.),(1.,1.),(1.,1.),(1.,1.),(1.,1.),(1.,1.),(1.,1.),(1.,1.),(1.,1.),(1.,
1.),(1.,1.)))
REPRESENTATION_ITEM('')
SURFACE()
);
#46=(
BOUNDED_SURFACE()
B_SPLINE_SURFACE(5,1,((#33340,#33341),(#33342,#33343),(#33344,#33345),(#33346,
#33347),(#33348,#33349),(#33350,#33351),(#33352,#33353),(#33354,#33355),
(#33356,#33357),(#33358,#33359),(#33360,#33361),(#33362,#33363),(#33364,
#33365),(#33366,#33367),(#33368,#33369),(#33370,#33371),(#33372,#33373),
(#33374,#33375),(#33376,#33377),(#33378,#33379),(#33380,#33381),(#33382,
#33383),(#33384,#33385),(#33386,#33387),(#33388,#33389),(#33390,#33391),
(#33392,#33393),(#33394,#33395),(#33396,#33397),(#33398,#33399),(#33400,
#33401),(#33402,#33403),(#33404,#33405),(#33406,#33407),(#33408,#33409),
(#33410,#33411),(#33412,#33413),(#33414,#33415),(#33416,#33417),(#33418,
#33419),(#33420,#33421),(#33422,#33423),(#33424,#33425),(#33426,#33427),
(#33428,#33429),(#33430,#33431),(#33432,#33433),(#33434,#33435),(#33436,
#33437),(#33438,#33439),(#33440,#33441),(#33442,#33443),(#33444,#33445),
(#33446,#33447),(#33448,#33449),(#33450,#33451),(#33452,#33453),(#33454,
#33455),(#33456,#33457),(#33458,#33459),(#33460,#33461),(#33462,#33463),
(#33464,#33465),(#33466,#33467),(#33468,#33469),(#33470,#33471),(#33472,
#33473),(#33474,#33475),(#33476,#33477),(#33478,#33479)),.UNSPECIFIED.,
 .F.,.F.,.F.)
B_SPLINE_SURFACE_WITH_KNOTS((6,1,1,1,1,1,1,1,1,1,1,1,1,1,1,1,1,1,1,1,1,
1,1,1,1,1,1,1,1,1,1,1,1,1,1,1,1,1,1,1,1,1,1,1,1,1,1,1,1,1,1,1,1,1,1,1,1,
1,1,1,1,1,1,1,1,6),(2,2),(-1.,-0.984615384615383,-0.969230769230768,-0.953846153846152,
-0.938461538461537,-0.923076923076922,-0.907692307692306,-0.892307692307691,
-0.876923076923076,-0.86153846153846,-0.846153846153845,-0.83076923076923,
-0.815384615384614,-0.799999999999999,-0.784615384615384,-0.769230769230768,
-0.753846153846153,-0.738461538461538,-0.723076923076922,-0.707692307692307,
-0.692307692307692,-0.676923076923076,-0.661538461538461,-0.646153846153846,
-0.63076923076923,-0.615384615384615,-0.6,-0.584615384615384,-0.569230769230769,
-0.553846153846154,-0.538461538461538,-0.523076923076923,-0.507692307692308,
-0.492307692307692,-0.476923076923077,-0.461538461538462,-0.446153846153846,
-0.430769230769231,-0.415384615384615,-0.4,-0.384615384615385,-0.369230769230769,
-0.353846153846154,-0.338461538461538,-0.323076923076923,-0.307692307692308,
-0.292307692307692,-0.276923076923077,-0.261538461538462,-0.246153846153846,
-0.230769230769231,-0.215384615384615,-0.2,-0.184615384615385,-0.169230769230769,
-0.153846153846154,-0.138461538461538,-0.123076923076923,-0.107692307692308,
-0.0923076923076923,-0.0769230769230769,-0.0615384615384615,-0.0461538461538462,
-0.0307692307692308,-0.0153846153846154,0.),(-1.,1.),.UNSPECIFIED.)
GEOMETRIC_REPRESENTATION_ITEM()
RATIONAL_B_SPLINE_SURFACE(((1.,1.),(1.,1.),(1.,1.),(1.,1.),(1.,1.),(1.,
1.),(1.,1.),(1.,1.),(1.,1.),(1.,1.),(1.,1.),(1.,1.),(1.,1.),(1.,1.),(1.,
1.),(1.,1.),(1.,1.),(1.,1.),(1.,1.),(1.,1.),(1.,1.),(1.,1.),(1.,1.),(1.,
1.),(1.,1.),(1.,1.),(1.,1.),(1.,1.),(1.,1.),(1.,1.),(1.,1.),(1.,1.),(1.,
1.),(1.,1.),(1.,1.),(1.,1.),(1.,1.),(1.,1.),(1.,1.),(1.,1.),(1.,1.),(1.,
1.),(1.,1.),(1.,1.),(1.,1.),(1.,1.),(1.,1.),(1.,1.),(1.,1.),(1.,1.),(1.,
1.),(1.,1.),(1.,1.),(1.,1.),(1.,1.),(1.,1.),(1.,1.),(1.,1.),(1.,1.),(1.,
1.),(1.,1.),(1.,1.),(1.,1.),(1.,1.),(1.,1.),(1.,1.),(1.,1.),(1.,1.),(1.,
1.),(1.,1.)))
REPRESENTATION_ITEM('')
SURFACE()
);
#47=(
BOUNDED_SURFACE()
B_SPLINE_SURFACE(5,1,((#33556,#33557),(#33558,#33559),(#33560,#33561),(#33562,
#33563),(#33564,#33565),(#33566,#33567),(#33568,#33569),(#33570,#33571),
(#33572,#33573),(#33574,#33575),(#33576,#33577),(#33578,#33579),(#33580,
#33581),(#33582,#33583),(#33584,#33585),(#33586,#33587),(#33588,#33589),
(#33590,#33591),(#33592,#33593),(#33594,#33595),(#33596,#33597),(#33598,
#33599),(#33600,#33601),(#33602,#33603),(#33604,#33605),(#33606,#33607),
(#33608,#33609),(#33610,#33611),(#33612,#33613),(#33614,#33615),(#33616,
#33617),(#33618,#33619),(#33620,#33621),(#33622,#33623),(#33624,#33625),
(#33626,#33627),(#33628,#33629),(#33630,#33631),(#33632,#33633),(#33634,
#33635),(#33636,#33637),(#33638,#33639),(#33640,#33641),(#33642,#33643),
(#33644,#33645),(#33646,#33647),(#33648,#33649),(#33650,#33651),(#33652,
#33653),(#33654,#33655),(#33656,#33657),(#33658,#33659),(#33660,#33661),
(#33662,#33663),(#33664,#33665),(#33666,#33667),(#33668,#33669),(#33670,
#33671),(#33672,#33673),(#33674,#33675),(#33676,#33677),(#33678,#33679),
(#33680,#33681),(#33682,#33683),(#33684,#33685),(#33686,#33687),(#33688,
#33689),(#33690,#33691),(#33692,#33693),(#33694,#33695)),.UNSPECIFIED.,
 .F.,.F.,.F.)
B_SPLINE_SURFACE_WITH_KNOTS((6,1,1,1,1,1,1,1,1,1,1,1,1,1,1,1,1,1,1,1,1,
1,1,1,1,1,1,1,1,1,1,1,1,1,1,1,1,1,1,1,1,1,1,1,1,1,1,1,1,1,1,1,1,1,1,1,1,
1,1,1,1,1,1,1,1,6),(2,2),(-1.,-0.984615384615383,-0.969230769230768,-0.953846153846152,
-0.938461538461537,-0.923076923076922,-0.907692307692306,-0.892307692307691,
-0.876923076923076,-0.86153846153846,-0.846153846153845,-0.83076923076923,
-0.815384615384614,-0.799999999999999,-0.784615384615384,-0.769230769230768,
-0.753846153846153,-0.738461538461538,-0.723076923076922,-0.707692307692307,
-0.692307692307692,-0.676923076923076,-0.661538461538461,-0.646153846153846,
-0.63076923076923,-0.615384615384615,-0.6,-0.584615384615384,-0.569230769230769,
-0.553846153846154,-0.538461538461538,-0.523076923076923,-0.507692307692308,
-0.492307692307692,-0.476923076923077,-0.461538461538462,-0.446153846153846,
-0.430769230769231,-0.415384615384615,-0.4,-0.384615384615385,-0.369230769230769,
-0.353846153846154,-0.338461538461538,-0.323076923076923,-0.307692307692308,
-0.292307692307692,-0.276923076923077,-0.261538461538462,-0.246153846153846,
-0.230769230769231,-0.215384615384615,-0.2,-0.184615384615385,-0.169230769230769,
-0.153846153846154,-0.138461538461538,-0.123076923076923,-0.107692307692308,
-0.0923076923076923,-0.0769230769230769,-0.0615384615384615,-0.0461538461538462,
-0.0307692307692308,-0.0153846153846154,0.),(-1.,1.),.UNSPECIFIED.)
GEOMETRIC_REPRESENTATION_ITEM()
RATIONAL_B_SPLINE_SURFACE(((1.,1.),(1.,1.),(1.,1.),(1.,1.),(1.,1.),(1.,
1.),(1.,1.),(1.,1.),(1.,1.),(1.,1.),(1.,1.),(1.,1.),(1.,1.),(1.,1.),(1.,
1.),(1.,1.),(1.,1.),(1.,1.),(1.,1.),(1.,1.),(1.,1.),(1.,1.),(1.,1.),(1.,
1.),(1.,1.),(1.,1.),(1.,1.),(1.,1.),(1.,1.),(1.,1.),(1.,1.),(1.,1.),(1.,
1.),(1.,1.),(1.,1.),(1.,1.),(1.,1.),(1.,1.),(1.,1.),(1.,1.),(1.,1.),(1.,
1.),(1.,1.),(1.,1.),(1.,1.),(1.,1.),(1.,1.),(1.,1.),(1.,1.),(1.,1.),(1.,
1.),(1.,1.),(1.,1.),(1.,1.),(1.,1.),(1.,1.),(1.,1.),(1.,1.),(1.,1.),(1.,
1.),(1.,1.),(1.,1.),(1.,1.),(1.,1.),(1.,1.),(1.,1.),(1.,1.),(1.,1.),(1.,
1.),(1.,1.)))
REPRESENTATION_ITEM('')
SURFACE()
);
#48=(
BOUNDED_SURFACE()
B_SPLINE_SURFACE(5,1,((#33772,#33773),(#33774,#33775),(#33776,#33777),(#33778,
#33779),(#33780,#33781),(#33782,#33783),(#33784,#33785),(#33786,#33787),
(#33788,#33789),(#33790,#33791),(#33792,#33793),(#33794,#33795),(#33796,
#33797),(#33798,#33799),(#33800,#33801),(#33802,#33803),(#33804,#33805),
(#33806,#33807),(#33808,#33809),(#33810,#33811),(#33812,#33813),(#33814,
#33815),(#33816,#33817),(#33818,#33819),(#33820,#33821),(#33822,#33823),
(#33824,#33825),(#33826,#33827),(#33828,#33829),(#33830,#33831),(#33832,
#33833),(#33834,#33835),(#33836,#33837),(#33838,#33839),(#33840,#33841),
(#33842,#33843),(#33844,#33845),(#33846,#33847),(#33848,#33849),(#33850,
#33851),(#33852,#33853),(#33854,#33855),(#33856,#33857),(#33858,#33859),
(#33860,#33861),(#33862,#33863),(#33864,#33865),(#33866,#33867),(#33868,
#33869),(#33870,#33871),(#33872,#33873),(#33874,#33875),(#33876,#33877),
(#33878,#33879),(#33880,#33881),(#33882,#33883),(#33884,#33885),(#33886,
#33887),(#33888,#33889),(#33890,#33891),(#33892,#33893),(#33894,#33895),
(#33896,#33897),(#33898,#33899),(#33900,#33901),(#33902,#33903),(#33904,
#33905),(#33906,#33907),(#33908,#33909),(#33910,#33911)),.UNSPECIFIED.,
 .F.,.F.,.F.)
B_SPLINE_SURFACE_WITH_KNOTS((6,1,1,1,1,1,1,1,1,1,1,1,1,1,1,1,1,1,1,1,1,
1,1,1,1,1,1,1,1,1,1,1,1,1,1,1,1,1,1,1,1,1,1,1,1,1,1,1,1,1,1,1,1,1,1,1,1,
1,1,1,1,1,1,1,1,6),(2,2),(-1.,-0.984615384615383,-0.969230769230768,-0.953846153846152,
-0.938461538461537,-0.923076923076922,-0.907692307692306,-0.892307692307691,
-0.876923076923076,-0.86153846153846,-0.846153846153845,-0.83076923076923,
-0.815384615384614,-0.799999999999999,-0.784615384615384,-0.769230769230768,
-0.753846153846153,-0.738461538461538,-0.723076923076922,-0.707692307692307,
-0.692307692307692,-0.676923076923076,-0.661538461538461,-0.646153846153846,
-0.63076923076923,-0.615384615384615,-0.6,-0.584615384615384,-0.569230769230769,
-0.553846153846154,-0.538461538461538,-0.523076923076923,-0.507692307692308,
-0.492307692307692,-0.476923076923077,-0.461538461538462,-0.446153846153846,
-0.430769230769231,-0.415384615384615,-0.4,-0.384615384615385,-0.369230769230769,
-0.353846153846154,-0.338461538461538,-0.323076923076923,-0.307692307692308,
-0.292307692307692,-0.276923076923077,-0.261538461538462,-0.246153846153846,
-0.230769230769231,-0.215384615384615,-0.2,-0.184615384615385,-0.169230769230769,
-0.153846153846154,-0.138461538461538,-0.123076923076923,-0.107692307692308,
-0.0923076923076923,-0.0769230769230769,-0.0615384615384615,-0.0461538461538462,
-0.0307692307692308,-0.0153846153846154,0.),(-1.,1.),.UNSPECIFIED.)
GEOMETRIC_REPRESENTATION_ITEM()
RATIONAL_B_SPLINE_SURFACE(((1.,1.),(1.,1.),(1.,1.),(1.,1.),(1.,1.),(1.,
1.),(1.,1.),(1.,1.),(1.,1.),(1.,1.),(1.,1.),(1.,1.),(1.,1.),(1.,1.),(1.,
1.),(1.,1.),(1.,1.),(1.,1.),(1.,1.),(1.,1.),(1.,1.),(1.,1.),(1.,1.),(1.,
1.),(1.,1.),(1.,1.),(1.,1.),(1.,1.),(1.,1.),(1.,1.),(1.,1.),(1.,1.),(1.,
1.),(1.,1.),(1.,1.),(1.,1.),(1.,1.),(1.,1.),(1.,1.),(1.,1.),(1.,1.),(1.,
1.),(1.,1.),(1.,1.),(1.,1.),(1.,1.),(1.,1.),(1.,1.),(1.,1.),(1.,1.),(1.,
1.),(1.,1.),(1.,1.),(1.,1.),(1.,1.),(1.,1.),(1.,1.),(1.,1.),(1.,1.),(1.,
1.),(1.,1.),(1.,1.),(1.,1.),(1.,1.),(1.,1.),(1.,1.),(1.,1.),(1.,1.),(1.,
1.),(1.,1.)))
REPRESENTATION_ITEM('')
SURFACE()
);
#49=(
BOUNDED_SURFACE()
B_SPLINE_SURFACE(5,1,((#33988,#33989),(#33990,#33991),(#33992,#33993),(#33994,
#33995),(#33996,#33997),(#33998,#33999),(#34000,#34001),(#34002,#34003),
(#34004,#34005),(#34006,#34007),(#34008,#34009),(#34010,#34011),(#34012,
#34013),(#34014,#34015),(#34016,#34017),(#34018,#34019),(#34020,#34021),
(#34022,#34023),(#34024,#34025),(#34026,#34027),(#34028,#34029),(#34030,
#34031),(#34032,#34033),(#34034,#34035),(#34036,#34037),(#34038,#34039),
(#34040,#34041),(#34042,#34043),(#34044,#34045),(#34046,#34047),(#34048,
#34049),(#34050,#34051),(#34052,#34053),(#34054,#34055),(#34056,#34057),
(#34058,#34059),(#34060,#34061),(#34062,#34063),(#34064,#34065),(#34066,
#34067),(#34068,#34069),(#34070,#34071),(#34072,#34073),(#34074,#34075),
(#34076,#34077),(#34078,#34079),(#34080,#34081),(#34082,#34083),(#34084,
#34085),(#34086,#34087),(#34088,#34089),(#34090,#34091),(#34092,#34093),
(#34094,#34095),(#34096,#34097),(#34098,#34099),(#34100,#34101),(#34102,
#34103),(#34104,#34105),(#34106,#34107),(#34108,#34109),(#34110,#34111),
(#34112,#34113),(#34114,#34115),(#34116,#34117),(#34118,#34119),(#34120,
#34121),(#34122,#34123),(#34124,#34125),(#34126,#34127)),.UNSPECIFIED.,
 .F.,.F.,.F.)
B_SPLINE_SURFACE_WITH_KNOTS((6,1,1,1,1,1,1,1,1,1,1,1,1,1,1,1,1,1,1,1,1,
1,1,1,1,1,1,1,1,1,1,1,1,1,1,1,1,1,1,1,1,1,1,1,1,1,1,1,1,1,1,1,1,1,1,1,1,
1,1,1,1,1,1,1,1,6),(2,2),(-1.,-0.984615384615383,-0.969230769230768,-0.953846153846152,
-0.938461538461537,-0.923076923076922,-0.907692307692306,-0.892307692307691,
-0.876923076923076,-0.86153846153846,-0.846153846153845,-0.83076923076923,
-0.815384615384614,-0.799999999999999,-0.784615384615384,-0.769230769230768,
-0.753846153846153,-0.738461538461538,-0.723076923076922,-0.707692307692307,
-0.692307692307692,-0.676923076923076,-0.661538461538461,-0.646153846153846,
-0.63076923076923,-0.615384615384615,-0.6,-0.584615384615384,-0.569230769230769,
-0.553846153846154,-0.538461538461538,-0.523076923076923,-0.507692307692308,
-0.492307692307692,-0.476923076923077,-0.461538461538462,-0.446153846153846,
-0.430769230769231,-0.415384615384615,-0.4,-0.384615384615385,-0.369230769230769,
-0.353846153846154,-0.338461538461538,-0.323076923076923,-0.307692307692308,
-0.292307692307692,-0.276923076923077,-0.261538461538462,-0.246153846153846,
-0.230769230769231,-0.215384615384615,-0.2,-0.184615384615385,-0.169230769230769,
-0.153846153846154,-0.138461538461538,-0.123076923076923,-0.107692307692308,
-0.0923076923076923,-0.0769230769230769,-0.0615384615384615,-0.0461538461538462,
-0.0307692307692308,-0.0153846153846154,0.),(-1.,1.),.UNSPECIFIED.)
GEOMETRIC_REPRESENTATION_ITEM()
RATIONAL_B_SPLINE_SURFACE(((1.,1.),(1.,1.),(1.,1.),(1.,1.),(1.,1.),(1.,
1.),(1.,1.),(1.,1.),(1.,1.),(1.,1.),(1.,1.),(1.,1.),(1.,1.),(1.,1.),(1.,
1.),(1.,1.),(1.,1.),(1.,1.),(1.,1.),(1.,1.),(1.,1.),(1.,1.),(1.,1.),(1.,
1.),(1.,1.),(1.,1.),(1.,1.),(1.,1.),(1.,1.),(1.,1.),(1.,1.),(1.,1.),(1.,
1.),(1.,1.),(1.,1.),(1.,1.),(1.,1.),(1.,1.),(1.,1.),(1.,1.),(1.,1.),(1.,
1.),(1.,1.),(1.,1.),(1.,1.),(1.,1.),(1.,1.),(1.,1.),(1.,1.),(1.,1.),(1.,
1.),(1.,1.),(1.,1.),(1.,1.),(1.,1.),(1.,1.),(1.,1.),(1.,1.),(1.,1.),(1.,
1.),(1.,1.),(1.,1.),(1.,1.),(1.,1.),(1.,1.),(1.,1.),(1.,1.),(1.,1.),(1.,
1.),(1.,1.)))
REPRESENTATION_ITEM('')
SURFACE()
);
#50=(
BOUNDED_SURFACE()
B_SPLINE_SURFACE(5,1,((#34204,#34205),(#34206,#34207),(#34208,#34209),(#34210,
#34211),(#34212,#34213),(#34214,#34215),(#34216,#34217),(#34218,#34219),
(#34220,#34221),(#34222,#34223),(#34224,#34225),(#34226,#34227),(#34228,
#34229),(#34230,#34231),(#34232,#34233),(#34234,#34235),(#34236,#34237),
(#34238,#34239),(#34240,#34241),(#34242,#34243),(#34244,#34245),(#34246,
#34247),(#34248,#34249),(#34250,#34251),(#34252,#34253),(#34254,#34255),
(#34256,#34257),(#34258,#34259),(#34260,#34261),(#34262,#34263),(#34264,
#34265),(#34266,#34267),(#34268,#34269),(#34270,#34271),(#34272,#34273),
(#34274,#34275),(#34276,#34277),(#34278,#34279),(#34280,#34281),(#34282,
#34283),(#34284,#34285),(#34286,#34287),(#34288,#34289),(#34290,#34291),
(#34292,#34293),(#34294,#34295),(#34296,#34297),(#34298,#34299),(#34300,
#34301),(#34302,#34303),(#34304,#34305),(#34306,#34307),(#34308,#34309),
(#34310,#34311),(#34312,#34313),(#34314,#34315),(#34316,#34317),(#34318,
#34319),(#34320,#34321),(#34322,#34323),(#34324,#34325),(#34326,#34327),
(#34328,#34329),(#34330,#34331),(#34332,#34333),(#34334,#34335),(#34336,
#34337),(#34338,#34339),(#34340,#34341),(#34342,#34343)),.UNSPECIFIED.,
 .F.,.F.,.F.)
B_SPLINE_SURFACE_WITH_KNOTS((6,1,1,1,1,1,1,1,1,1,1,1,1,1,1,1,1,1,1,1,1,
1,1,1,1,1,1,1,1,1,1,1,1,1,1,1,1,1,1,1,1,1,1,1,1,1,1,1,1,1,1,1,1,1,1,1,1,
1,1,1,1,1,1,1,1,6),(2,2),(-1.,-0.984615384615383,-0.969230769230768,-0.953846153846152,
-0.938461538461537,-0.923076923076922,-0.907692307692306,-0.892307692307691,
-0.876923076923076,-0.86153846153846,-0.846153846153845,-0.83076923076923,
-0.815384615384614,-0.799999999999999,-0.784615384615384,-0.769230769230768,
-0.753846153846153,-0.738461538461538,-0.723076923076922,-0.707692307692307,
-0.692307692307692,-0.676923076923076,-0.661538461538461,-0.646153846153846,
-0.63076923076923,-0.615384615384615,-0.6,-0.584615384615384,-0.569230769230769,
-0.553846153846154,-0.538461538461538,-0.523076923076923,-0.507692307692308,
-0.492307692307692,-0.476923076923077,-0.461538461538462,-0.446153846153846,
-0.430769230769231,-0.415384615384615,-0.4,-0.384615384615385,-0.369230769230769,
-0.353846153846154,-0.338461538461538,-0.323076923076923,-0.307692307692308,
-0.292307692307692,-0.276923076923077,-0.261538461538462,-0.246153846153846,
-0.230769230769231,-0.215384615384615,-0.2,-0.184615384615385,-0.169230769230769,
-0.153846153846154,-0.138461538461538,-0.123076923076923,-0.107692307692308,
-0.0923076923076923,-0.0769230769230769,-0.0615384615384615,-0.0461538461538462,
-0.0307692307692308,-0.0153846153846154,0.),(-1.,1.),.UNSPECIFIED.)
GEOMETRIC_REPRESENTATION_ITEM()
RATIONAL_B_SPLINE_SURFACE(((1.,1.),(1.,1.),(1.,1.),(1.,1.),(1.,1.),(1.,
1.),(1.,1.),(1.,1.),(1.,1.),(1.,1.),(1.,1.),(1.,1.),(1.,1.),(1.,1.),(1.,
1.),(1.,1.),(1.,1.),(1.,1.),(1.,1.),(1.,1.),(1.,1.),(1.,1.),(1.,1.),(1.,
1.),(1.,1.),(1.,1.),(1.,1.),(1.,1.),(1.,1.),(1.,1.),(1.,1.),(1.,1.),(1.,
1.),(1.,1.),(1.,1.),(1.,1.),(1.,1.),(1.,1.),(1.,1.),(1.,1.),(1.,1.),(1.,
1.),(1.,1.),(1.,1.),(1.,1.),(1.,1.),(1.,1.),(1.,1.),(1.,1.),(1.,1.),(1.,
1.),(1.,1.),(1.,1.),(1.,1.),(1.,1.),(1.,1.),(1.,1.),(1.,1.),(1.,1.),(1.,
1.),(1.,1.),(1.,1.),(1.,1.),(1.,1.),(1.,1.),(1.,1.),(1.,1.),(1.,1.),(1.,
1.),(1.,1.)))
REPRESENTATION_ITEM('')
SURFACE()
);
#51=(
BOUNDED_CURVE()
B_SPLINE_CURVE(5,(#22852,#22853,#22854,#22855,#22856,#22857,#22858,#22859,
#22860,#22861,#22862,#22863,#22864,#22865,#22866,#22867,#22868,#22869,#22870,
#22871,#22872,#22873,#22874,#22875,#22876,#22877,#22878,#22879,#22880,#22881,
#22882,#22883,#22884,#22885,#22886,#22887,#22888,#22889,#22890,#22891,#22892,
#22893,#22894,#22895,#22896,#22897,#22898,#22899,#22900,#22901,#22902,#22903,
#22904,#22905,#22906,#22907,#22908,#22909,#22910,#22911,#22912,#22913,#22914,
#22915,#22916,#22917,#22918,#22919,#22920,#22921),.UNSPECIFIED.,.F.,.F.)
B_SPLINE_CURVE_WITH_KNOTS((6,1,1,1,1,1,1,1,1,1,1,1,1,1,1,1,1,1,1,1,1,1,
1,1,1,1,1,1,1,1,1,1,1,1,1,1,1,1,1,1,1,1,1,1,1,1,1,1,1,1,1,1,1,1,1,1,1,1,
1,1,1,1,1,1,1,6),(0.,0.0153846153846154,0.0307692307692308,0.0461538461538462,
0.0615384615384615,0.0769230769230769,0.0923076923076923,0.107692307692308,
0.123076923076923,0.138461538461538,0.153846153846154,0.169230769230769,
0.184615384615385,0.2,0.215384615384615,0.230769230769231,0.246153846153846,
0.261538461538462,0.276923076923077,0.292307692307692,0.307692307692308,
0.323076923076923,0.338461538461538,0.353846153846154,0.369230769230769,
0.384615384615385,0.4,0.415384615384615,0.430769230769231,0.446153846153846,
0.461538461538462,0.476923076923077,0.492307692307692,0.507692307692308,
0.523076923076923,0.538461538461538,0.553846153846154,0.569230769230769,
0.584615384615384,0.6,0.615384615384615,0.63076923076923,0.646153846153846,
0.661538461538461,0.676923076923076,0.692307692307692,0.707692307692307,
0.723076923076922,0.738461538461538,0.753846153846153,0.769230769230768,
0.784615384615384,0.799999999999999,0.815384615384614,0.83076923076923,
0.846153846153845,0.86153846153846,0.876923076923076,0.892307692307691,
0.907692307692306,0.923076923076922,0.938461538461537,0.953846153846152,
0.969230769230768,0.984615384615383,1.),.UNSPECIFIED.)
CURVE()
GEOMETRIC_REPRESENTATION_ITEM()
RATIONAL_B_SPLINE_CURVE((1.,1.,1.,1.,1.,1.,1.,1.,1.,1.,1.,1.,1.,1.,1.,1.,
1.,1.,1.,1.,1.,1.,1.,1.,1.,1.,1.,1.,1.,1.,1.,1.,1.,1.,1.,1.,1.,1.,1.,1.,
1.,1.,1.,1.,1.,1.,1.,1.,1.,1.,1.,1.,1.,1.,1.,1.,1.,1.,1.,1.,1.,1.,1.,1.,
1.,1.,1.,1.,1.,1.))
REPRESENTATION_ITEM('')
);
#52=(
BOUNDED_CURVE()
B_SPLINE_CURVE(5,(#22925,#22926,#22927,#22928,#22929,#22930,#22931,#22932,
#22933,#22934,#22935,#22936,#22937,#22938,#22939,#22940,#22941,#22942,#22943,
#22944,#22945,#22946,#22947,#22948,#22949,#22950,#22951,#22952,#22953,#22954,
#22955,#22956,#22957,#22958,#22959,#22960,#22961,#22962,#22963,#22964,#22965,
#22966,#22967,#22968,#22969,#22970,#22971,#22972,#22973,#22974,#22975,#22976,
#22977,#22978,#22979,#22980,#22981,#22982,#22983,#22984,#22985,#22986,#22987,
#22988,#22989,#22990,#22991,#22992,#22993,#22994),.UNSPECIFIED.,.F.,.F.)
B_SPLINE_CURVE_WITH_KNOTS((6,1,1,1,1,1,1,1,1,1,1,1,1,1,1,1,1,1,1,1,1,1,
1,1,1,1,1,1,1,1,1,1,1,1,1,1,1,1,1,1,1,1,1,1,1,1,1,1,1,1,1,1,1,1,1,1,1,1,
1,1,1,1,1,1,1,6),(0.,0.0153846153846154,0.0307692307692308,0.0461538461538462,
0.0615384615384615,0.0769230769230769,0.0923076923076923,0.107692307692308,
0.123076923076923,0.138461538461538,0.153846153846154,0.169230769230769,
0.184615384615385,0.2,0.215384615384615,0.230769230769231,0.246153846153846,
0.261538461538462,0.276923076923077,0.292307692307692,0.307692307692308,
0.323076923076923,0.338461538461538,0.353846153846154,0.369230769230769,
0.384615384615385,0.4,0.415384615384615,0.430769230769231,0.446153846153846,
0.461538461538462,0.476923076923077,0.492307692307692,0.507692307692308,
0.523076923076923,0.538461538461538,0.553846153846154,0.569230769230769,
0.584615384615384,0.6,0.615384615384615,0.63076923076923,0.646153846153846,
0.661538461538461,0.676923076923076,0.692307692307692,0.707692307692307,
0.723076923076922,0.738461538461538,0.753846153846153,0.769230769230768,
0.784615384615384,0.799999999999999,0.815384615384614,0.83076923076923,
0.846153846153845,0.86153846153846,0.876923076923076,0.892307692307691,
0.907692307692306,0.923076923076922,0.938461538461537,0.953846153846152,
0.969230769230768,0.984615384615383,1.),.UNSPECIFIED.)
CURVE()
GEOMETRIC_REPRESENTATION_ITEM()
RATIONAL_B_SPLINE_CURVE((1.,1.,1.,1.,1.,1.,1.,1.,1.,1.,1.,1.,1.,1.,1.,1.,
1.,1.,1.,1.,1.,1.,1.,1.,1.,1.,1.,1.,1.,1.,1.,1.,1.,1.,1.,1.,1.,1.,1.,1.,
1.,1.,1.,1.,1.,1.,1.,1.,1.,1.,1.,1.,1.,1.,1.,1.,1.,1.,1.,1.,1.,1.,1.,1.,
1.,1.,1.,1.,1.,1.))
REPRESENTATION_ITEM('')
);
#53=(
BOUNDED_CURVE()
B_SPLINE_CURVE(5,(#22998,#22999,#23000,#23001,#23002,#23003,#23004,#23005,
#23006,#23007,#23008,#23009,#23010,#23011,#23012,#23013,#23014,#23015,#23016,
#23017,#23018,#23019,#23020,#23021,#23022,#23023,#23024,#23025,#23026,#23027,
#23028,#23029,#23030,#23031,#23032,#23033,#23034,#23035,#23036,#23037,#23038,
#23039,#23040,#23041,#23042,#23043,#23044,#23045,#23046,#23047,#23048,#23049,
#23050,#23051,#23052,#23053,#23054,#23055,#23056,#23057,#23058,#23059,#23060,
#23061,#23062,#23063,#23064,#23065,#23066,#23067),.UNSPECIFIED.,.F.,.F.)
B_SPLINE_CURVE_WITH_KNOTS((6,1,1,1,1,1,1,1,1,1,1,1,1,1,1,1,1,1,1,1,1,1,
1,1,1,1,1,1,1,1,1,1,1,1,1,1,1,1,1,1,1,1,1,1,1,1,1,1,1,1,1,1,1,1,1,1,1,1,
1,1,1,1,1,1,1,6),(0.,0.0153846153846154,0.0307692307692308,0.0461538461538462,
0.0615384615384615,0.0769230769230769,0.0923076923076923,0.107692307692308,
0.123076923076923,0.138461538461538,0.153846153846154,0.169230769230769,
0.184615384615385,0.2,0.215384615384615,0.230769230769231,0.246153846153846,
0.261538461538462,0.276923076923077,0.292307692307692,0.307692307692308,
0.323076923076923,0.338461538461538,0.353846153846154,0.369230769230769,
0.384615384615385,0.4,0.415384615384615,0.430769230769231,0.446153846153846,
0.461538461538462,0.476923076923077,0.492307692307692,0.507692307692308,
0.523076923076923,0.538461538461538,0.553846153846154,0.569230769230769,
0.584615384615384,0.6,0.615384615384615,0.63076923076923,0.646153846153846,
0.661538461538461,0.676923076923076,0.692307692307692,0.707692307692307,
0.723076923076922,0.738461538461538,0.753846153846153,0.769230769230768,
0.784615384615384,0.799999999999999,0.815384615384614,0.83076923076923,
0.846153846153845,0.86153846153846,0.876923076923076,0.892307692307691,
0.907692307692306,0.923076923076922,0.938461538461537,0.953846153846152,
0.969230769230768,0.984615384615383,1.),.UNSPECIFIED.)
CURVE()
GEOMETRIC_REPRESENTATION_ITEM()
RATIONAL_B_SPLINE_CURVE((1.,1.,1.,1.,1.,1.,1.,1.,1.,1.,1.,1.,1.,1.,1.,1.,
1.,1.,1.,1.,1.,1.,1.,1.,1.,1.,1.,1.,1.,1.,1.,1.,1.,1.,1.,1.,1.,1.,1.,1.,
1.,1.,1.,1.,1.,1.,1.,1.,1.,1.,1.,1.,1.,1.,1.,1.,1.,1.,1.,1.,1.,1.,1.,1.,
1.,1.,1.,1.,1.,1.))
REPRESENTATION_ITEM('')
);
#54=(
BOUNDED_CURVE()
B_SPLINE_CURVE(5,(#23071,#23072,#23073,#23074,#23075,#23076,#23077,#23078,
#23079,#23080,#23081,#23082,#23083,#23084,#23085,#23086,#23087,#23088,#23089,
#23090,#23091,#23092,#23093,#23094,#23095,#23096,#23097,#23098,#23099,#23100,
#23101,#23102,#23103,#23104,#23105,#23106,#23107,#23108,#23109,#23110,#23111,
#23112,#23113,#23114,#23115,#23116,#23117,#23118,#23119,#23120,#23121,#23122,
#23123,#23124,#23125,#23126,#23127,#23128,#23129,#23130,#23131,#23132,#23133,
#23134,#23135,#23136,#23137,#23138,#23139,#23140),.UNSPECIFIED.,.F.,.F.)
B_SPLINE_CURVE_WITH_KNOTS((6,1,1,1,1,1,1,1,1,1,1,1,1,1,1,1,1,1,1,1,1,1,
1,1,1,1,1,1,1,1,1,1,1,1,1,1,1,1,1,1,1,1,1,1,1,1,1,1,1,1,1,1,1,1,1,1,1,1,
1,1,1,1,1,1,1,6),(0.,0.0153846153846154,0.0307692307692308,0.0461538461538462,
0.0615384615384615,0.0769230769230769,0.0923076923076923,0.107692307692308,
0.123076923076923,0.138461538461538,0.153846153846154,0.169230769230769,
0.184615384615385,0.2,0.215384615384615,0.230769230769231,0.246153846153846,
0.261538461538462,0.276923076923077,0.292307692307692,0.307692307692308,
0.323076923076923,0.338461538461538,0.353846153846154,0.369230769230769,
0.384615384615385,0.4,0.415384615384615,0.430769230769231,0.446153846153846,
0.461538461538462,0.476923076923077,0.492307692307692,0.507692307692308,
0.523076923076923,0.538461538461538,0.553846153846154,0.569230769230769,
0.584615384615384,0.6,0.615384615384615,0.63076923076923,0.646153846153846,
0.661538461538461,0.676923076923076,0.692307692307692,0.707692307692307,
0.723076923076922,0.738461538461538,0.753846153846153,0.769230769230768,
0.784615384615384,0.799999999999999,0.815384615384614,0.83076923076923,
0.846153846153845,0.86153846153846,0.876923076923076,0.892307692307691,
0.907692307692306,0.923076923076922,0.938461538461537,0.953846153846152,
0.969230769230768,0.984615384615383,1.),.UNSPECIFIED.)
CURVE()
GEOMETRIC_REPRESENTATION_ITEM()
RATIONAL_B_SPLINE_CURVE((1.,1.,1.,1.,1.,1.,1.,1.,1.,1.,1.,1.,1.,1.,1.,1.,
1.,1.,1.,1.,1.,1.,1.,1.,1.,1.,1.,1.,1.,1.,1.,1.,1.,1.,1.,1.,1.,1.,1.,1.,
1.,1.,1.,1.,1.,1.,1.,1.,1.,1.,1.,1.,1.,1.,1.,1.,1.,1.,1.,1.,1.,1.,1.,1.,
1.,1.,1.,1.,1.,1.))
REPRESENTATION_ITEM('')
);
#55=(
BOUNDED_CURVE()
B_SPLINE_CURVE(5,(#23144,#23145,#23146,#23147,#23148,#23149,#23150,#23151,
#23152,#23153,#23154,#23155,#23156,#23157,#23158,#23159,#23160,#23161,#23162,
#23163,#23164,#23165,#23166,#23167,#23168,#23169,#23170,#23171,#23172,#23173,
#23174,#23175,#23176,#23177,#23178,#23179,#23180,#23181,#23182,#23183,#23184,
#23185,#23186,#23187,#23188,#23189,#23190,#23191,#23192,#23193,#23194,#23195,
#23196,#23197,#23198,#23199,#23200,#23201,#23202,#23203,#23204,#23205,#23206,
#23207,#23208,#23209,#23210,#23211,#23212,#23213),.UNSPECIFIED.,.F.,.F.)
B_SPLINE_CURVE_WITH_KNOTS((6,1,1,1,1,1,1,1,1,1,1,1,1,1,1,1,1,1,1,1,1,1,
1,1,1,1,1,1,1,1,1,1,1,1,1,1,1,1,1,1,1,1,1,1,1,1,1,1,1,1,1,1,1,1,1,1,1,1,
1,1,1,1,1,1,1,6),(0.,0.0153846153846154,0.0307692307692308,0.0461538461538462,
0.0615384615384615,0.0769230769230769,0.0923076923076923,0.107692307692308,
0.123076923076923,0.138461538461538,0.153846153846154,0.169230769230769,
0.184615384615385,0.2,0.215384615384615,0.230769230769231,0.246153846153846,
0.261538461538462,0.276923076923077,0.292307692307692,0.307692307692308,
0.323076923076923,0.338461538461538,0.353846153846154,0.369230769230769,
0.384615384615385,0.4,0.415384615384615,0.430769230769231,0.446153846153846,
0.461538461538462,0.476923076923077,0.492307692307692,0.507692307692308,
0.523076923076923,0.538461538461538,0.553846153846154,0.569230769230769,
0.584615384615384,0.6,0.615384615384615,0.63076923076923,0.646153846153846,
0.661538461538461,0.676923076923076,0.692307692307692,0.707692307692307,
0.723076923076922,0.738461538461538,0.753846153846153,0.769230769230768,
0.784615384615384,0.799999999999999,0.815384615384614,0.83076923076923,
0.846153846153845,0.86153846153846,0.876923076923076,0.892307692307691,
0.907692307692306,0.923076923076922,0.938461538461537,0.953846153846152,
0.969230769230768,0.984615384615383,1.),.UNSPECIFIED.)
CURVE()
GEOMETRIC_REPRESENTATION_ITEM()
RATIONAL_B_SPLINE_CURVE((1.,1.,1.,1.,1.,1.,1.,1.,1.,1.,1.,1.,1.,1.,1.,1.,
1.,1.,1.,1.,1.,1.,1.,1.,1.,1.,1.,1.,1.,1.,1.,1.,1.,1.,1.,1.,1.,1.,1.,1.,
1.,1.,1.,1.,1.,1.,1.,1.,1.,1.,1.,1.,1.,1.,1.,1.,1.,1.,1.,1.,1.,1.,1.,1.,
1.,1.,1.,1.,1.,1.))
REPRESENTATION_ITEM('')
);
#56=(
BOUNDED_CURVE()
B_SPLINE_CURVE(5,(#23217,#23218,#23219,#23220,#23221,#23222,#23223,#23224,
#23225,#23226,#23227,#23228,#23229,#23230,#23231,#23232,#23233,#23234,#23235,
#23236,#23237,#23238,#23239,#23240,#23241,#23242,#23243,#23244,#23245,#23246,
#23247,#23248,#23249,#23250,#23251,#23252,#23253,#23254,#23255,#23256,#23257,
#23258,#23259,#23260,#23261,#23262,#23263,#23264,#23265,#23266,#23267,#23268,
#23269,#23270,#23271,#23272,#23273,#23274,#23275,#23276,#23277,#23278,#23279,
#23280,#23281,#23282,#23283,#23284,#23285,#23286),.UNSPECIFIED.,.F.,.F.)
B_SPLINE_CURVE_WITH_KNOTS((6,1,1,1,1,1,1,1,1,1,1,1,1,1,1,1,1,1,1,1,1,1,
1,1,1,1,1,1,1,1,1,1,1,1,1,1,1,1,1,1,1,1,1,1,1,1,1,1,1,1,1,1,1,1,1,1,1,1,
1,1,1,1,1,1,1,6),(0.,0.0153846153846154,0.0307692307692308,0.0461538461538462,
0.0615384615384615,0.0769230769230769,0.0923076923076923,0.107692307692308,
0.123076923076923,0.138461538461538,0.153846153846154,0.169230769230769,
0.184615384615385,0.2,0.215384615384615,0.230769230769231,0.246153846153846,
0.261538461538462,0.276923076923077,0.292307692307692,0.307692307692308,
0.323076923076923,0.338461538461538,0.353846153846154,0.369230769230769,
0.384615384615385,0.4,0.415384615384615,0.430769230769231,0.446153846153846,
0.461538461538462,0.476923076923077,0.492307692307692,0.507692307692308,
0.523076923076923,0.538461538461538,0.553846153846154,0.569230769230769,
0.584615384615384,0.6,0.615384615384615,0.63076923076923,0.646153846153846,
0.661538461538461,0.676923076923076,0.692307692307692,0.707692307692307,
0.723076923076922,0.738461538461538,0.753846153846153,0.769230769230768,
0.784615384615384,0.799999999999999,0.815384615384614,0.83076923076923,
0.846153846153845,0.86153846153846,0.876923076923076,0.892307692307691,
0.907692307692306,0.923076923076922,0.938461538461537,0.953846153846152,
0.969230769230768,0.984615384615383,1.),.UNSPECIFIED.)
CURVE()
GEOMETRIC_REPRESENTATION_ITEM()
RATIONAL_B_SPLINE_CURVE((1.,1.,1.,1.,1.,1.,1.,1.,1.,1.,1.,1.,1.,1.,1.,1.,
1.,1.,1.,1.,1.,1.,1.,1.,1.,1.,1.,1.,1.,1.,1.,1.,1.,1.,1.,1.,1.,1.,1.,1.,
1.,1.,1.,1.,1.,1.,1.,1.,1.,1.,1.,1.,1.,1.,1.,1.,1.,1.,1.,1.,1.,1.,1.,1.,
1.,1.,1.,1.,1.,1.))
REPRESENTATION_ITEM('')
);
#57=(
BOUNDED_CURVE()
B_SPLINE_CURVE(5,(#23290,#23291,#23292,#23293,#23294,#23295,#23296,#23297,
#23298,#23299,#23300,#23301,#23302,#23303,#23304,#23305,#23306,#23307,#23308,
#23309,#23310,#23311,#23312,#23313,#23314,#23315,#23316,#23317,#23318,#23319,
#23320,#23321,#23322,#23323,#23324,#23325,#23326,#23327,#23328,#23329,#23330,
#23331,#23332,#23333,#23334,#23335,#23336,#23337,#23338,#23339,#23340,#23341,
#23342,#23343,#23344,#23345,#23346,#23347,#23348,#23349,#23350,#23351,#23352,
#23353,#23354,#23355,#23356,#23357,#23358,#23359),.UNSPECIFIED.,.F.,.F.)
B_SPLINE_CURVE_WITH_KNOTS((6,1,1,1,1,1,1,1,1,1,1,1,1,1,1,1,1,1,1,1,1,1,
1,1,1,1,1,1,1,1,1,1,1,1,1,1,1,1,1,1,1,1,1,1,1,1,1,1,1,1,1,1,1,1,1,1,1,1,
1,1,1,1,1,1,1,6),(0.,0.0153846153846154,0.0307692307692308,0.0461538461538462,
0.0615384615384615,0.0769230769230769,0.0923076923076923,0.107692307692308,
0.123076923076923,0.138461538461538,0.153846153846154,0.169230769230769,
0.184615384615385,0.2,0.215384615384615,0.230769230769231,0.246153846153846,
0.261538461538462,0.276923076923077,0.292307692307692,0.307692307692308,
0.323076923076923,0.338461538461538,0.353846153846154,0.369230769230769,
0.384615384615385,0.4,0.415384615384615,0.430769230769231,0.446153846153846,
0.461538461538462,0.476923076923077,0.492307692307692,0.507692307692308,
0.523076923076923,0.538461538461538,0.553846153846154,0.569230769230769,
0.584615384615384,0.6,0.615384615384615,0.63076923076923,0.646153846153846,
0.661538461538461,0.676923076923076,0.692307692307692,0.707692307692307,
0.723076923076922,0.738461538461538,0.753846153846153,0.769230769230768,
0.784615384615384,0.799999999999999,0.815384615384614,0.83076923076923,
0.846153846153845,0.86153846153846,0.876923076923076,0.892307692307691,
0.907692307692306,0.923076923076922,0.938461538461537,0.953846153846152,
0.969230769230768,0.984615384615383,1.),.UNSPECIFIED.)
CURVE()
GEOMETRIC_REPRESENTATION_ITEM()
RATIONAL_B_SPLINE_CURVE((1.,1.,1.,1.,1.,1.,1.,1.,1.,1.,1.,1.,1.,1.,1.,1.,
1.,1.,1.,1.,1.,1.,1.,1.,1.,1.,1.,1.,1.,1.,1.,1.,1.,1.,1.,1.,1.,1.,1.,1.,
1.,1.,1.,1.,1.,1.,1.,1.,1.,1.,1.,1.,1.,1.,1.,1.,1.,1.,1.,1.,1.,1.,1.,1.,
1.,1.,1.,1.,1.,1.))
REPRESENTATION_ITEM('')
);
#58=(
BOUNDED_CURVE()
B_SPLINE_CURVE(5,(#23363,#23364,#23365,#23366,#23367,#23368,#23369,#23370,
#23371,#23372,#23373,#23374,#23375,#23376,#23377,#23378,#23379,#23380,#23381,
#23382,#23383,#23384,#23385,#23386,#23387,#23388,#23389,#23390,#23391,#23392,
#23393,#23394,#23395,#23396,#23397,#23398,#23399,#23400,#23401,#23402,#23403,
#23404,#23405,#23406,#23407,#23408,#23409,#23410,#23411,#23412,#23413,#23414,
#23415,#23416,#23417,#23418,#23419,#23420,#23421,#23422,#23423,#23424,#23425,
#23426,#23427,#23428,#23429,#23430,#23431,#23432),.UNSPECIFIED.,.F.,.F.)
B_SPLINE_CURVE_WITH_KNOTS((6,1,1,1,1,1,1,1,1,1,1,1,1,1,1,1,1,1,1,1,1,1,
1,1,1,1,1,1,1,1,1,1,1,1,1,1,1,1,1,1,1,1,1,1,1,1,1,1,1,1,1,1,1,1,1,1,1,1,
1,1,1,1,1,1,1,6),(0.,0.0153846153846154,0.0307692307692308,0.0461538461538462,
0.0615384615384615,0.0769230769230769,0.0923076923076923,0.107692307692308,
0.123076923076923,0.138461538461538,0.153846153846154,0.169230769230769,
0.184615384615385,0.2,0.215384615384615,0.230769230769231,0.246153846153846,
0.261538461538462,0.276923076923077,0.292307692307692,0.307692307692308,
0.323076923076923,0.338461538461538,0.353846153846154,0.369230769230769,
0.384615384615385,0.4,0.415384615384615,0.430769230769231,0.446153846153846,
0.461538461538462,0.476923076923077,0.492307692307692,0.507692307692308,
0.523076923076923,0.538461538461538,0.553846153846154,0.569230769230769,
0.584615384615384,0.6,0.615384615384615,0.63076923076923,0.646153846153846,
0.661538461538461,0.676923076923076,0.692307692307692,0.707692307692307,
0.723076923076922,0.738461538461538,0.753846153846153,0.769230769230768,
0.784615384615384,0.799999999999999,0.815384615384614,0.83076923076923,
0.846153846153845,0.86153846153846,0.876923076923076,0.892307692307691,
0.907692307692306,0.923076923076922,0.938461538461537,0.953846153846152,
0.969230769230768,0.984615384615383,1.),.UNSPECIFIED.)
CURVE()
GEOMETRIC_REPRESENTATION_ITEM()
RATIONAL_B_SPLINE_CURVE((1.,1.,1.,1.,1.,1.,1.,1.,1.,1.,1.,1.,1.,1.,1.,1.,
1.,1.,1.,1.,1.,1.,1.,1.,1.,1.,1.,1.,1.,1.,1.,1.,1.,1.,1.,1.,1.,1.,1.,1.,
1.,1.,1.,1.,1.,1.,1.,1.,1.,1.,1.,1.,1.,1.,1.,1.,1.,1.,1.,1.,1.,1.,1.,1.,
1.,1.,1.,1.,1.,1.))
REPRESENTATION_ITEM('')
);
#59=(
BOUNDED_CURVE()
B_SPLINE_CURVE(5,(#23436,#23437,#23438,#23439,#23440,#23441,#23442,#23443,
#23444,#23445,#23446,#23447,#23448,#23449,#23450,#23451,#23452,#23453,#23454,
#23455,#23456,#23457,#23458,#23459,#23460,#23461,#23462,#23463,#23464,#23465,
#23466,#23467,#23468,#23469,#23470,#23471,#23472,#23473,#23474,#23475,#23476,
#23477,#23478,#23479,#23480,#23481,#23482,#23483,#23484,#23485,#23486,#23487,
#23488,#23489,#23490,#23491,#23492,#23493,#23494,#23495,#23496,#23497,#23498,
#23499,#23500,#23501,#23502,#23503,#23504,#23505),.UNSPECIFIED.,.F.,.F.)
B_SPLINE_CURVE_WITH_KNOTS((6,1,1,1,1,1,1,1,1,1,1,1,1,1,1,1,1,1,1,1,1,1,
1,1,1,1,1,1,1,1,1,1,1,1,1,1,1,1,1,1,1,1,1,1,1,1,1,1,1,1,1,1,1,1,1,1,1,1,
1,1,1,1,1,1,1,6),(0.,0.0153846153846154,0.0307692307692308,0.0461538461538462,
0.0615384615384615,0.0769230769230769,0.0923076923076923,0.107692307692308,
0.123076923076923,0.138461538461538,0.153846153846154,0.169230769230769,
0.184615384615385,0.2,0.215384615384615,0.230769230769231,0.246153846153846,
0.261538461538462,0.276923076923077,0.292307692307692,0.307692307692308,
0.323076923076923,0.338461538461538,0.353846153846154,0.369230769230769,
0.384615384615385,0.4,0.415384615384615,0.430769230769231,0.446153846153846,
0.461538461538462,0.476923076923077,0.492307692307692,0.507692307692308,
0.523076923076923,0.538461538461538,0.553846153846154,0.569230769230769,
0.584615384615384,0.6,0.615384615384615,0.63076923076923,0.646153846153846,
0.661538461538461,0.676923076923076,0.692307692307692,0.707692307692307,
0.723076923076922,0.738461538461538,0.753846153846153,0.769230769230768,
0.784615384615384,0.799999999999999,0.815384615384614,0.83076923076923,
0.846153846153845,0.86153846153846,0.876923076923076,0.892307692307691,
0.907692307692306,0.923076923076922,0.938461538461537,0.953846153846152,
0.969230769230768,0.984615384615383,1.),.UNSPECIFIED.)
CURVE()
GEOMETRIC_REPRESENTATION_ITEM()
RATIONAL_B_SPLINE_CURVE((1.,1.,1.,1.,1.,1.,1.,1.,1.,1.,1.,1.,1.,1.,1.,1.,
1.,1.,1.,1.,1.,1.,1.,1.,1.,1.,1.,1.,1.,1.,1.,1.,1.,1.,1.,1.,1.,1.,1.,1.,
1.,1.,1.,1.,1.,1.,1.,1.,1.,1.,1.,1.,1.,1.,1.,1.,1.,1.,1.,1.,1.,1.,1.,1.,
1.,1.,1.,1.,1.,1.))
REPRESENTATION_ITEM('')
);
#60=(
BOUNDED_CURVE()
B_SPLINE_CURVE(5,(#23509,#23510,#23511,#23512,#23513,#23514,#23515,#23516,
#23517,#23518,#23519,#23520,#23521,#23522,#23523,#23524,#23525,#23526,#23527,
#23528,#23529,#23530,#23531,#23532,#23533,#23534,#23535,#23536,#23537,#23538,
#23539,#23540,#23541,#23542,#23543,#23544,#23545,#23546,#23547,#23548,#23549,
#23550,#23551,#23552,#23553,#23554,#23555,#23556,#23557,#23558,#23559,#23560,
#23561,#23562,#23563,#23564,#23565,#23566,#23567,#23568,#23569,#23570,#23571,
#23572,#23573,#23574,#23575,#23576,#23577,#23578),.UNSPECIFIED.,.F.,.F.)
B_SPLINE_CURVE_WITH_KNOTS((6,1,1,1,1,1,1,1,1,1,1,1,1,1,1,1,1,1,1,1,1,1,
1,1,1,1,1,1,1,1,1,1,1,1,1,1,1,1,1,1,1,1,1,1,1,1,1,1,1,1,1,1,1,1,1,1,1,1,
1,1,1,1,1,1,1,6),(0.,0.0153846153846154,0.0307692307692308,0.0461538461538462,
0.0615384615384615,0.0769230769230769,0.0923076923076923,0.107692307692308,
0.123076923076923,0.138461538461538,0.153846153846154,0.169230769230769,
0.184615384615385,0.2,0.215384615384615,0.230769230769231,0.246153846153846,
0.261538461538462,0.276923076923077,0.292307692307692,0.307692307692308,
0.323076923076923,0.338461538461538,0.353846153846154,0.369230769230769,
0.384615384615385,0.4,0.415384615384615,0.430769230769231,0.446153846153846,
0.461538461538462,0.476923076923077,0.492307692307692,0.507692307692308,
0.523076923076923,0.538461538461538,0.553846153846154,0.569230769230769,
0.584615384615384,0.6,0.615384615384615,0.63076923076923,0.646153846153846,
0.661538461538461,0.676923076923076,0.692307692307692,0.707692307692307,
0.723076923076922,0.738461538461538,0.753846153846153,0.769230769230768,
0.784615384615384,0.799999999999999,0.815384615384614,0.83076923076923,
0.846153846153845,0.86153846153846,0.876923076923076,0.892307692307691,
0.907692307692306,0.923076923076922,0.938461538461537,0.953846153846152,
0.969230769230768,0.984615384615383,1.),.UNSPECIFIED.)
CURVE()
GEOMETRIC_REPRESENTATION_ITEM()
RATIONAL_B_SPLINE_CURVE((1.,1.,1.,1.,1.,1.,1.,1.,1.,1.,1.,1.,1.,1.,1.,1.,
1.,1.,1.,1.,1.,1.,1.,1.,1.,1.,1.,1.,1.,1.,1.,1.,1.,1.,1.,1.,1.,1.,1.,1.,
1.,1.,1.,1.,1.,1.,1.,1.,1.,1.,1.,1.,1.,1.,1.,1.,1.,1.,1.,1.,1.,1.,1.,1.,
1.,1.,1.,1.,1.,1.))
REPRESENTATION_ITEM('')
);
#61=(
BOUNDED_CURVE()
B_SPLINE_CURVE(5,(#23582,#23583,#23584,#23585,#23586,#23587,#23588,#23589,
#23590,#23591,#23592,#23593,#23594,#23595,#23596,#23597,#23598,#23599,#23600,
#23601,#23602,#23603,#23604,#23605,#23606,#23607,#23608,#23609,#23610,#23611,
#23612,#23613,#23614,#23615,#23616,#23617,#23618,#23619,#23620,#23621,#23622,
#23623,#23624,#23625,#23626,#23627,#23628,#23629,#23630,#23631,#23632,#23633,
#23634,#23635,#23636,#23637,#23638,#23639,#23640,#23641,#23642,#23643,#23644,
#23645,#23646,#23647,#23648,#23649,#23650,#23651),.UNSPECIFIED.,.F.,.F.)
B_SPLINE_CURVE_WITH_KNOTS((6,1,1,1,1,1,1,1,1,1,1,1,1,1,1,1,1,1,1,1,1,1,
1,1,1,1,1,1,1,1,1,1,1,1,1,1,1,1,1,1,1,1,1,1,1,1,1,1,1,1,1,1,1,1,1,1,1,1,
1,1,1,1,1,1,1,6),(0.,0.0153846153846154,0.0307692307692308,0.0461538461538462,
0.0615384615384615,0.0769230769230769,0.0923076923076923,0.107692307692308,
0.123076923076923,0.138461538461538,0.153846153846154,0.169230769230769,
0.184615384615385,0.2,0.215384615384615,0.230769230769231,0.246153846153846,
0.261538461538462,0.276923076923077,0.292307692307692,0.307692307692308,
0.323076923076923,0.338461538461538,0.353846153846154,0.369230769230769,
0.384615384615385,0.4,0.415384615384615,0.430769230769231,0.446153846153846,
0.461538461538462,0.476923076923077,0.492307692307692,0.507692307692308,
0.523076923076923,0.538461538461538,0.553846153846154,0.569230769230769,
0.584615384615384,0.6,0.615384615384615,0.63076923076923,0.646153846153846,
0.661538461538461,0.676923076923076,0.692307692307692,0.707692307692307,
0.723076923076922,0.738461538461538,0.753846153846153,0.769230769230768,
0.784615384615384,0.799999999999999,0.815384615384614,0.83076923076923,
0.846153846153845,0.86153846153846,0.876923076923076,0.892307692307691,
0.907692307692306,0.923076923076922,0.938461538461537,0.953846153846152,
0.969230769230768,0.984615384615383,1.),.UNSPECIFIED.)
CURVE()
GEOMETRIC_REPRESENTATION_ITEM()
RATIONAL_B_SPLINE_CURVE((1.,1.,1.,1.,1.,1.,1.,1.,1.,1.,1.,1.,1.,1.,1.,1.,
1.,1.,1.,1.,1.,1.,1.,1.,1.,1.,1.,1.,1.,1.,1.,1.,1.,1.,1.,1.,1.,1.,1.,1.,
1.,1.,1.,1.,1.,1.,1.,1.,1.,1.,1.,1.,1.,1.,1.,1.,1.,1.,1.,1.,1.,1.,1.,1.,
1.,1.,1.,1.,1.,1.))
REPRESENTATION_ITEM('')
);
#62=(
BOUNDED_CURVE()
B_SPLINE_CURVE(5,(#23655,#23656,#23657,#23658,#23659,#23660,#23661,#23662,
#23663,#23664,#23665,#23666,#23667,#23668,#23669,#23670,#23671,#23672,#23673,
#23674,#23675,#23676,#23677,#23678,#23679,#23680,#23681,#23682,#23683,#23684,
#23685,#23686,#23687,#23688,#23689,#23690,#23691,#23692,#23693,#23694,#23695,
#23696,#23697,#23698,#23699,#23700,#23701,#23702,#23703,#23704,#23705,#23706,
#23707,#23708,#23709,#23710,#23711,#23712,#23713,#23714,#23715,#23716,#23717,
#23718,#23719,#23720,#23721,#23722,#23723,#23724),.UNSPECIFIED.,.F.,.F.)
B_SPLINE_CURVE_WITH_KNOTS((6,1,1,1,1,1,1,1,1,1,1,1,1,1,1,1,1,1,1,1,1,1,
1,1,1,1,1,1,1,1,1,1,1,1,1,1,1,1,1,1,1,1,1,1,1,1,1,1,1,1,1,1,1,1,1,1,1,1,
1,1,1,1,1,1,1,6),(0.,0.0153846153846154,0.0307692307692308,0.0461538461538462,
0.0615384615384615,0.0769230769230769,0.0923076923076923,0.107692307692308,
0.123076923076923,0.138461538461538,0.153846153846154,0.169230769230769,
0.184615384615385,0.2,0.215384615384615,0.230769230769231,0.246153846153846,
0.261538461538462,0.276923076923077,0.292307692307692,0.307692307692308,
0.323076923076923,0.338461538461538,0.353846153846154,0.369230769230769,
0.384615384615385,0.4,0.415384615384615,0.430769230769231,0.446153846153846,
0.461538461538462,0.476923076923077,0.492307692307692,0.507692307692308,
0.523076923076923,0.538461538461538,0.553846153846154,0.569230769230769,
0.584615384615384,0.6,0.615384615384615,0.63076923076923,0.646153846153846,
0.661538461538461,0.676923076923076,0.692307692307692,0.707692307692307,
0.723076923076922,0.738461538461538,0.753846153846153,0.769230769230768,
0.784615384615384,0.799999999999999,0.815384615384614,0.83076923076923,
0.846153846153845,0.86153846153846,0.876923076923076,0.892307692307691,
0.907692307692306,0.923076923076922,0.938461538461537,0.953846153846152,
0.969230769230768,0.984615384615383,1.),.UNSPECIFIED.)
CURVE()
GEOMETRIC_REPRESENTATION_ITEM()
RATIONAL_B_SPLINE_CURVE((1.,1.,1.,1.,1.,1.,1.,1.,1.,1.,1.,1.,1.,1.,1.,1.,
1.,1.,1.,1.,1.,1.,1.,1.,1.,1.,1.,1.,1.,1.,1.,1.,1.,1.,1.,1.,1.,1.,1.,1.,
1.,1.,1.,1.,1.,1.,1.,1.,1.,1.,1.,1.,1.,1.,1.,1.,1.,1.,1.,1.,1.,1.,1.,1.,
1.,1.,1.,1.,1.,1.))
REPRESENTATION_ITEM('')
);
#63=(
BOUNDED_CURVE()
B_SPLINE_CURVE(5,(#23728,#23729,#23730,#23731,#23732,#23733,#23734,#23735,
#23736,#23737,#23738,#23739,#23740,#23741,#23742,#23743,#23744,#23745,#23746,
#23747,#23748,#23749,#23750,#23751,#23752,#23753,#23754,#23755,#23756,#23757,
#23758,#23759,#23760,#23761,#23762,#23763,#23764,#23765,#23766,#23767,#23768,
#23769,#23770,#23771,#23772,#23773,#23774,#23775,#23776,#23777,#23778,#23779,
#23780,#23781,#23782,#23783,#23784,#23785,#23786,#23787,#23788,#23789,#23790,
#23791,#23792,#23793,#23794,#23795,#23796,#23797),.UNSPECIFIED.,.F.,.F.)
B_SPLINE_CURVE_WITH_KNOTS((6,1,1,1,1,1,1,1,1,1,1,1,1,1,1,1,1,1,1,1,1,1,
1,1,1,1,1,1,1,1,1,1,1,1,1,1,1,1,1,1,1,1,1,1,1,1,1,1,1,1,1,1,1,1,1,1,1,1,
1,1,1,1,1,1,1,6),(0.,0.0153846153846154,0.0307692307692308,0.0461538461538462,
0.0615384615384615,0.0769230769230769,0.0923076923076923,0.107692307692308,
0.123076923076923,0.138461538461538,0.153846153846154,0.169230769230769,
0.184615384615385,0.2,0.215384615384615,0.230769230769231,0.246153846153846,
0.261538461538462,0.276923076923077,0.292307692307692,0.307692307692308,
0.323076923076923,0.338461538461538,0.353846153846154,0.369230769230769,
0.384615384615385,0.4,0.415384615384615,0.430769230769231,0.446153846153846,
0.461538461538462,0.476923076923077,0.492307692307692,0.507692307692308,
0.523076923076923,0.538461538461538,0.553846153846154,0.569230769230769,
0.584615384615384,0.6,0.615384615384615,0.63076923076923,0.646153846153846,
0.661538461538461,0.676923076923076,0.692307692307692,0.707692307692307,
0.723076923076922,0.738461538461538,0.753846153846153,0.769230769230768,
0.784615384615384,0.799999999999999,0.815384615384614,0.83076923076923,
0.846153846153845,0.86153846153846,0.876923076923076,0.892307692307691,
0.907692307692306,0.923076923076922,0.938461538461537,0.953846153846152,
0.969230769230768,0.984615384615383,1.),.UNSPECIFIED.)
CURVE()
GEOMETRIC_REPRESENTATION_ITEM()
RATIONAL_B_SPLINE_CURVE((1.,1.,1.,1.,1.,1.,1.,1.,1.,1.,1.,1.,1.,1.,1.,1.,
1.,1.,1.,1.,1.,1.,1.,1.,1.,1.,1.,1.,1.,1.,1.,1.,1.,1.,1.,1.,1.,1.,1.,1.,
1.,1.,1.,1.,1.,1.,1.,1.,1.,1.,1.,1.,1.,1.,1.,1.,1.,1.,1.,1.,1.,1.,1.,1.,
1.,1.,1.,1.,1.,1.))
REPRESENTATION_ITEM('')
);
#64=(
BOUNDED_CURVE()
B_SPLINE_CURVE(5,(#23801,#23802,#23803,#23804,#23805,#23806,#23807,#23808,
#23809,#23810,#23811,#23812,#23813,#23814,#23815,#23816,#23817,#23818,#23819,
#23820,#23821,#23822,#23823,#23824,#23825,#23826,#23827,#23828,#23829,#23830,
#23831,#23832,#23833,#23834,#23835,#23836,#23837,#23838,#23839,#23840,#23841,
#23842,#23843,#23844,#23845,#23846,#23847,#23848,#23849,#23850,#23851,#23852,
#23853,#23854,#23855,#23856,#23857,#23858,#23859,#23860,#23861,#23862,#23863,
#23864,#23865,#23866,#23867,#23868,#23869,#23870),.UNSPECIFIED.,.F.,.F.)
B_SPLINE_CURVE_WITH_KNOTS((6,1,1,1,1,1,1,1,1,1,1,1,1,1,1,1,1,1,1,1,1,1,
1,1,1,1,1,1,1,1,1,1,1,1,1,1,1,1,1,1,1,1,1,1,1,1,1,1,1,1,1,1,1,1,1,1,1,1,
1,1,1,1,1,1,1,6),(0.,0.0153846153846154,0.0307692307692308,0.0461538461538462,
0.0615384615384615,0.0769230769230769,0.0923076923076923,0.107692307692308,
0.123076923076923,0.138461538461538,0.153846153846154,0.169230769230769,
0.184615384615385,0.2,0.215384615384615,0.230769230769231,0.246153846153846,
0.261538461538462,0.276923076923077,0.292307692307692,0.307692307692308,
0.323076923076923,0.338461538461538,0.353846153846154,0.369230769230769,
0.384615384615385,0.4,0.415384615384615,0.430769230769231,0.446153846153846,
0.461538461538462,0.476923076923077,0.492307692307692,0.507692307692308,
0.523076923076923,0.538461538461538,0.553846153846154,0.569230769230769,
0.584615384615384,0.6,0.615384615384615,0.63076923076923,0.646153846153846,
0.661538461538461,0.676923076923076,0.692307692307692,0.707692307692307,
0.723076923076922,0.738461538461538,0.753846153846153,0.769230769230768,
0.784615384615384,0.799999999999999,0.815384615384614,0.83076923076923,
0.846153846153845,0.86153846153846,0.876923076923076,0.892307692307691,
0.907692307692306,0.923076923076922,0.938461538461537,0.953846153846152,
0.969230769230768,0.984615384615383,1.),.UNSPECIFIED.)
CURVE()
GEOMETRIC_REPRESENTATION_ITEM()
RATIONAL_B_SPLINE_CURVE((1.,1.,1.,1.,1.,1.,1.,1.,1.,1.,1.,1.,1.,1.,1.,1.,
1.,1.,1.,1.,1.,1.,1.,1.,1.,1.,1.,1.,1.,1.,1.,1.,1.,1.,1.,1.,1.,1.,1.,1.,
1.,1.,1.,1.,1.,1.,1.,1.,1.,1.,1.,1.,1.,1.,1.,1.,1.,1.,1.,1.,1.,1.,1.,1.,
1.,1.,1.,1.,1.,1.))
REPRESENTATION_ITEM('')
);
#65=(
BOUNDED_CURVE()
B_SPLINE_CURVE(5,(#23874,#23875,#23876,#23877,#23878,#23879,#23880,#23881,
#23882,#23883,#23884,#23885,#23886,#23887,#23888,#23889,#23890,#23891,#23892,
#23893,#23894,#23895,#23896,#23897,#23898,#23899,#23900,#23901,#23902,#23903,
#23904,#23905,#23906,#23907,#23908,#23909,#23910,#23911,#23912,#23913,#23914,
#23915,#23916,#23917,#23918,#23919,#23920,#23921,#23922,#23923,#23924,#23925,
#23926,#23927,#23928,#23929,#23930,#23931,#23932,#23933,#23934,#23935,#23936,
#23937,#23938,#23939,#23940,#23941,#23942,#23943),.UNSPECIFIED.,.F.,.F.)
B_SPLINE_CURVE_WITH_KNOTS((6,1,1,1,1,1,1,1,1,1,1,1,1,1,1,1,1,1,1,1,1,1,
1,1,1,1,1,1,1,1,1,1,1,1,1,1,1,1,1,1,1,1,1,1,1,1,1,1,1,1,1,1,1,1,1,1,1,1,
1,1,1,1,1,1,1,6),(0.,0.0153846153846154,0.0307692307692308,0.0461538461538462,
0.0615384615384615,0.0769230769230769,0.0923076923076923,0.107692307692308,
0.123076923076923,0.138461538461538,0.153846153846154,0.169230769230769,
0.184615384615385,0.2,0.215384615384615,0.230769230769231,0.246153846153846,
0.261538461538462,0.276923076923077,0.292307692307692,0.307692307692308,
0.323076923076923,0.338461538461538,0.353846153846154,0.369230769230769,
0.384615384615385,0.4,0.415384615384615,0.430769230769231,0.446153846153846,
0.461538461538462,0.476923076923077,0.492307692307692,0.507692307692308,
0.523076923076923,0.538461538461538,0.553846153846154,0.569230769230769,
0.584615384615384,0.6,0.615384615384615,0.63076923076923,0.646153846153846,
0.661538461538461,0.676923076923076,0.692307692307692,0.707692307692307,
0.723076923076922,0.738461538461538,0.753846153846153,0.769230769230768,
0.784615384615384,0.799999999999999,0.815384615384614,0.83076923076923,
0.846153846153845,0.86153846153846,0.876923076923076,0.892307692307691,
0.907692307692306,0.923076923076922,0.938461538461537,0.953846153846152,
0.969230769230768,0.984615384615383,1.),.UNSPECIFIED.)
CURVE()
GEOMETRIC_REPRESENTATION_ITEM()
RATIONAL_B_SPLINE_CURVE((1.,1.,1.,1.,1.,1.,1.,1.,1.,1.,1.,1.,1.,1.,1.,1.,
1.,1.,1.,1.,1.,1.,1.,1.,1.,1.,1.,1.,1.,1.,1.,1.,1.,1.,1.,1.,1.,1.,1.,1.,
1.,1.,1.,1.,1.,1.,1.,1.,1.,1.,1.,1.,1.,1.,1.,1.,1.,1.,1.,1.,1.,1.,1.,1.,
1.,1.,1.,1.,1.,1.))
REPRESENTATION_ITEM('')
);
#66=(
BOUNDED_CURVE()
B_SPLINE_CURVE(5,(#23947,#23948,#23949,#23950,#23951,#23952,#23953,#23954,
#23955,#23956,#23957,#23958,#23959,#23960,#23961,#23962,#23963,#23964,#23965,
#23966,#23967,#23968,#23969,#23970,#23971,#23972,#23973,#23974,#23975,#23976,
#23977,#23978,#23979,#23980,#23981,#23982,#23983,#23984,#23985,#23986,#23987,
#23988,#23989,#23990,#23991,#23992,#23993,#23994,#23995,#23996,#23997,#23998,
#23999,#24000,#24001,#24002,#24003,#24004,#24005,#24006,#24007,#24008,#24009,
#24010,#24011,#24012,#24013,#24014,#24015,#24016),.UNSPECIFIED.,.F.,.F.)
B_SPLINE_CURVE_WITH_KNOTS((6,1,1,1,1,1,1,1,1,1,1,1,1,1,1,1,1,1,1,1,1,1,
1,1,1,1,1,1,1,1,1,1,1,1,1,1,1,1,1,1,1,1,1,1,1,1,1,1,1,1,1,1,1,1,1,1,1,1,
1,1,1,1,1,1,1,6),(0.,0.0153846153846154,0.0307692307692308,0.0461538461538462,
0.0615384615384615,0.0769230769230769,0.0923076923076923,0.107692307692308,
0.123076923076923,0.138461538461538,0.153846153846154,0.169230769230769,
0.184615384615385,0.2,0.215384615384615,0.230769230769231,0.246153846153846,
0.261538461538462,0.276923076923077,0.292307692307692,0.307692307692308,
0.323076923076923,0.338461538461538,0.353846153846154,0.369230769230769,
0.384615384615385,0.4,0.415384615384615,0.430769230769231,0.446153846153846,
0.461538461538462,0.476923076923077,0.492307692307692,0.507692307692308,
0.523076923076923,0.538461538461538,0.553846153846154,0.569230769230769,
0.584615384615384,0.6,0.615384615384615,0.63076923076923,0.646153846153846,
0.661538461538461,0.676923076923076,0.692307692307692,0.707692307692307,
0.723076923076922,0.738461538461538,0.753846153846153,0.769230769230768,
0.784615384615384,0.799999999999999,0.815384615384614,0.83076923076923,
0.846153846153845,0.86153846153846,0.876923076923076,0.892307692307691,
0.907692307692306,0.923076923076922,0.938461538461537,0.953846153846152,
0.969230769230768,0.984615384615383,1.),.UNSPECIFIED.)
CURVE()
GEOMETRIC_REPRESENTATION_ITEM()
RATIONAL_B_SPLINE_CURVE((1.,1.,1.,1.,1.,1.,1.,1.,1.,1.,1.,1.,1.,1.,1.,1.,
1.,1.,1.,1.,1.,1.,1.,1.,1.,1.,1.,1.,1.,1.,1.,1.,1.,1.,1.,1.,1.,1.,1.,1.,
1.,1.,1.,1.,1.,1.,1.,1.,1.,1.,1.,1.,1.,1.,1.,1.,1.,1.,1.,1.,1.,1.,1.,1.,
1.,1.,1.,1.,1.,1.))
REPRESENTATION_ITEM('')
);
#67=(
BOUNDED_CURVE()
B_SPLINE_CURVE(5,(#24020,#24021,#24022,#24023,#24024,#24025,#24026,#24027,
#24028,#24029,#24030,#24031,#24032,#24033,#24034,#24035,#24036,#24037,#24038,
#24039,#24040,#24041,#24042,#24043,#24044,#24045,#24046,#24047,#24048,#24049,
#24050,#24051,#24052,#24053,#24054,#24055,#24056,#24057,#24058,#24059,#24060,
#24061,#24062,#24063,#24064,#24065,#24066,#24067,#24068,#24069,#24070,#24071,
#24072,#24073,#24074,#24075,#24076,#24077,#24078,#24079,#24080,#24081,#24082,
#24083,#24084,#24085,#24086,#24087,#24088,#24089),.UNSPECIFIED.,.F.,.F.)
B_SPLINE_CURVE_WITH_KNOTS((6,1,1,1,1,1,1,1,1,1,1,1,1,1,1,1,1,1,1,1,1,1,
1,1,1,1,1,1,1,1,1,1,1,1,1,1,1,1,1,1,1,1,1,1,1,1,1,1,1,1,1,1,1,1,1,1,1,1,
1,1,1,1,1,1,1,6),(0.,0.0153846153846154,0.0307692307692308,0.0461538461538462,
0.0615384615384615,0.0769230769230769,0.0923076923076923,0.107692307692308,
0.123076923076923,0.138461538461538,0.153846153846154,0.169230769230769,
0.184615384615385,0.2,0.215384615384615,0.230769230769231,0.246153846153846,
0.261538461538462,0.276923076923077,0.292307692307692,0.307692307692308,
0.323076923076923,0.338461538461538,0.353846153846154,0.369230769230769,
0.384615384615385,0.4,0.415384615384615,0.430769230769231,0.446153846153846,
0.461538461538462,0.476923076923077,0.492307692307692,0.507692307692308,
0.523076923076923,0.538461538461538,0.553846153846154,0.569230769230769,
0.584615384615384,0.6,0.615384615384615,0.63076923076923,0.646153846153846,
0.661538461538461,0.676923076923076,0.692307692307692,0.707692307692307,
0.723076923076922,0.738461538461538,0.753846153846153,0.769230769230768,
0.784615384615384,0.799999999999999,0.815384615384614,0.83076923076923,
0.846153846153845,0.86153846153846,0.876923076923076,0.892307692307691,
0.907692307692306,0.923076923076922,0.938461538461537,0.953846153846152,
0.969230769230768,0.984615384615383,1.),.UNSPECIFIED.)
CURVE()
GEOMETRIC_REPRESENTATION_ITEM()
RATIONAL_B_SPLINE_CURVE((1.,1.,1.,1.,1.,1.,1.,1.,1.,1.,1.,1.,1.,1.,1.,1.,
1.,1.,1.,1.,1.,1.,1.,1.,1.,1.,1.,1.,1.,1.,1.,1.,1.,1.,1.,1.,1.,1.,1.,1.,
1.,1.,1.,1.,1.,1.,1.,1.,1.,1.,1.,1.,1.,1.,1.,1.,1.,1.,1.,1.,1.,1.,1.,1.,
1.,1.,1.,1.,1.,1.))
REPRESENTATION_ITEM('')
);
#68=(
BOUNDED_CURVE()
B_SPLINE_CURVE(5,(#24093,#24094,#24095,#24096,#24097,#24098,#24099,#24100,
#24101,#24102,#24103,#24104,#24105,#24106,#24107,#24108,#24109,#24110,#24111,
#24112,#24113,#24114,#24115,#24116,#24117,#24118,#24119,#24120,#24121,#24122,
#24123,#24124,#24125,#24126,#24127,#24128,#24129,#24130,#24131,#24132,#24133,
#24134,#24135,#24136,#24137,#24138,#24139,#24140,#24141,#24142,#24143,#24144,
#24145,#24146,#24147,#24148,#24149,#24150,#24151,#24152,#24153,#24154,#24155,
#24156,#24157,#24158,#24159,#24160,#24161,#24162),.UNSPECIFIED.,.F.,.F.)
B_SPLINE_CURVE_WITH_KNOTS((6,1,1,1,1,1,1,1,1,1,1,1,1,1,1,1,1,1,1,1,1,1,
1,1,1,1,1,1,1,1,1,1,1,1,1,1,1,1,1,1,1,1,1,1,1,1,1,1,1,1,1,1,1,1,1,1,1,1,
1,1,1,1,1,1,1,6),(0.,0.0153846153846154,0.0307692307692308,0.0461538461538462,
0.0615384615384615,0.0769230769230769,0.0923076923076923,0.107692307692308,
0.123076923076923,0.138461538461538,0.153846153846154,0.169230769230769,
0.184615384615385,0.2,0.215384615384615,0.230769230769231,0.246153846153846,
0.261538461538462,0.276923076923077,0.292307692307692,0.307692307692308,
0.323076923076923,0.338461538461538,0.353846153846154,0.369230769230769,
0.384615384615385,0.4,0.415384615384615,0.430769230769231,0.446153846153846,
0.461538461538462,0.476923076923077,0.492307692307692,0.507692307692308,
0.523076923076923,0.538461538461538,0.553846153846154,0.569230769230769,
0.584615384615384,0.6,0.615384615384615,0.63076923076923,0.646153846153846,
0.661538461538461,0.676923076923076,0.692307692307692,0.707692307692307,
0.723076923076922,0.738461538461538,0.753846153846153,0.769230769230768,
0.784615384615384,0.799999999999999,0.815384615384614,0.83076923076923,
0.846153846153845,0.86153846153846,0.876923076923076,0.892307692307691,
0.907692307692306,0.923076923076922,0.938461538461537,0.953846153846152,
0.969230769230768,0.984615384615383,1.),.UNSPECIFIED.)
CURVE()
GEOMETRIC_REPRESENTATION_ITEM()
RATIONAL_B_SPLINE_CURVE((1.,1.,1.,1.,1.,1.,1.,1.,1.,1.,1.,1.,1.,1.,1.,1.,
1.,1.,1.,1.,1.,1.,1.,1.,1.,1.,1.,1.,1.,1.,1.,1.,1.,1.,1.,1.,1.,1.,1.,1.,
1.,1.,1.,1.,1.,1.,1.,1.,1.,1.,1.,1.,1.,1.,1.,1.,1.,1.,1.,1.,1.,1.,1.,1.,
1.,1.,1.,1.,1.,1.))
REPRESENTATION_ITEM('')
);
#69=(
BOUNDED_CURVE()
B_SPLINE_CURVE(5,(#24166,#24167,#24168,#24169,#24170,#24171,#24172,#24173,
#24174,#24175,#24176,#24177,#24178,#24179,#24180,#24181,#24182,#24183,#24184,
#24185,#24186,#24187,#24188,#24189,#24190,#24191,#24192,#24193,#24194,#24195,
#24196,#24197,#24198,#24199,#24200,#24201,#24202,#24203,#24204,#24205,#24206,
#24207,#24208,#24209,#24210,#24211,#24212,#24213,#24214,#24215,#24216,#24217,
#24218,#24219,#24220,#24221,#24222,#24223,#24224,#24225,#24226,#24227,#24228,
#24229,#24230,#24231,#24232,#24233,#24234,#24235),.UNSPECIFIED.,.F.,.F.)
B_SPLINE_CURVE_WITH_KNOTS((6,1,1,1,1,1,1,1,1,1,1,1,1,1,1,1,1,1,1,1,1,1,
1,1,1,1,1,1,1,1,1,1,1,1,1,1,1,1,1,1,1,1,1,1,1,1,1,1,1,1,1,1,1,1,1,1,1,1,
1,1,1,1,1,1,1,6),(0.,0.0153846153846154,0.0307692307692308,0.0461538461538462,
0.0615384615384615,0.0769230769230769,0.0923076923076923,0.107692307692308,
0.123076923076923,0.138461538461538,0.153846153846154,0.169230769230769,
0.184615384615385,0.2,0.215384615384615,0.230769230769231,0.246153846153846,
0.261538461538462,0.276923076923077,0.292307692307692,0.307692307692308,
0.323076923076923,0.338461538461538,0.353846153846154,0.369230769230769,
0.384615384615385,0.4,0.415384615384615,0.430769230769231,0.446153846153846,
0.461538461538462,0.476923076923077,0.492307692307692,0.507692307692308,
0.523076923076923,0.538461538461538,0.553846153846154,0.569230769230769,
0.584615384615384,0.6,0.615384615384615,0.63076923076923,0.646153846153846,
0.661538461538461,0.676923076923076,0.692307692307692,0.707692307692307,
0.723076923076922,0.738461538461538,0.753846153846153,0.769230769230768,
0.784615384615384,0.799999999999999,0.815384615384614,0.83076923076923,
0.846153846153845,0.86153846153846,0.876923076923076,0.892307692307691,
0.907692307692306,0.923076923076922,0.938461538461537,0.953846153846152,
0.969230769230768,0.984615384615383,1.),.UNSPECIFIED.)
CURVE()
GEOMETRIC_REPRESENTATION_ITEM()
RATIONAL_B_SPLINE_CURVE((1.,1.,1.,1.,1.,1.,1.,1.,1.,1.,1.,1.,1.,1.,1.,1.,
1.,1.,1.,1.,1.,1.,1.,1.,1.,1.,1.,1.,1.,1.,1.,1.,1.,1.,1.,1.,1.,1.,1.,1.,
1.,1.,1.,1.,1.,1.,1.,1.,1.,1.,1.,1.,1.,1.,1.,1.,1.,1.,1.,1.,1.,1.,1.,1.,
1.,1.,1.,1.,1.,1.))
REPRESENTATION_ITEM('')
);
#70=(
BOUNDED_CURVE()
B_SPLINE_CURVE(5,(#24239,#24240,#24241,#24242,#24243,#24244,#24245,#24246,
#24247,#24248,#24249,#24250,#24251,#24252,#24253,#24254,#24255,#24256,#24257,
#24258,#24259,#24260,#24261,#24262,#24263,#24264,#24265,#24266,#24267,#24268,
#24269,#24270,#24271,#24272,#24273,#24274,#24275,#24276,#24277,#24278,#24279,
#24280,#24281,#24282,#24283,#24284,#24285,#24286,#24287,#24288,#24289,#24290,
#24291,#24292,#24293,#24294,#24295,#24296,#24297,#24298,#24299,#24300,#24301,
#24302,#24303,#24304,#24305,#24306,#24307,#24308),.UNSPECIFIED.,.F.,.F.)
B_SPLINE_CURVE_WITH_KNOTS((6,1,1,1,1,1,1,1,1,1,1,1,1,1,1,1,1,1,1,1,1,1,
1,1,1,1,1,1,1,1,1,1,1,1,1,1,1,1,1,1,1,1,1,1,1,1,1,1,1,1,1,1,1,1,1,1,1,1,
1,1,1,1,1,1,1,6),(0.,0.0153846153846154,0.0307692307692308,0.0461538461538462,
0.0615384615384615,0.0769230769230769,0.0923076923076923,0.107692307692308,
0.123076923076923,0.138461538461538,0.153846153846154,0.169230769230769,
0.184615384615385,0.2,0.215384615384615,0.230769230769231,0.246153846153846,
0.261538461538462,0.276923076923077,0.292307692307692,0.307692307692308,
0.323076923076923,0.338461538461538,0.353846153846154,0.369230769230769,
0.384615384615385,0.4,0.415384615384615,0.430769230769231,0.446153846153846,
0.461538461538462,0.476923076923077,0.492307692307692,0.507692307692308,
0.523076923076923,0.538461538461538,0.553846153846154,0.569230769230769,
0.584615384615384,0.6,0.615384615384615,0.63076923076923,0.646153846153846,
0.661538461538461,0.676923076923076,0.692307692307692,0.707692307692307,
0.723076923076922,0.738461538461538,0.753846153846153,0.769230769230768,
0.784615384615384,0.799999999999999,0.815384615384614,0.83076923076923,
0.846153846153845,0.86153846153846,0.876923076923076,0.892307692307691,
0.907692307692306,0.923076923076922,0.938461538461537,0.953846153846152,
0.969230769230768,0.984615384615383,1.),.UNSPECIFIED.)
CURVE()
GEOMETRIC_REPRESENTATION_ITEM()
RATIONAL_B_SPLINE_CURVE((1.,1.,1.,1.,1.,1.,1.,1.,1.,1.,1.,1.,1.,1.,1.,1.,
1.,1.,1.,1.,1.,1.,1.,1.,1.,1.,1.,1.,1.,1.,1.,1.,1.,1.,1.,1.,1.,1.,1.,1.,
1.,1.,1.,1.,1.,1.,1.,1.,1.,1.,1.,1.,1.,1.,1.,1.,1.,1.,1.,1.,1.,1.,1.,1.,
1.,1.,1.,1.,1.,1.))
REPRESENTATION_ITEM('')
);
#71=(
BOUNDED_CURVE()
B_SPLINE_CURVE(5,(#24312,#24313,#24314,#24315,#24316,#24317,#24318,#24319,
#24320,#24321,#24322,#24323,#24324,#24325,#24326,#24327,#24328,#24329,#24330,
#24331,#24332,#24333,#24334,#24335,#24336,#24337,#24338,#24339,#24340,#24341,
#24342,#24343,#24344,#24345,#24346,#24347,#24348,#24349,#24350,#24351,#24352,
#24353,#24354,#24355,#24356,#24357,#24358,#24359,#24360,#24361,#24362,#24363,
#24364,#24365,#24366,#24367,#24368,#24369,#24370,#24371,#24372,#24373,#24374,
#24375,#24376,#24377,#24378,#24379,#24380,#24381),.UNSPECIFIED.,.F.,.F.)
B_SPLINE_CURVE_WITH_KNOTS((6,1,1,1,1,1,1,1,1,1,1,1,1,1,1,1,1,1,1,1,1,1,
1,1,1,1,1,1,1,1,1,1,1,1,1,1,1,1,1,1,1,1,1,1,1,1,1,1,1,1,1,1,1,1,1,1,1,1,
1,1,1,1,1,1,1,6),(0.,0.0153846153846154,0.0307692307692308,0.0461538461538462,
0.0615384615384615,0.0769230769230769,0.0923076923076923,0.107692307692308,
0.123076923076923,0.138461538461538,0.153846153846154,0.169230769230769,
0.184615384615385,0.2,0.215384615384615,0.230769230769231,0.246153846153846,
0.261538461538462,0.276923076923077,0.292307692307692,0.307692307692308,
0.323076923076923,0.338461538461538,0.353846153846154,0.369230769230769,
0.384615384615385,0.4,0.415384615384615,0.430769230769231,0.446153846153846,
0.461538461538462,0.476923076923077,0.492307692307692,0.507692307692308,
0.523076923076923,0.538461538461538,0.553846153846154,0.569230769230769,
0.584615384615384,0.6,0.615384615384615,0.63076923076923,0.646153846153846,
0.661538461538461,0.676923076923076,0.692307692307692,0.707692307692307,
0.723076923076922,0.738461538461538,0.753846153846153,0.769230769230768,
0.784615384615384,0.799999999999999,0.815384615384614,0.83076923076923,
0.846153846153845,0.86153846153846,0.876923076923076,0.892307692307691,
0.907692307692306,0.923076923076922,0.938461538461537,0.953846153846152,
0.969230769230768,0.984615384615383,1.),.UNSPECIFIED.)
CURVE()
GEOMETRIC_REPRESENTATION_ITEM()
RATIONAL_B_SPLINE_CURVE((1.,1.,1.,1.,1.,1.,1.,1.,1.,1.,1.,1.,1.,1.,1.,1.,
1.,1.,1.,1.,1.,1.,1.,1.,1.,1.,1.,1.,1.,1.,1.,1.,1.,1.,1.,1.,1.,1.,1.,1.,
1.,1.,1.,1.,1.,1.,1.,1.,1.,1.,1.,1.,1.,1.,1.,1.,1.,1.,1.,1.,1.,1.,1.,1.,
1.,1.,1.,1.,1.,1.))
REPRESENTATION_ITEM('')
);
#72=(
BOUNDED_CURVE()
B_SPLINE_CURVE(5,(#24385,#24386,#24387,#24388,#24389,#24390,#24391,#24392,
#24393,#24394,#24395,#24396,#24397,#24398,#24399,#24400,#24401,#24402,#24403,
#24404,#24405,#24406,#24407,#24408,#24409,#24410,#24411,#24412,#24413,#24414,
#24415,#24416,#24417,#24418,#24419,#24420,#24421,#24422,#24423,#24424,#24425,
#24426,#24427,#24428,#24429,#24430,#24431,#24432,#24433,#24434,#24435,#24436,
#24437,#24438,#24439,#24440,#24441,#24442,#24443,#24444,#24445,#24446,#24447,
#24448,#24449,#24450,#24451,#24452,#24453,#24454),.UNSPECIFIED.,.F.,.F.)
B_SPLINE_CURVE_WITH_KNOTS((6,1,1,1,1,1,1,1,1,1,1,1,1,1,1,1,1,1,1,1,1,1,
1,1,1,1,1,1,1,1,1,1,1,1,1,1,1,1,1,1,1,1,1,1,1,1,1,1,1,1,1,1,1,1,1,1,1,1,
1,1,1,1,1,1,1,6),(0.,0.0153846153846154,0.0307692307692308,0.0461538461538462,
0.0615384615384615,0.0769230769230769,0.0923076923076923,0.107692307692308,
0.123076923076923,0.138461538461538,0.153846153846154,0.169230769230769,
0.184615384615385,0.2,0.215384615384615,0.230769230769231,0.246153846153846,
0.261538461538462,0.276923076923077,0.292307692307692,0.307692307692308,
0.323076923076923,0.338461538461538,0.353846153846154,0.369230769230769,
0.384615384615385,0.4,0.415384615384615,0.430769230769231,0.446153846153846,
0.461538461538462,0.476923076923077,0.492307692307692,0.507692307692308,
0.523076923076923,0.538461538461538,0.553846153846154,0.569230769230769,
0.584615384615384,0.6,0.615384615384615,0.63076923076923,0.646153846153846,
0.661538461538461,0.676923076923076,0.692307692307692,0.707692307692307,
0.723076923076922,0.738461538461538,0.753846153846153,0.769230769230768,
0.784615384615384,0.799999999999999,0.815384615384614,0.83076923076923,
0.846153846153845,0.86153846153846,0.876923076923076,0.892307692307691,
0.907692307692306,0.923076923076922,0.938461538461537,0.953846153846152,
0.969230769230768,0.984615384615383,1.),.UNSPECIFIED.)
CURVE()
GEOMETRIC_REPRESENTATION_ITEM()
RATIONAL_B_SPLINE_CURVE((1.,1.,1.,1.,1.,1.,1.,1.,1.,1.,1.,1.,1.,1.,1.,1.,
1.,1.,1.,1.,1.,1.,1.,1.,1.,1.,1.,1.,1.,1.,1.,1.,1.,1.,1.,1.,1.,1.,1.,1.,
1.,1.,1.,1.,1.,1.,1.,1.,1.,1.,1.,1.,1.,1.,1.,1.,1.,1.,1.,1.,1.,1.,1.,1.,
1.,1.,1.,1.,1.,1.))
REPRESENTATION_ITEM('')
);
#73=(
BOUNDED_CURVE()
B_SPLINE_CURVE(5,(#24458,#24459,#24460,#24461,#24462,#24463,#24464,#24465,
#24466,#24467,#24468,#24469,#24470,#24471,#24472,#24473,#24474,#24475,#24476,
#24477,#24478,#24479,#24480,#24481,#24482,#24483,#24484,#24485,#24486,#24487,
#24488,#24489,#24490,#24491,#24492,#24493,#24494,#24495,#24496,#24497,#24498,
#24499,#24500,#24501,#24502,#24503,#24504,#24505,#24506,#24507,#24508,#24509,
#24510,#24511,#24512,#24513,#24514,#24515,#24516,#24517,#24518,#24519,#24520,
#24521,#24522,#24523,#24524,#24525,#24526,#24527),.UNSPECIFIED.,.F.,.F.)
B_SPLINE_CURVE_WITH_KNOTS((6,1,1,1,1,1,1,1,1,1,1,1,1,1,1,1,1,1,1,1,1,1,
1,1,1,1,1,1,1,1,1,1,1,1,1,1,1,1,1,1,1,1,1,1,1,1,1,1,1,1,1,1,1,1,1,1,1,1,
1,1,1,1,1,1,1,6),(0.,0.0153846153846154,0.0307692307692308,0.0461538461538462,
0.0615384615384615,0.0769230769230769,0.0923076923076923,0.107692307692308,
0.123076923076923,0.138461538461538,0.153846153846154,0.169230769230769,
0.184615384615385,0.2,0.215384615384615,0.230769230769231,0.246153846153846,
0.261538461538462,0.276923076923077,0.292307692307692,0.307692307692308,
0.323076923076923,0.338461538461538,0.353846153846154,0.369230769230769,
0.384615384615385,0.4,0.415384615384615,0.430769230769231,0.446153846153846,
0.461538461538462,0.476923076923077,0.492307692307692,0.507692307692308,
0.523076923076923,0.538461538461538,0.553846153846154,0.569230769230769,
0.584615384615384,0.6,0.615384615384615,0.63076923076923,0.646153846153846,
0.661538461538461,0.676923076923076,0.692307692307692,0.707692307692307,
0.723076923076922,0.738461538461538,0.753846153846153,0.769230769230768,
0.784615384615384,0.799999999999999,0.815384615384614,0.83076923076923,
0.846153846153845,0.86153846153846,0.876923076923076,0.892307692307691,
0.907692307692306,0.923076923076922,0.938461538461537,0.953846153846152,
0.969230769230768,0.984615384615383,1.),.UNSPECIFIED.)
CURVE()
GEOMETRIC_REPRESENTATION_ITEM()
RATIONAL_B_SPLINE_CURVE((1.,1.,1.,1.,1.,1.,1.,1.,1.,1.,1.,1.,1.,1.,1.,1.,
1.,1.,1.,1.,1.,1.,1.,1.,1.,1.,1.,1.,1.,1.,1.,1.,1.,1.,1.,1.,1.,1.,1.,1.,
1.,1.,1.,1.,1.,1.,1.,1.,1.,1.,1.,1.,1.,1.,1.,1.,1.,1.,1.,1.,1.,1.,1.,1.,
1.,1.,1.,1.,1.,1.))
REPRESENTATION_ITEM('')
);
#74=(
BOUNDED_CURVE()
B_SPLINE_CURVE(5,(#24531,#24532,#24533,#24534,#24535,#24536,#24537,#24538,
#24539,#24540,#24541,#24542,#24543,#24544,#24545,#24546,#24547,#24548,#24549,
#24550,#24551,#24552,#24553,#24554,#24555,#24556,#24557,#24558,#24559,#24560,
#24561,#24562,#24563,#24564,#24565,#24566,#24567,#24568,#24569,#24570,#24571,
#24572,#24573,#24574,#24575,#24576,#24577,#24578,#24579,#24580,#24581,#24582,
#24583,#24584,#24585,#24586,#24587,#24588,#24589,#24590,#24591,#24592,#24593,
#24594,#24595,#24596,#24597,#24598,#24599,#24600),.UNSPECIFIED.,.F.,.F.)
B_SPLINE_CURVE_WITH_KNOTS((6,1,1,1,1,1,1,1,1,1,1,1,1,1,1,1,1,1,1,1,1,1,
1,1,1,1,1,1,1,1,1,1,1,1,1,1,1,1,1,1,1,1,1,1,1,1,1,1,1,1,1,1,1,1,1,1,1,1,
1,1,1,1,1,1,1,6),(0.,0.0153846153846154,0.0307692307692308,0.0461538461538462,
0.0615384615384615,0.0769230769230769,0.0923076923076923,0.107692307692308,
0.123076923076923,0.138461538461538,0.153846153846154,0.169230769230769,
0.184615384615385,0.2,0.215384615384615,0.230769230769231,0.246153846153846,
0.261538461538462,0.276923076923077,0.292307692307692,0.307692307692308,
0.323076923076923,0.338461538461538,0.353846153846154,0.369230769230769,
0.384615384615385,0.4,0.415384615384615,0.430769230769231,0.446153846153846,
0.461538461538462,0.476923076923077,0.492307692307692,0.507692307692308,
0.523076923076923,0.538461538461538,0.553846153846154,0.569230769230769,
0.584615384615384,0.6,0.615384615384615,0.63076923076923,0.646153846153846,
0.661538461538461,0.676923076923076,0.692307692307692,0.707692307692307,
0.723076923076922,0.738461538461538,0.753846153846153,0.769230769230768,
0.784615384615384,0.799999999999999,0.815384615384614,0.83076923076923,
0.846153846153845,0.86153846153846,0.876923076923076,0.892307692307691,
0.907692307692306,0.923076923076922,0.938461538461537,0.953846153846152,
0.969230769230768,0.984615384615383,1.),.UNSPECIFIED.)
CURVE()
GEOMETRIC_REPRESENTATION_ITEM()
RATIONAL_B_SPLINE_CURVE((1.,1.,1.,1.,1.,1.,1.,1.,1.,1.,1.,1.,1.,1.,1.,1.,
1.,1.,1.,1.,1.,1.,1.,1.,1.,1.,1.,1.,1.,1.,1.,1.,1.,1.,1.,1.,1.,1.,1.,1.,
1.,1.,1.,1.,1.,1.,1.,1.,1.,1.,1.,1.,1.,1.,1.,1.,1.,1.,1.,1.,1.,1.,1.,1.,
1.,1.,1.,1.,1.,1.))
REPRESENTATION_ITEM('')
);
#75=(
BOUNDED_CURVE()
B_SPLINE_CURVE(5,(#24604,#24605,#24606,#24607,#24608,#24609,#24610,#24611,
#24612,#24613,#24614,#24615,#24616,#24617,#24618,#24619,#24620,#24621,#24622,
#24623,#24624,#24625,#24626,#24627,#24628,#24629,#24630,#24631,#24632,#24633,
#24634,#24635,#24636,#24637,#24638,#24639,#24640,#24641,#24642,#24643,#24644,
#24645,#24646,#24647,#24648,#24649,#24650,#24651,#24652,#24653,#24654,#24655,
#24656,#24657,#24658,#24659,#24660,#24661,#24662,#24663,#24664,#24665,#24666,
#24667,#24668,#24669,#24670,#24671,#24672,#24673),.UNSPECIFIED.,.F.,.F.)
B_SPLINE_CURVE_WITH_KNOTS((6,1,1,1,1,1,1,1,1,1,1,1,1,1,1,1,1,1,1,1,1,1,
1,1,1,1,1,1,1,1,1,1,1,1,1,1,1,1,1,1,1,1,1,1,1,1,1,1,1,1,1,1,1,1,1,1,1,1,
1,1,1,1,1,1,1,6),(0.,0.0153846153846154,0.0307692307692308,0.0461538461538462,
0.0615384615384615,0.0769230769230769,0.0923076923076923,0.107692307692308,
0.123076923076923,0.138461538461538,0.153846153846154,0.169230769230769,
0.184615384615385,0.2,0.215384615384615,0.230769230769231,0.246153846153846,
0.261538461538462,0.276923076923077,0.292307692307692,0.307692307692308,
0.323076923076923,0.338461538461538,0.353846153846154,0.369230769230769,
0.384615384615385,0.4,0.415384615384615,0.430769230769231,0.446153846153846,
0.461538461538462,0.476923076923077,0.492307692307692,0.507692307692308,
0.523076923076923,0.538461538461538,0.553846153846154,0.569230769230769,
0.584615384615384,0.6,0.615384615384615,0.63076923076923,0.646153846153846,
0.661538461538461,0.676923076923076,0.692307692307692,0.707692307692307,
0.723076923076922,0.738461538461538,0.753846153846153,0.769230769230768,
0.784615384615384,0.799999999999999,0.815384615384614,0.83076923076923,
0.846153846153845,0.86153846153846,0.876923076923076,0.892307692307691,
0.907692307692306,0.923076923076922,0.938461538461537,0.953846153846152,
0.969230769230768,0.984615384615383,1.),.UNSPECIFIED.)
CURVE()
GEOMETRIC_REPRESENTATION_ITEM()
RATIONAL_B_SPLINE_CURVE((1.,1.,1.,1.,1.,1.,1.,1.,1.,1.,1.,1.,1.,1.,1.,1.,
1.,1.,1.,1.,1.,1.,1.,1.,1.,1.,1.,1.,1.,1.,1.,1.,1.,1.,1.,1.,1.,1.,1.,1.,
1.,1.,1.,1.,1.,1.,1.,1.,1.,1.,1.,1.,1.,1.,1.,1.,1.,1.,1.,1.,1.,1.,1.,1.,
1.,1.,1.,1.,1.,1.))
REPRESENTATION_ITEM('')
);
#76=(
BOUNDED_CURVE()
B_SPLINE_CURVE(5,(#24677,#24678,#24679,#24680,#24681,#24682,#24683,#24684,
#24685,#24686,#24687,#24688,#24689,#24690,#24691,#24692,#24693,#24694,#24695,
#24696,#24697,#24698,#24699,#24700,#24701,#24702,#24703,#24704,#24705,#24706,
#24707,#24708,#24709,#24710,#24711,#24712,#24713,#24714,#24715,#24716,#24717,
#24718,#24719,#24720,#24721,#24722,#24723,#24724,#24725,#24726,#24727,#24728,
#24729,#24730,#24731,#24732,#24733,#24734,#24735,#24736,#24737,#24738,#24739,
#24740,#24741,#24742,#24743,#24744,#24745,#24746),.UNSPECIFIED.,.F.,.F.)
B_SPLINE_CURVE_WITH_KNOTS((6,1,1,1,1,1,1,1,1,1,1,1,1,1,1,1,1,1,1,1,1,1,
1,1,1,1,1,1,1,1,1,1,1,1,1,1,1,1,1,1,1,1,1,1,1,1,1,1,1,1,1,1,1,1,1,1,1,1,
1,1,1,1,1,1,1,6),(0.,0.0153846153846154,0.0307692307692308,0.0461538461538462,
0.0615384615384615,0.0769230769230769,0.0923076923076923,0.107692307692308,
0.123076923076923,0.138461538461538,0.153846153846154,0.169230769230769,
0.184615384615385,0.2,0.215384615384615,0.230769230769231,0.246153846153846,
0.261538461538462,0.276923076923077,0.292307692307692,0.307692307692308,
0.323076923076923,0.338461538461538,0.353846153846154,0.369230769230769,
0.384615384615385,0.4,0.415384615384615,0.430769230769231,0.446153846153846,
0.461538461538462,0.476923076923077,0.492307692307692,0.507692307692308,
0.523076923076923,0.538461538461538,0.553846153846154,0.569230769230769,
0.584615384615384,0.6,0.615384615384615,0.63076923076923,0.646153846153846,
0.661538461538461,0.676923076923076,0.692307692307692,0.707692307692307,
0.723076923076922,0.738461538461538,0.753846153846153,0.769230769230768,
0.784615384615384,0.799999999999999,0.815384615384614,0.83076923076923,
0.846153846153845,0.86153846153846,0.876923076923076,0.892307692307691,
0.907692307692306,0.923076923076922,0.938461538461537,0.953846153846152,
0.969230769230768,0.984615384615383,1.),.UNSPECIFIED.)
CURVE()
GEOMETRIC_REPRESENTATION_ITEM()
RATIONAL_B_SPLINE_CURVE((1.,1.,1.,1.,1.,1.,1.,1.,1.,1.,1.,1.,1.,1.,1.,1.,
1.,1.,1.,1.,1.,1.,1.,1.,1.,1.,1.,1.,1.,1.,1.,1.,1.,1.,1.,1.,1.,1.,1.,1.,
1.,1.,1.,1.,1.,1.,1.,1.,1.,1.,1.,1.,1.,1.,1.,1.,1.,1.,1.,1.,1.,1.,1.,1.,
1.,1.,1.,1.,1.,1.))
REPRESENTATION_ITEM('')
);
#77=(
BOUNDED_CURVE()
B_SPLINE_CURVE(5,(#24750,#24751,#24752,#24753,#24754,#24755,#24756,#24757,
#24758,#24759,#24760,#24761,#24762,#24763,#24764,#24765,#24766,#24767,#24768,
#24769,#24770,#24771,#24772,#24773,#24774,#24775,#24776,#24777,#24778,#24779,
#24780,#24781,#24782,#24783,#24784,#24785,#24786,#24787,#24788,#24789,#24790,
#24791,#24792,#24793,#24794,#24795,#24796,#24797,#24798,#24799,#24800,#24801,
#24802,#24803,#24804,#24805,#24806,#24807,#24808,#24809,#24810,#24811,#24812,
#24813,#24814,#24815,#24816,#24817,#24818,#24819),.UNSPECIFIED.,.F.,.F.)
B_SPLINE_CURVE_WITH_KNOTS((6,1,1,1,1,1,1,1,1,1,1,1,1,1,1,1,1,1,1,1,1,1,
1,1,1,1,1,1,1,1,1,1,1,1,1,1,1,1,1,1,1,1,1,1,1,1,1,1,1,1,1,1,1,1,1,1,1,1,
1,1,1,1,1,1,1,6),(0.,0.0153846153846154,0.0307692307692308,0.0461538461538462,
0.0615384615384615,0.0769230769230769,0.0923076923076923,0.107692307692308,
0.123076923076923,0.138461538461538,0.153846153846154,0.169230769230769,
0.184615384615385,0.2,0.215384615384615,0.230769230769231,0.246153846153846,
0.261538461538462,0.276923076923077,0.292307692307692,0.307692307692308,
0.323076923076923,0.338461538461538,0.353846153846154,0.369230769230769,
0.384615384615385,0.4,0.415384615384615,0.430769230769231,0.446153846153846,
0.461538461538462,0.476923076923077,0.492307692307692,0.507692307692308,
0.523076923076923,0.538461538461538,0.553846153846154,0.569230769230769,
0.584615384615384,0.6,0.615384615384615,0.63076923076923,0.646153846153846,
0.661538461538461,0.676923076923076,0.692307692307692,0.707692307692307,
0.723076923076922,0.738461538461538,0.753846153846153,0.769230769230768,
0.784615384615384,0.799999999999999,0.815384615384614,0.83076923076923,
0.846153846153845,0.86153846153846,0.876923076923076,0.892307692307691,
0.907692307692306,0.923076923076922,0.938461538461537,0.953846153846152,
0.969230769230768,0.984615384615383,1.),.UNSPECIFIED.)
CURVE()
GEOMETRIC_REPRESENTATION_ITEM()
RATIONAL_B_SPLINE_CURVE((1.,1.,1.,1.,1.,1.,1.,1.,1.,1.,1.,1.,1.,1.,1.,1.,
1.,1.,1.,1.,1.,1.,1.,1.,1.,1.,1.,1.,1.,1.,1.,1.,1.,1.,1.,1.,1.,1.,1.,1.,
1.,1.,1.,1.,1.,1.,1.,1.,1.,1.,1.,1.,1.,1.,1.,1.,1.,1.,1.,1.,1.,1.,1.,1.,
1.,1.,1.,1.,1.,1.))
REPRESENTATION_ITEM('')
);
#78=(
BOUNDED_CURVE()
B_SPLINE_CURVE(5,(#24823,#24824,#24825,#24826,#24827,#24828,#24829,#24830,
#24831,#24832,#24833,#24834,#24835,#24836,#24837,#24838,#24839,#24840,#24841,
#24842,#24843,#24844,#24845,#24846,#24847,#24848,#24849,#24850,#24851,#24852,
#24853,#24854,#24855,#24856,#24857,#24858,#24859,#24860,#24861,#24862,#24863,
#24864,#24865,#24866,#24867,#24868,#24869,#24870,#24871,#24872,#24873,#24874,
#24875,#24876,#24877,#24878,#24879,#24880,#24881,#24882,#24883,#24884,#24885,
#24886,#24887,#24888,#24889,#24890,#24891,#24892),.UNSPECIFIED.,.F.,.F.)
B_SPLINE_CURVE_WITH_KNOTS((6,1,1,1,1,1,1,1,1,1,1,1,1,1,1,1,1,1,1,1,1,1,
1,1,1,1,1,1,1,1,1,1,1,1,1,1,1,1,1,1,1,1,1,1,1,1,1,1,1,1,1,1,1,1,1,1,1,1,
1,1,1,1,1,1,1,6),(0.,0.0153846153846154,0.0307692307692308,0.0461538461538462,
0.0615384615384615,0.0769230769230769,0.0923076923076923,0.107692307692308,
0.123076923076923,0.138461538461538,0.153846153846154,0.169230769230769,
0.184615384615385,0.2,0.215384615384615,0.230769230769231,0.246153846153846,
0.261538461538462,0.276923076923077,0.292307692307692,0.307692307692308,
0.323076923076923,0.338461538461538,0.353846153846154,0.369230769230769,
0.384615384615385,0.4,0.415384615384615,0.430769230769231,0.446153846153846,
0.461538461538462,0.476923076923077,0.492307692307692,0.507692307692308,
0.523076923076923,0.538461538461538,0.553846153846154,0.569230769230769,
0.584615384615384,0.6,0.615384615384615,0.63076923076923,0.646153846153846,
0.661538461538461,0.676923076923076,0.692307692307692,0.707692307692307,
0.723076923076922,0.738461538461538,0.753846153846153,0.769230769230768,
0.784615384615384,0.799999999999999,0.815384615384614,0.83076923076923,
0.846153846153845,0.86153846153846,0.876923076923076,0.892307692307691,
0.907692307692306,0.923076923076922,0.938461538461537,0.953846153846152,
0.969230769230768,0.984615384615383,1.),.UNSPECIFIED.)
CURVE()
GEOMETRIC_REPRESENTATION_ITEM()
RATIONAL_B_SPLINE_CURVE((1.,1.,1.,1.,1.,1.,1.,1.,1.,1.,1.,1.,1.,1.,1.,1.,
1.,1.,1.,1.,1.,1.,1.,1.,1.,1.,1.,1.,1.,1.,1.,1.,1.,1.,1.,1.,1.,1.,1.,1.,
1.,1.,1.,1.,1.,1.,1.,1.,1.,1.,1.,1.,1.,1.,1.,1.,1.,1.,1.,1.,1.,1.,1.,1.,
1.,1.,1.,1.,1.,1.))
REPRESENTATION_ITEM('')
);
#79=(
BOUNDED_CURVE()
B_SPLINE_CURVE(5,(#24896,#24897,#24898,#24899,#24900,#24901,#24902,#24903,
#24904,#24905,#24906,#24907,#24908,#24909,#24910,#24911,#24912,#24913,#24914,
#24915,#24916,#24917,#24918,#24919,#24920,#24921,#24922,#24923,#24924,#24925,
#24926,#24927,#24928,#24929,#24930,#24931,#24932,#24933,#24934,#24935,#24936,
#24937,#24938,#24939,#24940,#24941,#24942,#24943,#24944,#24945,#24946,#24947,
#24948,#24949,#24950,#24951,#24952,#24953,#24954,#24955,#24956,#24957,#24958,
#24959,#24960,#24961,#24962,#24963,#24964,#24965),.UNSPECIFIED.,.F.,.F.)
B_SPLINE_CURVE_WITH_KNOTS((6,1,1,1,1,1,1,1,1,1,1,1,1,1,1,1,1,1,1,1,1,1,
1,1,1,1,1,1,1,1,1,1,1,1,1,1,1,1,1,1,1,1,1,1,1,1,1,1,1,1,1,1,1,1,1,1,1,1,
1,1,1,1,1,1,1,6),(0.,0.0153846153846154,0.0307692307692308,0.0461538461538462,
0.0615384615384615,0.0769230769230769,0.0923076923076923,0.107692307692308,
0.123076923076923,0.138461538461538,0.153846153846154,0.169230769230769,
0.184615384615385,0.2,0.215384615384615,0.230769230769231,0.246153846153846,
0.261538461538462,0.276923076923077,0.292307692307692,0.307692307692308,
0.323076923076923,0.338461538461538,0.353846153846154,0.369230769230769,
0.384615384615385,0.4,0.415384615384615,0.430769230769231,0.446153846153846,
0.461538461538462,0.476923076923077,0.492307692307692,0.507692307692308,
0.523076923076923,0.538461538461538,0.553846153846154,0.569230769230769,
0.584615384615384,0.6,0.615384615384615,0.63076923076923,0.646153846153846,
0.661538461538461,0.676923076923076,0.692307692307692,0.707692307692307,
0.723076923076922,0.738461538461538,0.753846153846153,0.769230769230768,
0.784615384615384,0.799999999999999,0.815384615384614,0.83076923076923,
0.846153846153845,0.86153846153846,0.876923076923076,0.892307692307691,
0.907692307692306,0.923076923076922,0.938461538461537,0.953846153846152,
0.969230769230768,0.984615384615383,1.),.UNSPECIFIED.)
CURVE()
GEOMETRIC_REPRESENTATION_ITEM()
RATIONAL_B_SPLINE_CURVE((1.,1.,1.,1.,1.,1.,1.,1.,1.,1.,1.,1.,1.,1.,1.,1.,
1.,1.,1.,1.,1.,1.,1.,1.,1.,1.,1.,1.,1.,1.,1.,1.,1.,1.,1.,1.,1.,1.,1.,1.,
1.,1.,1.,1.,1.,1.,1.,1.,1.,1.,1.,1.,1.,1.,1.,1.,1.,1.,1.,1.,1.,1.,1.,1.,
1.,1.,1.,1.,1.,1.))
REPRESENTATION_ITEM('')
);
#80=(
BOUNDED_CURVE()
B_SPLINE_CURVE(5,(#24969,#24970,#24971,#24972,#24973,#24974,#24975,#24976,
#24977,#24978,#24979,#24980,#24981,#24982,#24983,#24984,#24985,#24986,#24987,
#24988,#24989,#24990,#24991,#24992,#24993,#24994,#24995,#24996,#24997,#24998,
#24999,#25000,#25001,#25002,#25003,#25004,#25005,#25006,#25007,#25008,#25009,
#25010,#25011,#25012,#25013,#25014,#25015,#25016,#25017,#25018,#25019,#25020,
#25021,#25022,#25023,#25024,#25025,#25026,#25027,#25028,#25029,#25030,#25031,
#25032,#25033,#25034,#25035,#25036,#25037,#25038),.UNSPECIFIED.,.F.,.F.)
B_SPLINE_CURVE_WITH_KNOTS((6,1,1,1,1,1,1,1,1,1,1,1,1,1,1,1,1,1,1,1,1,1,
1,1,1,1,1,1,1,1,1,1,1,1,1,1,1,1,1,1,1,1,1,1,1,1,1,1,1,1,1,1,1,1,1,1,1,1,
1,1,1,1,1,1,1,6),(0.,0.0153846153846154,0.0307692307692308,0.0461538461538462,
0.0615384615384615,0.0769230769230769,0.0923076923076923,0.107692307692308,
0.123076923076923,0.138461538461538,0.153846153846154,0.169230769230769,
0.184615384615385,0.2,0.215384615384615,0.230769230769231,0.246153846153846,
0.261538461538462,0.276923076923077,0.292307692307692,0.307692307692308,
0.323076923076923,0.338461538461538,0.353846153846154,0.369230769230769,
0.384615384615385,0.4,0.415384615384615,0.430769230769231,0.446153846153846,
0.461538461538462,0.476923076923077,0.492307692307692,0.507692307692308,
0.523076923076923,0.538461538461538,0.553846153846154,0.569230769230769,
0.584615384615384,0.6,0.615384615384615,0.63076923076923,0.646153846153846,
0.661538461538461,0.676923076923076,0.692307692307692,0.707692307692307,
0.723076923076922,0.738461538461538,0.753846153846153,0.769230769230768,
0.784615384615384,0.799999999999999,0.815384615384614,0.83076923076923,
0.846153846153845,0.86153846153846,0.876923076923076,0.892307692307691,
0.907692307692306,0.923076923076922,0.938461538461537,0.953846153846152,
0.969230769230768,0.984615384615383,1.),.UNSPECIFIED.)
CURVE()
GEOMETRIC_REPRESENTATION_ITEM()
RATIONAL_B_SPLINE_CURVE((1.,1.,1.,1.,1.,1.,1.,1.,1.,1.,1.,1.,1.,1.,1.,1.,
1.,1.,1.,1.,1.,1.,1.,1.,1.,1.,1.,1.,1.,1.,1.,1.,1.,1.,1.,1.,1.,1.,1.,1.,
1.,1.,1.,1.,1.,1.,1.,1.,1.,1.,1.,1.,1.,1.,1.,1.,1.,1.,1.,1.,1.,1.,1.,1.,
1.,1.,1.,1.,1.,1.))
REPRESENTATION_ITEM('')
);
#81=(
BOUNDED_CURVE()
B_SPLINE_CURVE(5,(#25042,#25043,#25044,#25045,#25046,#25047,#25048,#25049,
#25050,#25051,#25052,#25053,#25054,#25055,#25056,#25057,#25058,#25059,#25060,
#25061,#25062,#25063,#25064,#25065,#25066,#25067,#25068,#25069,#25070,#25071,
#25072,#25073,#25074,#25075,#25076,#25077,#25078,#25079,#25080,#25081,#25082,
#25083,#25084,#25085,#25086,#25087,#25088,#25089,#25090,#25091,#25092,#25093,
#25094,#25095,#25096,#25097,#25098,#25099,#25100,#25101,#25102,#25103,#25104,
#25105,#25106,#25107,#25108,#25109,#25110,#25111),.UNSPECIFIED.,.F.,.F.)
B_SPLINE_CURVE_WITH_KNOTS((6,1,1,1,1,1,1,1,1,1,1,1,1,1,1,1,1,1,1,1,1,1,
1,1,1,1,1,1,1,1,1,1,1,1,1,1,1,1,1,1,1,1,1,1,1,1,1,1,1,1,1,1,1,1,1,1,1,1,
1,1,1,1,1,1,1,6),(0.,0.0153846153846154,0.0307692307692308,0.0461538461538462,
0.0615384615384615,0.0769230769230769,0.0923076923076923,0.107692307692308,
0.123076923076923,0.138461538461538,0.153846153846154,0.169230769230769,
0.184615384615385,0.2,0.215384615384615,0.230769230769231,0.246153846153846,
0.261538461538462,0.276923076923077,0.292307692307692,0.307692307692308,
0.323076923076923,0.338461538461538,0.353846153846154,0.369230769230769,
0.384615384615385,0.4,0.415384615384615,0.430769230769231,0.446153846153846,
0.461538461538462,0.476923076923077,0.492307692307692,0.507692307692308,
0.523076923076923,0.538461538461538,0.553846153846154,0.569230769230769,
0.584615384615384,0.6,0.615384615384615,0.63076923076923,0.646153846153846,
0.661538461538461,0.676923076923076,0.692307692307692,0.707692307692307,
0.723076923076922,0.738461538461538,0.753846153846153,0.769230769230768,
0.784615384615384,0.799999999999999,0.815384615384614,0.83076923076923,
0.846153846153845,0.86153846153846,0.876923076923076,0.892307692307691,
0.907692307692306,0.923076923076922,0.938461538461537,0.953846153846152,
0.969230769230768,0.984615384615383,1.),.UNSPECIFIED.)
CURVE()
GEOMETRIC_REPRESENTATION_ITEM()
RATIONAL_B_SPLINE_CURVE((1.,1.,1.,1.,1.,1.,1.,1.,1.,1.,1.,1.,1.,1.,1.,1.,
1.,1.,1.,1.,1.,1.,1.,1.,1.,1.,1.,1.,1.,1.,1.,1.,1.,1.,1.,1.,1.,1.,1.,1.,
1.,1.,1.,1.,1.,1.,1.,1.,1.,1.,1.,1.,1.,1.,1.,1.,1.,1.,1.,1.,1.,1.,1.,1.,
1.,1.,1.,1.,1.,1.))
REPRESENTATION_ITEM('')
);
#82=(
BOUNDED_CURVE()
B_SPLINE_CURVE(5,(#25115,#25116,#25117,#25118,#25119,#25120,#25121,#25122,
#25123,#25124,#25125,#25126,#25127,#25128,#25129,#25130,#25131,#25132,#25133,
#25134,#25135,#25136,#25137,#25138,#25139,#25140,#25141,#25142,#25143,#25144,
#25145,#25146,#25147,#25148,#25149,#25150,#25151,#25152,#25153,#25154,#25155,
#25156,#25157,#25158,#25159,#25160,#25161,#25162,#25163,#25164,#25165,#25166,
#25167,#25168,#25169,#25170,#25171,#25172,#25173,#25174,#25175,#25176,#25177,
#25178,#25179,#25180,#25181,#25182,#25183,#25184),.UNSPECIFIED.,.F.,.F.)
B_SPLINE_CURVE_WITH_KNOTS((6,1,1,1,1,1,1,1,1,1,1,1,1,1,1,1,1,1,1,1,1,1,
1,1,1,1,1,1,1,1,1,1,1,1,1,1,1,1,1,1,1,1,1,1,1,1,1,1,1,1,1,1,1,1,1,1,1,1,
1,1,1,1,1,1,1,6),(0.,0.0153846153846154,0.0307692307692308,0.0461538461538462,
0.0615384615384615,0.0769230769230769,0.0923076923076923,0.107692307692308,
0.123076923076923,0.138461538461538,0.153846153846154,0.169230769230769,
0.184615384615385,0.2,0.215384615384615,0.230769230769231,0.246153846153846,
0.261538461538462,0.276923076923077,0.292307692307692,0.307692307692308,
0.323076923076923,0.338461538461538,0.353846153846154,0.369230769230769,
0.384615384615385,0.4,0.415384615384615,0.430769230769231,0.446153846153846,
0.461538461538462,0.476923076923077,0.492307692307692,0.507692307692308,
0.523076923076923,0.538461538461538,0.553846153846154,0.569230769230769,
0.584615384615384,0.6,0.615384615384615,0.63076923076923,0.646153846153846,
0.661538461538461,0.676923076923076,0.692307692307692,0.707692307692307,
0.723076923076922,0.738461538461538,0.753846153846153,0.769230769230768,
0.784615384615384,0.799999999999999,0.815384615384614,0.83076923076923,
0.846153846153845,0.86153846153846,0.876923076923076,0.892307692307691,
0.907692307692306,0.923076923076922,0.938461538461537,0.953846153846152,
0.969230769230768,0.984615384615383,1.),.UNSPECIFIED.)
CURVE()
GEOMETRIC_REPRESENTATION_ITEM()
RATIONAL_B_SPLINE_CURVE((1.,1.,1.,1.,1.,1.,1.,1.,1.,1.,1.,1.,1.,1.,1.,1.,
1.,1.,1.,1.,1.,1.,1.,1.,1.,1.,1.,1.,1.,1.,1.,1.,1.,1.,1.,1.,1.,1.,1.,1.,
1.,1.,1.,1.,1.,1.,1.,1.,1.,1.,1.,1.,1.,1.,1.,1.,1.,1.,1.,1.,1.,1.,1.,1.,
1.,1.,1.,1.,1.,1.))
REPRESENTATION_ITEM('')
);
#83=(
BOUNDED_CURVE()
B_SPLINE_CURVE(5,(#25188,#25189,#25190,#25191,#25192,#25193,#25194,#25195,
#25196,#25197,#25198,#25199,#25200,#25201,#25202,#25203,#25204,#25205,#25206,
#25207,#25208,#25209,#25210,#25211,#25212,#25213,#25214,#25215,#25216,#25217,
#25218,#25219,#25220,#25221,#25222,#25223,#25224,#25225,#25226,#25227,#25228,
#25229,#25230,#25231,#25232,#25233,#25234,#25235,#25236,#25237,#25238,#25239,
#25240,#25241,#25242,#25243,#25244,#25245,#25246,#25247,#25248,#25249,#25250,
#25251,#25252,#25253,#25254,#25255,#25256,#25257),.UNSPECIFIED.,.F.,.F.)
B_SPLINE_CURVE_WITH_KNOTS((6,1,1,1,1,1,1,1,1,1,1,1,1,1,1,1,1,1,1,1,1,1,
1,1,1,1,1,1,1,1,1,1,1,1,1,1,1,1,1,1,1,1,1,1,1,1,1,1,1,1,1,1,1,1,1,1,1,1,
1,1,1,1,1,1,1,6),(0.,0.0153846153846154,0.0307692307692308,0.0461538461538462,
0.0615384615384615,0.0769230769230769,0.0923076923076923,0.107692307692308,
0.123076923076923,0.138461538461538,0.153846153846154,0.169230769230769,
0.184615384615385,0.2,0.215384615384615,0.230769230769231,0.246153846153846,
0.261538461538462,0.276923076923077,0.292307692307692,0.307692307692308,
0.323076923076923,0.338461538461538,0.353846153846154,0.369230769230769,
0.384615384615385,0.4,0.415384615384615,0.430769230769231,0.446153846153846,
0.461538461538462,0.476923076923077,0.492307692307692,0.507692307692308,
0.523076923076923,0.538461538461538,0.553846153846154,0.569230769230769,
0.584615384615384,0.6,0.615384615384615,0.63076923076923,0.646153846153846,
0.661538461538461,0.676923076923076,0.692307692307692,0.707692307692307,
0.723076923076922,0.738461538461538,0.753846153846153,0.769230769230768,
0.784615384615384,0.799999999999999,0.815384615384614,0.83076923076923,
0.846153846153845,0.86153846153846,0.876923076923076,0.892307692307691,
0.907692307692306,0.923076923076922,0.938461538461537,0.953846153846152,
0.969230769230768,0.984615384615383,1.),.UNSPECIFIED.)
CURVE()
GEOMETRIC_REPRESENTATION_ITEM()
RATIONAL_B_SPLINE_CURVE((1.,1.,1.,1.,1.,1.,1.,1.,1.,1.,1.,1.,1.,1.,1.,1.,
1.,1.,1.,1.,1.,1.,1.,1.,1.,1.,1.,1.,1.,1.,1.,1.,1.,1.,1.,1.,1.,1.,1.,1.,
1.,1.,1.,1.,1.,1.,1.,1.,1.,1.,1.,1.,1.,1.,1.,1.,1.,1.,1.,1.,1.,1.,1.,1.,
1.,1.,1.,1.,1.,1.))
REPRESENTATION_ITEM('')
);
#84=(
BOUNDED_CURVE()
B_SPLINE_CURVE(5,(#25261,#25262,#25263,#25264,#25265,#25266,#25267,#25268,
#25269,#25270,#25271,#25272,#25273,#25274,#25275,#25276,#25277,#25278,#25279,
#25280,#25281,#25282,#25283,#25284,#25285,#25286,#25287,#25288,#25289,#25290,
#25291,#25292,#25293,#25294,#25295,#25296,#25297,#25298,#25299,#25300,#25301,
#25302,#25303,#25304,#25305,#25306,#25307,#25308,#25309,#25310,#25311,#25312,
#25313,#25314,#25315,#25316,#25317,#25318,#25319,#25320,#25321,#25322,#25323,
#25324,#25325,#25326,#25327,#25328,#25329,#25330),.UNSPECIFIED.,.F.,.F.)
B_SPLINE_CURVE_WITH_KNOTS((6,1,1,1,1,1,1,1,1,1,1,1,1,1,1,1,1,1,1,1,1,1,
1,1,1,1,1,1,1,1,1,1,1,1,1,1,1,1,1,1,1,1,1,1,1,1,1,1,1,1,1,1,1,1,1,1,1,1,
1,1,1,1,1,1,1,6),(0.,0.0153846153846154,0.0307692307692308,0.0461538461538462,
0.0615384615384615,0.0769230769230769,0.0923076923076923,0.107692307692308,
0.123076923076923,0.138461538461538,0.153846153846154,0.169230769230769,
0.184615384615385,0.2,0.215384615384615,0.230769230769231,0.246153846153846,
0.261538461538462,0.276923076923077,0.292307692307692,0.307692307692308,
0.323076923076923,0.338461538461538,0.353846153846154,0.369230769230769,
0.384615384615385,0.4,0.415384615384615,0.430769230769231,0.446153846153846,
0.461538461538462,0.476923076923077,0.492307692307692,0.507692307692308,
0.523076923076923,0.538461538461538,0.553846153846154,0.569230769230769,
0.584615384615384,0.6,0.615384615384615,0.63076923076923,0.646153846153846,
0.661538461538461,0.676923076923076,0.692307692307692,0.707692307692307,
0.723076923076922,0.738461538461538,0.753846153846153,0.769230769230768,
0.784615384615384,0.799999999999999,0.815384615384614,0.83076923076923,
0.846153846153845,0.86153846153846,0.876923076923076,0.892307692307691,
0.907692307692306,0.923076923076922,0.938461538461537,0.953846153846152,
0.969230769230768,0.984615384615383,1.),.UNSPECIFIED.)
CURVE()
GEOMETRIC_REPRESENTATION_ITEM()
RATIONAL_B_SPLINE_CURVE((1.,1.,1.,1.,1.,1.,1.,1.,1.,1.,1.,1.,1.,1.,1.,1.,
1.,1.,1.,1.,1.,1.,1.,1.,1.,1.,1.,1.,1.,1.,1.,1.,1.,1.,1.,1.,1.,1.,1.,1.,
1.,1.,1.,1.,1.,1.,1.,1.,1.,1.,1.,1.,1.,1.,1.,1.,1.,1.,1.,1.,1.,1.,1.,1.,
1.,1.,1.,1.,1.,1.))
REPRESENTATION_ITEM('')
);
#85=(
BOUNDED_CURVE()
B_SPLINE_CURVE(5,(#25334,#25335,#25336,#25337,#25338,#25339,#25340,#25341,
#25342,#25343,#25344,#25345,#25346,#25347,#25348,#25349,#25350,#25351,#25352,
#25353,#25354,#25355,#25356,#25357,#25358,#25359,#25360,#25361,#25362,#25363,
#25364,#25365,#25366,#25367,#25368,#25369,#25370,#25371,#25372,#25373,#25374,
#25375,#25376,#25377,#25378,#25379,#25380,#25381,#25382,#25383,#25384,#25385,
#25386,#25387,#25388,#25389,#25390,#25391,#25392,#25393,#25394,#25395,#25396,
#25397,#25398,#25399,#25400,#25401,#25402,#25403),.UNSPECIFIED.,.F.,.F.)
B_SPLINE_CURVE_WITH_KNOTS((6,1,1,1,1,1,1,1,1,1,1,1,1,1,1,1,1,1,1,1,1,1,
1,1,1,1,1,1,1,1,1,1,1,1,1,1,1,1,1,1,1,1,1,1,1,1,1,1,1,1,1,1,1,1,1,1,1,1,
1,1,1,1,1,1,1,6),(0.,0.0153846153846154,0.0307692307692308,0.0461538461538462,
0.0615384615384615,0.0769230769230769,0.0923076923076923,0.107692307692308,
0.123076923076923,0.138461538461538,0.153846153846154,0.169230769230769,
0.184615384615385,0.2,0.215384615384615,0.230769230769231,0.246153846153846,
0.261538461538462,0.276923076923077,0.292307692307692,0.307692307692308,
0.323076923076923,0.338461538461538,0.353846153846154,0.369230769230769,
0.384615384615385,0.4,0.415384615384615,0.430769230769231,0.446153846153846,
0.461538461538462,0.476923076923077,0.492307692307692,0.507692307692308,
0.523076923076923,0.538461538461538,0.553846153846154,0.569230769230769,
0.584615384615384,0.6,0.615384615384615,0.63076923076923,0.646153846153846,
0.661538461538461,0.676923076923076,0.692307692307692,0.707692307692307,
0.723076923076922,0.738461538461538,0.753846153846153,0.769230769230768,
0.784615384615384,0.799999999999999,0.815384615384614,0.83076923076923,
0.846153846153845,0.86153846153846,0.876923076923076,0.892307692307691,
0.907692307692306,0.923076923076922,0.938461538461537,0.953846153846152,
0.969230769230768,0.984615384615383,1.),.UNSPECIFIED.)
CURVE()
GEOMETRIC_REPRESENTATION_ITEM()
RATIONAL_B_SPLINE_CURVE((1.,1.,1.,1.,1.,1.,1.,1.,1.,1.,1.,1.,1.,1.,1.,1.,
1.,1.,1.,1.,1.,1.,1.,1.,1.,1.,1.,1.,1.,1.,1.,1.,1.,1.,1.,1.,1.,1.,1.,1.,
1.,1.,1.,1.,1.,1.,1.,1.,1.,1.,1.,1.,1.,1.,1.,1.,1.,1.,1.,1.,1.,1.,1.,1.,
1.,1.,1.,1.,1.,1.))
REPRESENTATION_ITEM('')
);
#86=(
BOUNDED_CURVE()
B_SPLINE_CURVE(5,(#25407,#25408,#25409,#25410,#25411,#25412,#25413,#25414,
#25415,#25416,#25417,#25418,#25419,#25420,#25421,#25422,#25423,#25424,#25425,
#25426,#25427,#25428,#25429,#25430,#25431,#25432,#25433,#25434,#25435,#25436,
#25437,#25438,#25439,#25440,#25441,#25442,#25443,#25444,#25445,#25446,#25447,
#25448,#25449,#25450,#25451,#25452,#25453,#25454,#25455,#25456,#25457,#25458,
#25459,#25460,#25461,#25462,#25463,#25464,#25465,#25466,#25467,#25468,#25469,
#25470,#25471,#25472,#25473,#25474,#25475,#25476),.UNSPECIFIED.,.F.,.F.)
B_SPLINE_CURVE_WITH_KNOTS((6,1,1,1,1,1,1,1,1,1,1,1,1,1,1,1,1,1,1,1,1,1,
1,1,1,1,1,1,1,1,1,1,1,1,1,1,1,1,1,1,1,1,1,1,1,1,1,1,1,1,1,1,1,1,1,1,1,1,
1,1,1,1,1,1,1,6),(0.,0.0153846153846154,0.0307692307692308,0.0461538461538462,
0.0615384615384615,0.0769230769230769,0.0923076923076923,0.107692307692308,
0.123076923076923,0.138461538461538,0.153846153846154,0.169230769230769,
0.184615384615385,0.2,0.215384615384615,0.230769230769231,0.246153846153846,
0.261538461538462,0.276923076923077,0.292307692307692,0.307692307692308,
0.323076923076923,0.338461538461538,0.353846153846154,0.369230769230769,
0.384615384615385,0.4,0.415384615384615,0.430769230769231,0.446153846153846,
0.461538461538462,0.476923076923077,0.492307692307692,0.507692307692308,
0.523076923076923,0.538461538461538,0.553846153846154,0.569230769230769,
0.584615384615384,0.6,0.615384615384615,0.63076923076923,0.646153846153846,
0.661538461538461,0.676923076923076,0.692307692307692,0.707692307692307,
0.723076923076922,0.738461538461538,0.753846153846153,0.769230769230768,
0.784615384615384,0.799999999999999,0.815384615384614,0.83076923076923,
0.846153846153845,0.86153846153846,0.876923076923076,0.892307692307691,
0.907692307692306,0.923076923076922,0.938461538461537,0.953846153846152,
0.969230769230768,0.984615384615383,1.),.UNSPECIFIED.)
CURVE()
GEOMETRIC_REPRESENTATION_ITEM()
RATIONAL_B_SPLINE_CURVE((1.,1.,1.,1.,1.,1.,1.,1.,1.,1.,1.,1.,1.,1.,1.,1.,
1.,1.,1.,1.,1.,1.,1.,1.,1.,1.,1.,1.,1.,1.,1.,1.,1.,1.,1.,1.,1.,1.,1.,1.,
1.,1.,1.,1.,1.,1.,1.,1.,1.,1.,1.,1.,1.,1.,1.,1.,1.,1.,1.,1.,1.,1.,1.,1.,
1.,1.,1.,1.,1.,1.))
REPRESENTATION_ITEM('')
);
#87=(
BOUNDED_CURVE()
B_SPLINE_CURVE(5,(#25480,#25481,#25482,#25483,#25484,#25485,#25486,#25487,
#25488,#25489,#25490,#25491,#25492,#25493,#25494,#25495,#25496,#25497,#25498,
#25499,#25500,#25501,#25502,#25503,#25504,#25505,#25506,#25507,#25508,#25509,
#25510,#25511,#25512,#25513,#25514,#25515,#25516,#25517,#25518,#25519,#25520,
#25521,#25522,#25523,#25524,#25525,#25526,#25527,#25528,#25529,#25530,#25531,
#25532,#25533,#25534,#25535,#25536,#25537,#25538,#25539,#25540,#25541,#25542,
#25543,#25544,#25545,#25546,#25547,#25548,#25549),.UNSPECIFIED.,.F.,.F.)
B_SPLINE_CURVE_WITH_KNOTS((6,1,1,1,1,1,1,1,1,1,1,1,1,1,1,1,1,1,1,1,1,1,
1,1,1,1,1,1,1,1,1,1,1,1,1,1,1,1,1,1,1,1,1,1,1,1,1,1,1,1,1,1,1,1,1,1,1,1,
1,1,1,1,1,1,1,6),(0.,0.0153846153846154,0.0307692307692308,0.0461538461538462,
0.0615384615384615,0.0769230769230769,0.0923076923076923,0.107692307692308,
0.123076923076923,0.138461538461538,0.153846153846154,0.169230769230769,
0.184615384615385,0.2,0.215384615384615,0.230769230769231,0.246153846153846,
0.261538461538462,0.276923076923077,0.292307692307692,0.307692307692308,
0.323076923076923,0.338461538461538,0.353846153846154,0.369230769230769,
0.384615384615385,0.4,0.415384615384615,0.430769230769231,0.446153846153846,
0.461538461538462,0.476923076923077,0.492307692307692,0.507692307692308,
0.523076923076923,0.538461538461538,0.553846153846154,0.569230769230769,
0.584615384615384,0.6,0.615384615384615,0.63076923076923,0.646153846153846,
0.661538461538461,0.676923076923076,0.692307692307692,0.707692307692307,
0.723076923076922,0.738461538461538,0.753846153846153,0.769230769230768,
0.784615384615384,0.799999999999999,0.815384615384614,0.83076923076923,
0.846153846153845,0.86153846153846,0.876923076923076,0.892307692307691,
0.907692307692306,0.923076923076922,0.938461538461537,0.953846153846152,
0.969230769230768,0.984615384615383,1.),.UNSPECIFIED.)
CURVE()
GEOMETRIC_REPRESENTATION_ITEM()
RATIONAL_B_SPLINE_CURVE((1.,1.,1.,1.,1.,1.,1.,1.,1.,1.,1.,1.,1.,1.,1.,1.,
1.,1.,1.,1.,1.,1.,1.,1.,1.,1.,1.,1.,1.,1.,1.,1.,1.,1.,1.,1.,1.,1.,1.,1.,
1.,1.,1.,1.,1.,1.,1.,1.,1.,1.,1.,1.,1.,1.,1.,1.,1.,1.,1.,1.,1.,1.,1.,1.,
1.,1.,1.,1.,1.,1.))
REPRESENTATION_ITEM('')
);
#88=(
BOUNDED_CURVE()
B_SPLINE_CURVE(5,(#25553,#25554,#25555,#25556,#25557,#25558,#25559,#25560,
#25561,#25562,#25563,#25564,#25565,#25566,#25567,#25568,#25569,#25570,#25571,
#25572,#25573,#25574,#25575,#25576,#25577,#25578,#25579,#25580,#25581,#25582,
#25583,#25584,#25585,#25586,#25587,#25588,#25589,#25590,#25591,#25592,#25593,
#25594,#25595,#25596,#25597,#25598,#25599,#25600,#25601,#25602,#25603,#25604,
#25605,#25606,#25607,#25608,#25609,#25610,#25611,#25612,#25613,#25614,#25615,
#25616,#25617,#25618,#25619,#25620,#25621,#25622),.UNSPECIFIED.,.F.,.F.)
B_SPLINE_CURVE_WITH_KNOTS((6,1,1,1,1,1,1,1,1,1,1,1,1,1,1,1,1,1,1,1,1,1,
1,1,1,1,1,1,1,1,1,1,1,1,1,1,1,1,1,1,1,1,1,1,1,1,1,1,1,1,1,1,1,1,1,1,1,1,
1,1,1,1,1,1,1,6),(0.,0.0153846153846154,0.0307692307692308,0.0461538461538462,
0.0615384615384615,0.0769230769230769,0.0923076923076923,0.107692307692308,
0.123076923076923,0.138461538461538,0.153846153846154,0.169230769230769,
0.184615384615385,0.2,0.215384615384615,0.230769230769231,0.246153846153846,
0.261538461538462,0.276923076923077,0.292307692307692,0.307692307692308,
0.323076923076923,0.338461538461538,0.353846153846154,0.369230769230769,
0.384615384615385,0.4,0.415384615384615,0.430769230769231,0.446153846153846,
0.461538461538462,0.476923076923077,0.492307692307692,0.507692307692308,
0.523076923076923,0.538461538461538,0.553846153846154,0.569230769230769,
0.584615384615384,0.6,0.615384615384615,0.63076923076923,0.646153846153846,
0.661538461538461,0.676923076923076,0.692307692307692,0.707692307692307,
0.723076923076922,0.738461538461538,0.753846153846153,0.769230769230768,
0.784615384615384,0.799999999999999,0.815384615384614,0.83076923076923,
0.846153846153845,0.86153846153846,0.876923076923076,0.892307692307691,
0.907692307692306,0.923076923076922,0.938461538461537,0.953846153846152,
0.969230769230768,0.984615384615383,1.),.UNSPECIFIED.)
CURVE()
GEOMETRIC_REPRESENTATION_ITEM()
RATIONAL_B_SPLINE_CURVE((1.,1.,1.,1.,1.,1.,1.,1.,1.,1.,1.,1.,1.,1.,1.,1.,
1.,1.,1.,1.,1.,1.,1.,1.,1.,1.,1.,1.,1.,1.,1.,1.,1.,1.,1.,1.,1.,1.,1.,1.,
1.,1.,1.,1.,1.,1.,1.,1.,1.,1.,1.,1.,1.,1.,1.,1.,1.,1.,1.,1.,1.,1.,1.,1.,
1.,1.,1.,1.,1.,1.))
REPRESENTATION_ITEM('')
);
#89=(
BOUNDED_CURVE()
B_SPLINE_CURVE(5,(#25626,#25627,#25628,#25629,#25630,#25631,#25632,#25633,
#25634,#25635,#25636,#25637,#25638,#25639,#25640,#25641,#25642,#25643,#25644,
#25645,#25646,#25647,#25648,#25649,#25650,#25651,#25652,#25653,#25654,#25655,
#25656,#25657,#25658,#25659,#25660,#25661,#25662,#25663,#25664,#25665,#25666,
#25667,#25668,#25669,#25670,#25671,#25672,#25673,#25674,#25675,#25676,#25677,
#25678,#25679,#25680,#25681,#25682,#25683,#25684,#25685,#25686,#25687,#25688,
#25689,#25690,#25691,#25692,#25693,#25694,#25695),.UNSPECIFIED.,.F.,.F.)
B_SPLINE_CURVE_WITH_KNOTS((6,1,1,1,1,1,1,1,1,1,1,1,1,1,1,1,1,1,1,1,1,1,
1,1,1,1,1,1,1,1,1,1,1,1,1,1,1,1,1,1,1,1,1,1,1,1,1,1,1,1,1,1,1,1,1,1,1,1,
1,1,1,1,1,1,1,6),(0.,0.0153846153846154,0.0307692307692308,0.0461538461538462,
0.0615384615384615,0.0769230769230769,0.0923076923076923,0.107692307692308,
0.123076923076923,0.138461538461538,0.153846153846154,0.169230769230769,
0.184615384615385,0.2,0.215384615384615,0.230769230769231,0.246153846153846,
0.261538461538462,0.276923076923077,0.292307692307692,0.307692307692308,
0.323076923076923,0.338461538461538,0.353846153846154,0.369230769230769,
0.384615384615385,0.4,0.415384615384615,0.430769230769231,0.446153846153846,
0.461538461538462,0.476923076923077,0.492307692307692,0.507692307692308,
0.523076923076923,0.538461538461538,0.553846153846154,0.569230769230769,
0.584615384615384,0.6,0.615384615384615,0.63076923076923,0.646153846153846,
0.661538461538461,0.676923076923076,0.692307692307692,0.707692307692307,
0.723076923076922,0.738461538461538,0.753846153846153,0.769230769230768,
0.784615384615384,0.799999999999999,0.815384615384614,0.83076923076923,
0.846153846153845,0.86153846153846,0.876923076923076,0.892307692307691,
0.907692307692306,0.923076923076922,0.938461538461537,0.953846153846152,
0.969230769230768,0.984615384615383,1.),.UNSPECIFIED.)
CURVE()
GEOMETRIC_REPRESENTATION_ITEM()
RATIONAL_B_SPLINE_CURVE((1.,1.,1.,1.,1.,1.,1.,1.,1.,1.,1.,1.,1.,1.,1.,1.,
1.,1.,1.,1.,1.,1.,1.,1.,1.,1.,1.,1.,1.,1.,1.,1.,1.,1.,1.,1.,1.,1.,1.,1.,
1.,1.,1.,1.,1.,1.,1.,1.,1.,1.,1.,1.,1.,1.,1.,1.,1.,1.,1.,1.,1.,1.,1.,1.,
1.,1.,1.,1.,1.,1.))
REPRESENTATION_ITEM('')
);
#90=(
BOUNDED_CURVE()
B_SPLINE_CURVE(5,(#25698,#25699,#25700,#25701,#25702,#25703,#25704,#25705,
#25706,#25707,#25708,#25709,#25710,#25711,#25712,#25713,#25714,#25715,#25716,
#25717,#25718,#25719,#25720,#25721,#25722,#25723,#25724,#25725,#25726,#25727,
#25728,#25729,#25730,#25731,#25732,#25733,#25734,#25735,#25736,#25737,#25738,
#25739,#25740,#25741,#25742,#25743,#25744,#25745,#25746,#25747,#25748,#25749,
#25750,#25751,#25752,#25753,#25754,#25755,#25756,#25757,#25758,#25759,#25760,
#25761,#25762,#25763,#25764,#25765,#25766,#25767),.UNSPECIFIED.,.F.,.F.)
B_SPLINE_CURVE_WITH_KNOTS((6,1,1,1,1,1,1,1,1,1,1,1,1,1,1,1,1,1,1,1,1,1,
1,1,1,1,1,1,1,1,1,1,1,1,1,1,1,1,1,1,1,1,1,1,1,1,1,1,1,1,1,1,1,1,1,1,1,1,
1,1,1,1,1,1,1,6),(0.,0.0153846153846154,0.0307692307692308,0.0461538461538462,
0.0615384615384615,0.0769230769230769,0.0923076923076923,0.107692307692308,
0.123076923076923,0.138461538461538,0.153846153846154,0.169230769230769,
0.184615384615385,0.2,0.215384615384615,0.230769230769231,0.246153846153846,
0.261538461538462,0.276923076923077,0.292307692307692,0.307692307692308,
0.323076923076923,0.338461538461538,0.353846153846154,0.369230769230769,
0.384615384615385,0.4,0.415384615384615,0.430769230769231,0.446153846153846,
0.461538461538462,0.476923076923077,0.492307692307692,0.507692307692308,
0.523076923076923,0.538461538461538,0.553846153846154,0.569230769230769,
0.584615384615384,0.6,0.615384615384615,0.63076923076923,0.646153846153846,
0.661538461538461,0.676923076923076,0.692307692307692,0.707692307692307,
0.723076923076922,0.738461538461538,0.753846153846153,0.769230769230768,
0.784615384615384,0.799999999999999,0.815384615384614,0.83076923076923,
0.846153846153845,0.86153846153846,0.876923076923076,0.892307692307691,
0.907692307692306,0.923076923076922,0.938461538461537,0.953846153846152,
0.969230769230768,0.984615384615383,1.),.UNSPECIFIED.)
CURVE()
GEOMETRIC_REPRESENTATION_ITEM()
RATIONAL_B_SPLINE_CURVE((1.,1.,1.,1.,1.,1.,1.,1.,1.,1.,1.,1.,1.,1.,1.,1.,
1.,1.,1.,1.,1.,1.,1.,1.,1.,1.,1.,1.,1.,1.,1.,1.,1.,1.,1.,1.,1.,1.,1.,1.,
1.,1.,1.,1.,1.,1.,1.,1.,1.,1.,1.,1.,1.,1.,1.,1.,1.,1.,1.,1.,1.,1.,1.,1.,
1.,1.,1.,1.,1.,1.))
REPRESENTATION_ITEM('')
);
#91=(
BOUNDED_CURVE()
B_SPLINE_CURVE(5,(#25921,#25922,#25923,#25924,#25925,#25926,#25927,#25928,
#25929,#25930,#25931,#25932,#25933,#25934,#25935,#25936,#25937,#25938,#25939,
#25940,#25941,#25942,#25943,#25944,#25945,#25946,#25947,#25948,#25949,#25950,
#25951,#25952,#25953,#25954,#25955,#25956,#25957,#25958,#25959,#25960,#25961,
#25962,#25963,#25964,#25965,#25966,#25967,#25968,#25969,#25970,#25971,#25972,
#25973,#25974,#25975,#25976,#25977,#25978,#25979,#25980,#25981,#25982,#25983,
#25984,#25985,#25986,#25987,#25988,#25989,#25990),.UNSPECIFIED.,.F.,.F.)
B_SPLINE_CURVE_WITH_KNOTS((6,1,1,1,1,1,1,1,1,1,1,1,1,1,1,1,1,1,1,1,1,1,
1,1,1,1,1,1,1,1,1,1,1,1,1,1,1,1,1,1,1,1,1,1,1,1,1,1,1,1,1,1,1,1,1,1,1,1,
1,1,1,1,1,1,1,6),(-1.,-0.984615384615383,-0.969230769230768,-0.953846153846152,
-0.938461538461537,-0.923076923076922,-0.907692307692306,-0.892307692307691,
-0.876923076923076,-0.86153846153846,-0.846153846153845,-0.83076923076923,
-0.815384615384614,-0.799999999999999,-0.784615384615384,-0.769230769230768,
-0.753846153846153,-0.738461538461538,-0.723076923076922,-0.707692307692307,
-0.692307692307692,-0.676923076923076,-0.661538461538461,-0.646153846153846,
-0.63076923076923,-0.615384615384615,-0.6,-0.584615384615384,-0.569230769230769,
-0.553846153846154,-0.538461538461538,-0.523076923076923,-0.507692307692308,
-0.492307692307692,-0.476923076923077,-0.461538461538462,-0.446153846153846,
-0.430769230769231,-0.415384615384615,-0.4,-0.384615384615385,-0.369230769230769,
-0.353846153846154,-0.338461538461538,-0.323076923076923,-0.307692307692308,
-0.292307692307692,-0.276923076923077,-0.261538461538462,-0.246153846153846,
-0.230769230769231,-0.215384615384615,-0.2,-0.184615384615385,-0.169230769230769,
-0.153846153846154,-0.138461538461538,-0.123076923076923,-0.107692307692308,
-0.0923076923076923,-0.0769230769230769,-0.0615384615384615,-0.0461538461538462,
-0.0307692307692308,-0.0153846153846154,0.),.UNSPECIFIED.)
CURVE()
GEOMETRIC_REPRESENTATION_ITEM()
RATIONAL_B_SPLINE_CURVE((1.,1.,1.,1.,1.,1.,1.,1.,1.,1.,1.,1.,1.,1.,1.,1.,
1.,1.,1.,1.,1.,1.,1.,1.,1.,1.,1.,1.,1.,1.,1.,1.,1.,1.,1.,1.,1.,1.,1.,1.,
1.,1.,1.,1.,1.,1.,1.,1.,1.,1.,1.,1.,1.,1.,1.,1.,1.,1.,1.,1.,1.,1.,1.,1.,
1.,1.,1.,1.,1.,1.))
REPRESENTATION_ITEM('')
);
#92=(
BOUNDED_CURVE()
B_SPLINE_CURVE(5,(#26137,#26138,#26139,#26140,#26141,#26142,#26143,#26144,
#26145,#26146,#26147,#26148,#26149,#26150,#26151,#26152,#26153,#26154,#26155,
#26156,#26157,#26158,#26159,#26160,#26161,#26162,#26163,#26164,#26165,#26166,
#26167,#26168,#26169,#26170,#26171,#26172,#26173,#26174,#26175,#26176,#26177,
#26178,#26179,#26180,#26181,#26182,#26183,#26184,#26185,#26186,#26187,#26188,
#26189,#26190,#26191,#26192,#26193,#26194,#26195,#26196,#26197,#26198,#26199,
#26200,#26201,#26202,#26203,#26204,#26205,#26206),.UNSPECIFIED.,.F.,.F.)
B_SPLINE_CURVE_WITH_KNOTS((6,1,1,1,1,1,1,1,1,1,1,1,1,1,1,1,1,1,1,1,1,1,
1,1,1,1,1,1,1,1,1,1,1,1,1,1,1,1,1,1,1,1,1,1,1,1,1,1,1,1,1,1,1,1,1,1,1,1,
1,1,1,1,1,1,1,6),(-1.,-0.984615384615383,-0.969230769230768,-0.953846153846152,
-0.938461538461537,-0.923076923076922,-0.907692307692306,-0.892307692307691,
-0.876923076923076,-0.86153846153846,-0.846153846153845,-0.83076923076923,
-0.815384615384614,-0.799999999999999,-0.784615384615384,-0.769230769230768,
-0.753846153846153,-0.738461538461538,-0.723076923076922,-0.707692307692307,
-0.692307692307692,-0.676923076923076,-0.661538461538461,-0.646153846153846,
-0.63076923076923,-0.615384615384615,-0.6,-0.584615384615384,-0.569230769230769,
-0.553846153846154,-0.538461538461538,-0.523076923076923,-0.507692307692308,
-0.492307692307692,-0.476923076923077,-0.461538461538462,-0.446153846153846,
-0.430769230769231,-0.415384615384615,-0.4,-0.384615384615385,-0.369230769230769,
-0.353846153846154,-0.338461538461538,-0.323076923076923,-0.307692307692308,
-0.292307692307692,-0.276923076923077,-0.261538461538462,-0.246153846153846,
-0.230769230769231,-0.215384615384615,-0.2,-0.184615384615385,-0.169230769230769,
-0.153846153846154,-0.138461538461538,-0.123076923076923,-0.107692307692308,
-0.0923076923076923,-0.0769230769230769,-0.0615384615384615,-0.0461538461538462,
-0.0307692307692308,-0.0153846153846154,0.),.UNSPECIFIED.)
CURVE()
GEOMETRIC_REPRESENTATION_ITEM()
RATIONAL_B_SPLINE_CURVE((1.,1.,1.,1.,1.,1.,1.,1.,1.,1.,1.,1.,1.,1.,1.,1.,
1.,1.,1.,1.,1.,1.,1.,1.,1.,1.,1.,1.,1.,1.,1.,1.,1.,1.,1.,1.,1.,1.,1.,1.,
1.,1.,1.,1.,1.,1.,1.,1.,1.,1.,1.,1.,1.,1.,1.,1.,1.,1.,1.,1.,1.,1.,1.,1.,
1.,1.,1.,1.,1.,1.))
REPRESENTATION_ITEM('')
);
#93=(
BOUNDED_CURVE()
B_SPLINE_CURVE(5,(#26353,#26354,#26355,#26356,#26357,#26358,#26359,#26360,
#26361,#26362,#26363,#26364,#26365,#26366,#26367,#26368,#26369,#26370,#26371,
#26372,#26373,#26374,#26375,#26376,#26377,#26378,#26379,#26380,#26381,#26382,
#26383,#26384,#26385,#26386,#26387,#26388,#26389,#26390,#26391,#26392,#26393,
#26394,#26395,#26396,#26397,#26398,#26399,#26400,#26401,#26402,#26403,#26404,
#26405,#26406,#26407,#26408,#26409,#26410,#26411,#26412,#26413,#26414,#26415,
#26416,#26417,#26418,#26419,#26420,#26421,#26422),.UNSPECIFIED.,.F.,.F.)
B_SPLINE_CURVE_WITH_KNOTS((6,1,1,1,1,1,1,1,1,1,1,1,1,1,1,1,1,1,1,1,1,1,
1,1,1,1,1,1,1,1,1,1,1,1,1,1,1,1,1,1,1,1,1,1,1,1,1,1,1,1,1,1,1,1,1,1,1,1,
1,1,1,1,1,1,1,6),(-1.,-0.984615384615383,-0.969230769230768,-0.953846153846152,
-0.938461538461537,-0.923076923076922,-0.907692307692306,-0.892307692307691,
-0.876923076923076,-0.86153846153846,-0.846153846153845,-0.83076923076923,
-0.815384615384614,-0.799999999999999,-0.784615384615384,-0.769230769230768,
-0.753846153846153,-0.738461538461538,-0.723076923076922,-0.707692307692307,
-0.692307692307692,-0.676923076923076,-0.661538461538461,-0.646153846153846,
-0.63076923076923,-0.615384615384615,-0.6,-0.584615384615384,-0.569230769230769,
-0.553846153846154,-0.538461538461538,-0.523076923076923,-0.507692307692308,
-0.492307692307692,-0.476923076923077,-0.461538461538462,-0.446153846153846,
-0.430769230769231,-0.415384615384615,-0.4,-0.384615384615385,-0.369230769230769,
-0.353846153846154,-0.338461538461538,-0.323076923076923,-0.307692307692308,
-0.292307692307692,-0.276923076923077,-0.261538461538462,-0.246153846153846,
-0.230769230769231,-0.215384615384615,-0.2,-0.184615384615385,-0.169230769230769,
-0.153846153846154,-0.138461538461538,-0.123076923076923,-0.107692307692308,
-0.0923076923076923,-0.0769230769230769,-0.0615384615384615,-0.0461538461538462,
-0.0307692307692308,-0.0153846153846154,0.),.UNSPECIFIED.)
CURVE()
GEOMETRIC_REPRESENTATION_ITEM()
RATIONAL_B_SPLINE_CURVE((1.,1.,1.,1.,1.,1.,1.,1.,1.,1.,1.,1.,1.,1.,1.,1.,
1.,1.,1.,1.,1.,1.,1.,1.,1.,1.,1.,1.,1.,1.,1.,1.,1.,1.,1.,1.,1.,1.,1.,1.,
1.,1.,1.,1.,1.,1.,1.,1.,1.,1.,1.,1.,1.,1.,1.,1.,1.,1.,1.,1.,1.,1.,1.,1.,
1.,1.,1.,1.,1.,1.))
REPRESENTATION_ITEM('')
);
#94=(
BOUNDED_CURVE()
B_SPLINE_CURVE(5,(#26569,#26570,#26571,#26572,#26573,#26574,#26575,#26576,
#26577,#26578,#26579,#26580,#26581,#26582,#26583,#26584,#26585,#26586,#26587,
#26588,#26589,#26590,#26591,#26592,#26593,#26594,#26595,#26596,#26597,#26598,
#26599,#26600,#26601,#26602,#26603,#26604,#26605,#26606,#26607,#26608,#26609,
#26610,#26611,#26612,#26613,#26614,#26615,#26616,#26617,#26618,#26619,#26620,
#26621,#26622,#26623,#26624,#26625,#26626,#26627,#26628,#26629,#26630,#26631,
#26632,#26633,#26634,#26635,#26636,#26637,#26638),.UNSPECIFIED.,.F.,.F.)
B_SPLINE_CURVE_WITH_KNOTS((6,1,1,1,1,1,1,1,1,1,1,1,1,1,1,1,1,1,1,1,1,1,
1,1,1,1,1,1,1,1,1,1,1,1,1,1,1,1,1,1,1,1,1,1,1,1,1,1,1,1,1,1,1,1,1,1,1,1,
1,1,1,1,1,1,1,6),(-1.,-0.984615384615383,-0.969230769230768,-0.953846153846152,
-0.938461538461537,-0.923076923076922,-0.907692307692306,-0.892307692307691,
-0.876923076923076,-0.86153846153846,-0.846153846153845,-0.83076923076923,
-0.815384615384614,-0.799999999999999,-0.784615384615384,-0.769230769230768,
-0.753846153846153,-0.738461538461538,-0.723076923076922,-0.707692307692307,
-0.692307692307692,-0.676923076923076,-0.661538461538461,-0.646153846153846,
-0.63076923076923,-0.615384615384615,-0.6,-0.584615384615384,-0.569230769230769,
-0.553846153846154,-0.538461538461538,-0.523076923076923,-0.507692307692308,
-0.492307692307692,-0.476923076923077,-0.461538461538462,-0.446153846153846,
-0.430769230769231,-0.415384615384615,-0.4,-0.384615384615385,-0.369230769230769,
-0.353846153846154,-0.338461538461538,-0.323076923076923,-0.307692307692308,
-0.292307692307692,-0.276923076923077,-0.261538461538462,-0.246153846153846,
-0.230769230769231,-0.215384615384615,-0.2,-0.184615384615385,-0.169230769230769,
-0.153846153846154,-0.138461538461538,-0.123076923076923,-0.107692307692308,
-0.0923076923076923,-0.0769230769230769,-0.0615384615384615,-0.0461538461538462,
-0.0307692307692308,-0.0153846153846154,0.),.UNSPECIFIED.)
CURVE()
GEOMETRIC_REPRESENTATION_ITEM()
RATIONAL_B_SPLINE_CURVE((1.,1.,1.,1.,1.,1.,1.,1.,1.,1.,1.,1.,1.,1.,1.,1.,
1.,1.,1.,1.,1.,1.,1.,1.,1.,1.,1.,1.,1.,1.,1.,1.,1.,1.,1.,1.,1.,1.,1.,1.,
1.,1.,1.,1.,1.,1.,1.,1.,1.,1.,1.,1.,1.,1.,1.,1.,1.,1.,1.,1.,1.,1.,1.,1.,
1.,1.,1.,1.,1.,1.))
REPRESENTATION_ITEM('')
);
#95=(
BOUNDED_CURVE()
B_SPLINE_CURVE(5,(#26785,#26786,#26787,#26788,#26789,#26790,#26791,#26792,
#26793,#26794,#26795,#26796,#26797,#26798,#26799,#26800,#26801,#26802,#26803,
#26804,#26805,#26806,#26807,#26808,#26809,#26810,#26811,#26812,#26813,#26814,
#26815,#26816,#26817,#26818,#26819,#26820,#26821,#26822,#26823,#26824,#26825,
#26826,#26827,#26828,#26829,#26830,#26831,#26832,#26833,#26834,#26835,#26836,
#26837,#26838,#26839,#26840,#26841,#26842,#26843,#26844,#26845,#26846,#26847,
#26848,#26849,#26850,#26851,#26852,#26853,#26854),.UNSPECIFIED.,.F.,.F.)
B_SPLINE_CURVE_WITH_KNOTS((6,1,1,1,1,1,1,1,1,1,1,1,1,1,1,1,1,1,1,1,1,1,
1,1,1,1,1,1,1,1,1,1,1,1,1,1,1,1,1,1,1,1,1,1,1,1,1,1,1,1,1,1,1,1,1,1,1,1,
1,1,1,1,1,1,1,6),(-1.,-0.984615384615383,-0.969230769230768,-0.953846153846152,
-0.938461538461537,-0.923076923076922,-0.907692307692306,-0.892307692307691,
-0.876923076923076,-0.86153846153846,-0.846153846153845,-0.83076923076923,
-0.815384615384614,-0.799999999999999,-0.784615384615384,-0.769230769230768,
-0.753846153846153,-0.738461538461538,-0.723076923076922,-0.707692307692307,
-0.692307692307692,-0.676923076923076,-0.661538461538461,-0.646153846153846,
-0.63076923076923,-0.615384615384615,-0.6,-0.584615384615384,-0.569230769230769,
-0.553846153846154,-0.538461538461538,-0.523076923076923,-0.507692307692308,
-0.492307692307692,-0.476923076923077,-0.461538461538462,-0.446153846153846,
-0.430769230769231,-0.415384615384615,-0.4,-0.384615384615385,-0.369230769230769,
-0.353846153846154,-0.338461538461538,-0.323076923076923,-0.307692307692308,
-0.292307692307692,-0.276923076923077,-0.261538461538462,-0.246153846153846,
-0.230769230769231,-0.215384615384615,-0.2,-0.184615384615385,-0.169230769230769,
-0.153846153846154,-0.138461538461538,-0.123076923076923,-0.107692307692308,
-0.0923076923076923,-0.0769230769230769,-0.0615384615384615,-0.0461538461538462,
-0.0307692307692308,-0.0153846153846154,0.),.UNSPECIFIED.)
CURVE()
GEOMETRIC_REPRESENTATION_ITEM()
RATIONAL_B_SPLINE_CURVE((1.,1.,1.,1.,1.,1.,1.,1.,1.,1.,1.,1.,1.,1.,1.,1.,
1.,1.,1.,1.,1.,1.,1.,1.,1.,1.,1.,1.,1.,1.,1.,1.,1.,1.,1.,1.,1.,1.,1.,1.,
1.,1.,1.,1.,1.,1.,1.,1.,1.,1.,1.,1.,1.,1.,1.,1.,1.,1.,1.,1.,1.,1.,1.,1.,
1.,1.,1.,1.,1.,1.))
REPRESENTATION_ITEM('')
);
#96=(
BOUNDED_CURVE()
B_SPLINE_CURVE(5,(#27001,#27002,#27003,#27004,#27005,#27006,#27007,#27008,
#27009,#27010,#27011,#27012,#27013,#27014,#27015,#27016,#27017,#27018,#27019,
#27020,#27021,#27022,#27023,#27024,#27025,#27026,#27027,#27028,#27029,#27030,
#27031,#27032,#27033,#27034,#27035,#27036,#27037,#27038,#27039,#27040,#27041,
#27042,#27043,#27044,#27045,#27046,#27047,#27048,#27049,#27050,#27051,#27052,
#27053,#27054,#27055,#27056,#27057,#27058,#27059,#27060,#27061,#27062,#27063,
#27064,#27065,#27066,#27067,#27068,#27069,#27070),.UNSPECIFIED.,.F.,.F.)
B_SPLINE_CURVE_WITH_KNOTS((6,1,1,1,1,1,1,1,1,1,1,1,1,1,1,1,1,1,1,1,1,1,
1,1,1,1,1,1,1,1,1,1,1,1,1,1,1,1,1,1,1,1,1,1,1,1,1,1,1,1,1,1,1,1,1,1,1,1,
1,1,1,1,1,1,1,6),(-1.,-0.984615384615383,-0.969230769230768,-0.953846153846152,
-0.938461538461537,-0.923076923076922,-0.907692307692306,-0.892307692307691,
-0.876923076923076,-0.86153846153846,-0.846153846153845,-0.83076923076923,
-0.815384615384614,-0.799999999999999,-0.784615384615384,-0.769230769230768,
-0.753846153846153,-0.738461538461538,-0.723076923076922,-0.707692307692307,
-0.692307692307692,-0.676923076923076,-0.661538461538461,-0.646153846153846,
-0.63076923076923,-0.615384615384615,-0.6,-0.584615384615384,-0.569230769230769,
-0.553846153846154,-0.538461538461538,-0.523076923076923,-0.507692307692308,
-0.492307692307692,-0.476923076923077,-0.461538461538462,-0.446153846153846,
-0.430769230769231,-0.415384615384615,-0.4,-0.384615384615385,-0.369230769230769,
-0.353846153846154,-0.338461538461538,-0.323076923076923,-0.307692307692308,
-0.292307692307692,-0.276923076923077,-0.261538461538462,-0.246153846153846,
-0.230769230769231,-0.215384615384615,-0.2,-0.184615384615385,-0.169230769230769,
-0.153846153846154,-0.138461538461538,-0.123076923076923,-0.107692307692308,
-0.0923076923076923,-0.0769230769230769,-0.0615384615384615,-0.0461538461538462,
-0.0307692307692308,-0.0153846153846154,0.),.UNSPECIFIED.)
CURVE()
GEOMETRIC_REPRESENTATION_ITEM()
RATIONAL_B_SPLINE_CURVE((1.,1.,1.,1.,1.,1.,1.,1.,1.,1.,1.,1.,1.,1.,1.,1.,
1.,1.,1.,1.,1.,1.,1.,1.,1.,1.,1.,1.,1.,1.,1.,1.,1.,1.,1.,1.,1.,1.,1.,1.,
1.,1.,1.,1.,1.,1.,1.,1.,1.,1.,1.,1.,1.,1.,1.,1.,1.,1.,1.,1.,1.,1.,1.,1.,
1.,1.,1.,1.,1.,1.))
REPRESENTATION_ITEM('')
);
#97=(
BOUNDED_CURVE()
B_SPLINE_CURVE(5,(#27217,#27218,#27219,#27220,#27221,#27222,#27223,#27224,
#27225,#27226,#27227,#27228,#27229,#27230,#27231,#27232,#27233,#27234,#27235,
#27236,#27237,#27238,#27239,#27240,#27241,#27242,#27243,#27244,#27245,#27246,
#27247,#27248,#27249,#27250,#27251,#27252,#27253,#27254,#27255,#27256,#27257,
#27258,#27259,#27260,#27261,#27262,#27263,#27264,#27265,#27266,#27267,#27268,
#27269,#27270,#27271,#27272,#27273,#27274,#27275,#27276,#27277,#27278,#27279,
#27280,#27281,#27282,#27283,#27284,#27285,#27286),.UNSPECIFIED.,.F.,.F.)
B_SPLINE_CURVE_WITH_KNOTS((6,1,1,1,1,1,1,1,1,1,1,1,1,1,1,1,1,1,1,1,1,1,
1,1,1,1,1,1,1,1,1,1,1,1,1,1,1,1,1,1,1,1,1,1,1,1,1,1,1,1,1,1,1,1,1,1,1,1,
1,1,1,1,1,1,1,6),(-1.,-0.984615384615383,-0.969230769230768,-0.953846153846152,
-0.938461538461537,-0.923076923076922,-0.907692307692306,-0.892307692307691,
-0.876923076923076,-0.86153846153846,-0.846153846153845,-0.83076923076923,
-0.815384615384614,-0.799999999999999,-0.784615384615384,-0.769230769230768,
-0.753846153846153,-0.738461538461538,-0.723076923076922,-0.707692307692307,
-0.692307692307692,-0.676923076923076,-0.661538461538461,-0.646153846153846,
-0.63076923076923,-0.615384615384615,-0.6,-0.584615384615384,-0.569230769230769,
-0.553846153846154,-0.538461538461538,-0.523076923076923,-0.507692307692308,
-0.492307692307692,-0.476923076923077,-0.461538461538462,-0.446153846153846,
-0.430769230769231,-0.415384615384615,-0.4,-0.384615384615385,-0.369230769230769,
-0.353846153846154,-0.338461538461538,-0.323076923076923,-0.307692307692308,
-0.292307692307692,-0.276923076923077,-0.261538461538462,-0.246153846153846,
-0.230769230769231,-0.215384615384615,-0.2,-0.184615384615385,-0.169230769230769,
-0.153846153846154,-0.138461538461538,-0.123076923076923,-0.107692307692308,
-0.0923076923076923,-0.0769230769230769,-0.0615384615384615,-0.0461538461538462,
-0.0307692307692308,-0.0153846153846154,0.),.UNSPECIFIED.)
CURVE()
GEOMETRIC_REPRESENTATION_ITEM()
RATIONAL_B_SPLINE_CURVE((1.,1.,1.,1.,1.,1.,1.,1.,1.,1.,1.,1.,1.,1.,1.,1.,
1.,1.,1.,1.,1.,1.,1.,1.,1.,1.,1.,1.,1.,1.,1.,1.,1.,1.,1.,1.,1.,1.,1.,1.,
1.,1.,1.,1.,1.,1.,1.,1.,1.,1.,1.,1.,1.,1.,1.,1.,1.,1.,1.,1.,1.,1.,1.,1.,
1.,1.,1.,1.,1.,1.))
REPRESENTATION_ITEM('')
);
#98=(
BOUNDED_CURVE()
B_SPLINE_CURVE(5,(#27433,#27434,#27435,#27436,#27437,#27438,#27439,#27440,
#27441,#27442,#27443,#27444,#27445,#27446,#27447,#27448,#27449,#27450,#27451,
#27452,#27453,#27454,#27455,#27456,#27457,#27458,#27459,#27460,#27461,#27462,
#27463,#27464,#27465,#27466,#27467,#27468,#27469,#27470,#27471,#27472,#27473,
#27474,#27475,#27476,#27477,#27478,#27479,#27480,#27481,#27482,#27483,#27484,
#27485,#27486,#27487,#27488,#27489,#27490,#27491,#27492,#27493,#27494,#27495,
#27496,#27497,#27498,#27499,#27500,#27501,#27502),.UNSPECIFIED.,.F.,.F.)
B_SPLINE_CURVE_WITH_KNOTS((6,1,1,1,1,1,1,1,1,1,1,1,1,1,1,1,1,1,1,1,1,1,
1,1,1,1,1,1,1,1,1,1,1,1,1,1,1,1,1,1,1,1,1,1,1,1,1,1,1,1,1,1,1,1,1,1,1,1,
1,1,1,1,1,1,1,6),(-1.,-0.984615384615383,-0.969230769230768,-0.953846153846152,
-0.938461538461537,-0.923076923076922,-0.907692307692306,-0.892307692307691,
-0.876923076923076,-0.86153846153846,-0.846153846153845,-0.83076923076923,
-0.815384615384614,-0.799999999999999,-0.784615384615384,-0.769230769230768,
-0.753846153846153,-0.738461538461538,-0.723076923076922,-0.707692307692307,
-0.692307692307692,-0.676923076923076,-0.661538461538461,-0.646153846153846,
-0.63076923076923,-0.615384615384615,-0.6,-0.584615384615384,-0.569230769230769,
-0.553846153846154,-0.538461538461538,-0.523076923076923,-0.507692307692308,
-0.492307692307692,-0.476923076923077,-0.461538461538462,-0.446153846153846,
-0.430769230769231,-0.415384615384615,-0.4,-0.384615384615385,-0.369230769230769,
-0.353846153846154,-0.338461538461538,-0.323076923076923,-0.307692307692308,
-0.292307692307692,-0.276923076923077,-0.261538461538462,-0.246153846153846,
-0.230769230769231,-0.215384615384615,-0.2,-0.184615384615385,-0.169230769230769,
-0.153846153846154,-0.138461538461538,-0.123076923076923,-0.107692307692308,
-0.0923076923076923,-0.0769230769230769,-0.0615384615384615,-0.0461538461538462,
-0.0307692307692308,-0.0153846153846154,0.),.UNSPECIFIED.)
CURVE()
GEOMETRIC_REPRESENTATION_ITEM()
RATIONAL_B_SPLINE_CURVE((1.,1.,1.,1.,1.,1.,1.,1.,1.,1.,1.,1.,1.,1.,1.,1.,
1.,1.,1.,1.,1.,1.,1.,1.,1.,1.,1.,1.,1.,1.,1.,1.,1.,1.,1.,1.,1.,1.,1.,1.,
1.,1.,1.,1.,1.,1.,1.,1.,1.,1.,1.,1.,1.,1.,1.,1.,1.,1.,1.,1.,1.,1.,1.,1.,
1.,1.,1.,1.,1.,1.))
REPRESENTATION_ITEM('')
);
#99=(
BOUNDED_CURVE()
B_SPLINE_CURVE(5,(#27649,#27650,#27651,#27652,#27653,#27654,#27655,#27656,
#27657,#27658,#27659,#27660,#27661,#27662,#27663,#27664,#27665,#27666,#27667,
#27668,#27669,#27670,#27671,#27672,#27673,#27674,#27675,#27676,#27677,#27678,
#27679,#27680,#27681,#27682,#27683,#27684,#27685,#27686,#27687,#27688,#27689,
#27690,#27691,#27692,#27693,#27694,#27695,#27696,#27697,#27698,#27699,#27700,
#27701,#27702,#27703,#27704,#27705,#27706,#27707,#27708,#27709,#27710,#27711,
#27712,#27713,#27714,#27715,#27716,#27717,#27718),.UNSPECIFIED.,.F.,.F.)
B_SPLINE_CURVE_WITH_KNOTS((6,1,1,1,1,1,1,1,1,1,1,1,1,1,1,1,1,1,1,1,1,1,
1,1,1,1,1,1,1,1,1,1,1,1,1,1,1,1,1,1,1,1,1,1,1,1,1,1,1,1,1,1,1,1,1,1,1,1,
1,1,1,1,1,1,1,6),(-1.,-0.984615384615383,-0.969230769230768,-0.953846153846152,
-0.938461538461537,-0.923076923076922,-0.907692307692306,-0.892307692307691,
-0.876923076923076,-0.86153846153846,-0.846153846153845,-0.83076923076923,
-0.815384615384614,-0.799999999999999,-0.784615384615384,-0.769230769230768,
-0.753846153846153,-0.738461538461538,-0.723076923076922,-0.707692307692307,
-0.692307692307692,-0.676923076923076,-0.661538461538461,-0.646153846153846,
-0.63076923076923,-0.615384615384615,-0.6,-0.584615384615384,-0.569230769230769,
-0.553846153846154,-0.538461538461538,-0.523076923076923,-0.507692307692308,
-0.492307692307692,-0.476923076923077,-0.461538461538462,-0.446153846153846,
-0.430769230769231,-0.415384615384615,-0.4,-0.384615384615385,-0.369230769230769,
-0.353846153846154,-0.338461538461538,-0.323076923076923,-0.307692307692308,
-0.292307692307692,-0.276923076923077,-0.261538461538462,-0.246153846153846,
-0.230769230769231,-0.215384615384615,-0.2,-0.184615384615385,-0.169230769230769,
-0.153846153846154,-0.138461538461538,-0.123076923076923,-0.107692307692308,
-0.0923076923076923,-0.0769230769230769,-0.0615384615384615,-0.0461538461538462,
-0.0307692307692308,-0.0153846153846154,0.),.UNSPECIFIED.)
CURVE()
GEOMETRIC_REPRESENTATION_ITEM()
RATIONAL_B_SPLINE_CURVE((1.,1.,1.,1.,1.,1.,1.,1.,1.,1.,1.,1.,1.,1.,1.,1.,
1.,1.,1.,1.,1.,1.,1.,1.,1.,1.,1.,1.,1.,1.,1.,1.,1.,1.,1.,1.,1.,1.,1.,1.,
1.,1.,1.,1.,1.,1.,1.,1.,1.,1.,1.,1.,1.,1.,1.,1.,1.,1.,1.,1.,1.,1.,1.,1.,
1.,1.,1.,1.,1.,1.))
REPRESENTATION_ITEM('')
);
#100=(
BOUNDED_CURVE()
B_SPLINE_CURVE(5,(#27865,#27866,#27867,#27868,#27869,#27870,#27871,#27872,
#27873,#27874,#27875,#27876,#27877,#27878,#27879,#27880,#27881,#27882,#27883,
#27884,#27885,#27886,#27887,#27888,#27889,#27890,#27891,#27892,#27893,#27894,
#27895,#27896,#27897,#27898,#27899,#27900,#27901,#27902,#27903,#27904,#27905,
#27906,#27907,#27908,#27909,#27910,#27911,#27912,#27913,#27914,#27915,#27916,
#27917,#27918,#27919,#27920,#27921,#27922,#27923,#27924,#27925,#27926,#27927,
#27928,#27929,#27930,#27931,#27932,#27933,#27934),.UNSPECIFIED.,.F.,.F.)
B_SPLINE_CURVE_WITH_KNOTS((6,1,1,1,1,1,1,1,1,1,1,1,1,1,1,1,1,1,1,1,1,1,
1,1,1,1,1,1,1,1,1,1,1,1,1,1,1,1,1,1,1,1,1,1,1,1,1,1,1,1,1,1,1,1,1,1,1,1,
1,1,1,1,1,1,1,6),(-1.,-0.984615384615383,-0.969230769230768,-0.953846153846152,
-0.938461538461537,-0.923076923076922,-0.907692307692306,-0.892307692307691,
-0.876923076923076,-0.86153846153846,-0.846153846153845,-0.83076923076923,
-0.815384615384614,-0.799999999999999,-0.784615384615384,-0.769230769230768,
-0.753846153846153,-0.738461538461538,-0.723076923076922,-0.707692307692307,
-0.692307692307692,-0.676923076923076,-0.661538461538461,-0.646153846153846,
-0.63076923076923,-0.615384615384615,-0.6,-0.584615384615384,-0.569230769230769,
-0.553846153846154,-0.538461538461538,-0.523076923076923,-0.507692307692308,
-0.492307692307692,-0.476923076923077,-0.461538461538462,-0.446153846153846,
-0.430769230769231,-0.415384615384615,-0.4,-0.384615384615385,-0.369230769230769,
-0.353846153846154,-0.338461538461538,-0.323076923076923,-0.307692307692308,
-0.292307692307692,-0.276923076923077,-0.261538461538462,-0.246153846153846,
-0.230769230769231,-0.215384615384615,-0.2,-0.184615384615385,-0.169230769230769,
-0.153846153846154,-0.138461538461538,-0.123076923076923,-0.107692307692308,
-0.0923076923076923,-0.0769230769230769,-0.0615384615384615,-0.0461538461538462,
-0.0307692307692308,-0.0153846153846154,0.),.UNSPECIFIED.)
CURVE()
GEOMETRIC_REPRESENTATION_ITEM()
RATIONAL_B_SPLINE_CURVE((1.,1.,1.,1.,1.,1.,1.,1.,1.,1.,1.,1.,1.,1.,1.,1.,
1.,1.,1.,1.,1.,1.,1.,1.,1.,1.,1.,1.,1.,1.,1.,1.,1.,1.,1.,1.,1.,1.,1.,1.,
1.,1.,1.,1.,1.,1.,1.,1.,1.,1.,1.,1.,1.,1.,1.,1.,1.,1.,1.,1.,1.,1.,1.,1.,
1.,1.,1.,1.,1.,1.))
REPRESENTATION_ITEM('')
);
#101=(
BOUNDED_CURVE()
B_SPLINE_CURVE(5,(#28081,#28082,#28083,#28084,#28085,#28086,#28087,#28088,
#28089,#28090,#28091,#28092,#28093,#28094,#28095,#28096,#28097,#28098,#28099,
#28100,#28101,#28102,#28103,#28104,#28105,#28106,#28107,#28108,#28109,#28110,
#28111,#28112,#28113,#28114,#28115,#28116,#28117,#28118,#28119,#28120,#28121,
#28122,#28123,#28124,#28125,#28126,#28127,#28128,#28129,#28130,#28131,#28132,
#28133,#28134,#28135,#28136,#28137,#28138,#28139,#28140,#28141,#28142,#28143,
#28144,#28145,#28146,#28147,#28148,#28149,#28150),.UNSPECIFIED.,.F.,.F.)
B_SPLINE_CURVE_WITH_KNOTS((6,1,1,1,1,1,1,1,1,1,1,1,1,1,1,1,1,1,1,1,1,1,
1,1,1,1,1,1,1,1,1,1,1,1,1,1,1,1,1,1,1,1,1,1,1,1,1,1,1,1,1,1,1,1,1,1,1,1,
1,1,1,1,1,1,1,6),(-1.,-0.984615384615383,-0.969230769230768,-0.953846153846152,
-0.938461538461537,-0.923076923076922,-0.907692307692306,-0.892307692307691,
-0.876923076923076,-0.86153846153846,-0.846153846153845,-0.83076923076923,
-0.815384615384614,-0.799999999999999,-0.784615384615384,-0.769230769230768,
-0.753846153846153,-0.738461538461538,-0.723076923076922,-0.707692307692307,
-0.692307692307692,-0.676923076923076,-0.661538461538461,-0.646153846153846,
-0.63076923076923,-0.615384615384615,-0.6,-0.584615384615384,-0.569230769230769,
-0.553846153846154,-0.538461538461538,-0.523076923076923,-0.507692307692308,
-0.492307692307692,-0.476923076923077,-0.461538461538462,-0.446153846153846,
-0.430769230769231,-0.415384615384615,-0.4,-0.384615384615385,-0.369230769230769,
-0.353846153846154,-0.338461538461538,-0.323076923076923,-0.307692307692308,
-0.292307692307692,-0.276923076923077,-0.261538461538462,-0.246153846153846,
-0.230769230769231,-0.215384615384615,-0.2,-0.184615384615385,-0.169230769230769,
-0.153846153846154,-0.138461538461538,-0.123076923076923,-0.107692307692308,
-0.0923076923076923,-0.0769230769230769,-0.0615384615384615,-0.0461538461538462,
-0.0307692307692308,-0.0153846153846154,0.),.UNSPECIFIED.)
CURVE()
GEOMETRIC_REPRESENTATION_ITEM()
RATIONAL_B_SPLINE_CURVE((1.,1.,1.,1.,1.,1.,1.,1.,1.,1.,1.,1.,1.,1.,1.,1.,
1.,1.,1.,1.,1.,1.,1.,1.,1.,1.,1.,1.,1.,1.,1.,1.,1.,1.,1.,1.,1.,1.,1.,1.,
1.,1.,1.,1.,1.,1.,1.,1.,1.,1.,1.,1.,1.,1.,1.,1.,1.,1.,1.,1.,1.,1.,1.,1.,
1.,1.,1.,1.,1.,1.))
REPRESENTATION_ITEM('')
);
#102=(
BOUNDED_CURVE()
B_SPLINE_CURVE(5,(#28297,#28298,#28299,#28300,#28301,#28302,#28303,#28304,
#28305,#28306,#28307,#28308,#28309,#28310,#28311,#28312,#28313,#28314,#28315,
#28316,#28317,#28318,#28319,#28320,#28321,#28322,#28323,#28324,#28325,#28326,
#28327,#28328,#28329,#28330,#28331,#28332,#28333,#28334,#28335,#28336,#28337,
#28338,#28339,#28340,#28341,#28342,#28343,#28344,#28345,#28346,#28347,#28348,
#28349,#28350,#28351,#28352,#28353,#28354,#28355,#28356,#28357,#28358,#28359,
#28360,#28361,#28362,#28363,#28364,#28365,#28366),.UNSPECIFIED.,.F.,.F.)
B_SPLINE_CURVE_WITH_KNOTS((6,1,1,1,1,1,1,1,1,1,1,1,1,1,1,1,1,1,1,1,1,1,
1,1,1,1,1,1,1,1,1,1,1,1,1,1,1,1,1,1,1,1,1,1,1,1,1,1,1,1,1,1,1,1,1,1,1,1,
1,1,1,1,1,1,1,6),(-1.,-0.984615384615383,-0.969230769230768,-0.953846153846152,
-0.938461538461537,-0.923076923076922,-0.907692307692306,-0.892307692307691,
-0.876923076923076,-0.86153846153846,-0.846153846153845,-0.83076923076923,
-0.815384615384614,-0.799999999999999,-0.784615384615384,-0.769230769230768,
-0.753846153846153,-0.738461538461538,-0.723076923076922,-0.707692307692307,
-0.692307692307692,-0.676923076923076,-0.661538461538461,-0.646153846153846,
-0.63076923076923,-0.615384615384615,-0.6,-0.584615384615384,-0.569230769230769,
-0.553846153846154,-0.538461538461538,-0.523076923076923,-0.507692307692308,
-0.492307692307692,-0.476923076923077,-0.461538461538462,-0.446153846153846,
-0.430769230769231,-0.415384615384615,-0.4,-0.384615384615385,-0.369230769230769,
-0.353846153846154,-0.338461538461538,-0.323076923076923,-0.307692307692308,
-0.292307692307692,-0.276923076923077,-0.261538461538462,-0.246153846153846,
-0.230769230769231,-0.215384615384615,-0.2,-0.184615384615385,-0.169230769230769,
-0.153846153846154,-0.138461538461538,-0.123076923076923,-0.107692307692308,
-0.0923076923076923,-0.0769230769230769,-0.0615384615384615,-0.0461538461538462,
-0.0307692307692308,-0.0153846153846154,0.),.UNSPECIFIED.)
CURVE()
GEOMETRIC_REPRESENTATION_ITEM()
RATIONAL_B_SPLINE_CURVE((1.,1.,1.,1.,1.,1.,1.,1.,1.,1.,1.,1.,1.,1.,1.,1.,
1.,1.,1.,1.,1.,1.,1.,1.,1.,1.,1.,1.,1.,1.,1.,1.,1.,1.,1.,1.,1.,1.,1.,1.,
1.,1.,1.,1.,1.,1.,1.,1.,1.,1.,1.,1.,1.,1.,1.,1.,1.,1.,1.,1.,1.,1.,1.,1.,
1.,1.,1.,1.,1.,1.))
REPRESENTATION_ITEM('')
);
#103=(
BOUNDED_CURVE()
B_SPLINE_CURVE(5,(#28513,#28514,#28515,#28516,#28517,#28518,#28519,#28520,
#28521,#28522,#28523,#28524,#28525,#28526,#28527,#28528,#28529,#28530,#28531,
#28532,#28533,#28534,#28535,#28536,#28537,#28538,#28539,#28540,#28541,#28542,
#28543,#28544,#28545,#28546,#28547,#28548,#28549,#28550,#28551,#28552,#28553,
#28554,#28555,#28556,#28557,#28558,#28559,#28560,#28561,#28562,#28563,#28564,
#28565,#28566,#28567,#28568,#28569,#28570,#28571,#28572,#28573,#28574,#28575,
#28576,#28577,#28578,#28579,#28580,#28581,#28582),.UNSPECIFIED.,.F.,.F.)
B_SPLINE_CURVE_WITH_KNOTS((6,1,1,1,1,1,1,1,1,1,1,1,1,1,1,1,1,1,1,1,1,1,
1,1,1,1,1,1,1,1,1,1,1,1,1,1,1,1,1,1,1,1,1,1,1,1,1,1,1,1,1,1,1,1,1,1,1,1,
1,1,1,1,1,1,1,6),(-1.,-0.984615384615383,-0.969230769230768,-0.953846153846152,
-0.938461538461537,-0.923076923076922,-0.907692307692306,-0.892307692307691,
-0.876923076923076,-0.86153846153846,-0.846153846153845,-0.83076923076923,
-0.815384615384614,-0.799999999999999,-0.784615384615384,-0.769230769230768,
-0.753846153846153,-0.738461538461538,-0.723076923076922,-0.707692307692307,
-0.692307692307692,-0.676923076923076,-0.661538461538461,-0.646153846153846,
-0.63076923076923,-0.615384615384615,-0.6,-0.584615384615384,-0.569230769230769,
-0.553846153846154,-0.538461538461538,-0.523076923076923,-0.507692307692308,
-0.492307692307692,-0.476923076923077,-0.461538461538462,-0.446153846153846,
-0.430769230769231,-0.415384615384615,-0.4,-0.384615384615385,-0.369230769230769,
-0.353846153846154,-0.338461538461538,-0.323076923076923,-0.307692307692308,
-0.292307692307692,-0.276923076923077,-0.261538461538462,-0.246153846153846,
-0.230769230769231,-0.215384615384615,-0.2,-0.184615384615385,-0.169230769230769,
-0.153846153846154,-0.138461538461538,-0.123076923076923,-0.107692307692308,
-0.0923076923076923,-0.0769230769230769,-0.0615384615384615,-0.0461538461538462,
-0.0307692307692308,-0.0153846153846154,0.),.UNSPECIFIED.)
CURVE()
GEOMETRIC_REPRESENTATION_ITEM()
RATIONAL_B_SPLINE_CURVE((1.,1.,1.,1.,1.,1.,1.,1.,1.,1.,1.,1.,1.,1.,1.,1.,
1.,1.,1.,1.,1.,1.,1.,1.,1.,1.,1.,1.,1.,1.,1.,1.,1.,1.,1.,1.,1.,1.,1.,1.,
1.,1.,1.,1.,1.,1.,1.,1.,1.,1.,1.,1.,1.,1.,1.,1.,1.,1.,1.,1.,1.,1.,1.,1.,
1.,1.,1.,1.,1.,1.))
REPRESENTATION_ITEM('')
);
#104=(
BOUNDED_CURVE()
B_SPLINE_CURVE(5,(#28729,#28730,#28731,#28732,#28733,#28734,#28735,#28736,
#28737,#28738,#28739,#28740,#28741,#28742,#28743,#28744,#28745,#28746,#28747,
#28748,#28749,#28750,#28751,#28752,#28753,#28754,#28755,#28756,#28757,#28758,
#28759,#28760,#28761,#28762,#28763,#28764,#28765,#28766,#28767,#28768,#28769,
#28770,#28771,#28772,#28773,#28774,#28775,#28776,#28777,#28778,#28779,#28780,
#28781,#28782,#28783,#28784,#28785,#28786,#28787,#28788,#28789,#28790,#28791,
#28792,#28793,#28794,#28795,#28796,#28797,#28798),.UNSPECIFIED.,.F.,.F.)
B_SPLINE_CURVE_WITH_KNOTS((6,1,1,1,1,1,1,1,1,1,1,1,1,1,1,1,1,1,1,1,1,1,
1,1,1,1,1,1,1,1,1,1,1,1,1,1,1,1,1,1,1,1,1,1,1,1,1,1,1,1,1,1,1,1,1,1,1,1,
1,1,1,1,1,1,1,6),(-1.,-0.984615384615383,-0.969230769230768,-0.953846153846152,
-0.938461538461537,-0.923076923076922,-0.907692307692306,-0.892307692307691,
-0.876923076923076,-0.86153846153846,-0.846153846153845,-0.83076923076923,
-0.815384615384614,-0.799999999999999,-0.784615384615384,-0.769230769230768,
-0.753846153846153,-0.738461538461538,-0.723076923076922,-0.707692307692307,
-0.692307692307692,-0.676923076923076,-0.661538461538461,-0.646153846153846,
-0.63076923076923,-0.615384615384615,-0.6,-0.584615384615384,-0.569230769230769,
-0.553846153846154,-0.538461538461538,-0.523076923076923,-0.507692307692308,
-0.492307692307692,-0.476923076923077,-0.461538461538462,-0.446153846153846,
-0.430769230769231,-0.415384615384615,-0.4,-0.384615384615385,-0.369230769230769,
-0.353846153846154,-0.338461538461538,-0.323076923076923,-0.307692307692308,
-0.292307692307692,-0.276923076923077,-0.261538461538462,-0.246153846153846,
-0.230769230769231,-0.215384615384615,-0.2,-0.184615384615385,-0.169230769230769,
-0.153846153846154,-0.138461538461538,-0.123076923076923,-0.107692307692308,
-0.0923076923076923,-0.0769230769230769,-0.0615384615384615,-0.0461538461538462,
-0.0307692307692308,-0.0153846153846154,0.),.UNSPECIFIED.)
CURVE()
GEOMETRIC_REPRESENTATION_ITEM()
RATIONAL_B_SPLINE_CURVE((1.,1.,1.,1.,1.,1.,1.,1.,1.,1.,1.,1.,1.,1.,1.,1.,
1.,1.,1.,1.,1.,1.,1.,1.,1.,1.,1.,1.,1.,1.,1.,1.,1.,1.,1.,1.,1.,1.,1.,1.,
1.,1.,1.,1.,1.,1.,1.,1.,1.,1.,1.,1.,1.,1.,1.,1.,1.,1.,1.,1.,1.,1.,1.,1.,
1.,1.,1.,1.,1.,1.))
REPRESENTATION_ITEM('')
);
#105=(
BOUNDED_CURVE()
B_SPLINE_CURVE(5,(#28945,#28946,#28947,#28948,#28949,#28950,#28951,#28952,
#28953,#28954,#28955,#28956,#28957,#28958,#28959,#28960,#28961,#28962,#28963,
#28964,#28965,#28966,#28967,#28968,#28969,#28970,#28971,#28972,#28973,#28974,
#28975,#28976,#28977,#28978,#28979,#28980,#28981,#28982,#28983,#28984,#28985,
#28986,#28987,#28988,#28989,#28990,#28991,#28992,#28993,#28994,#28995,#28996,
#28997,#28998,#28999,#29000,#29001,#29002,#29003,#29004,#29005,#29006,#29007,
#29008,#29009,#29010,#29011,#29012,#29013,#29014),.UNSPECIFIED.,.F.,.F.)
B_SPLINE_CURVE_WITH_KNOTS((6,1,1,1,1,1,1,1,1,1,1,1,1,1,1,1,1,1,1,1,1,1,
1,1,1,1,1,1,1,1,1,1,1,1,1,1,1,1,1,1,1,1,1,1,1,1,1,1,1,1,1,1,1,1,1,1,1,1,
1,1,1,1,1,1,1,6),(-1.,-0.984615384615383,-0.969230769230768,-0.953846153846152,
-0.938461538461537,-0.923076923076922,-0.907692307692306,-0.892307692307691,
-0.876923076923076,-0.86153846153846,-0.846153846153845,-0.83076923076923,
-0.815384615384614,-0.799999999999999,-0.784615384615384,-0.769230769230768,
-0.753846153846153,-0.738461538461538,-0.723076923076922,-0.707692307692307,
-0.692307692307692,-0.676923076923076,-0.661538461538461,-0.646153846153846,
-0.63076923076923,-0.615384615384615,-0.6,-0.584615384615384,-0.569230769230769,
-0.553846153846154,-0.538461538461538,-0.523076923076923,-0.507692307692308,
-0.492307692307692,-0.476923076923077,-0.461538461538462,-0.446153846153846,
-0.430769230769231,-0.415384615384615,-0.4,-0.384615384615385,-0.369230769230769,
-0.353846153846154,-0.338461538461538,-0.323076923076923,-0.307692307692308,
-0.292307692307692,-0.276923076923077,-0.261538461538462,-0.246153846153846,
-0.230769230769231,-0.215384615384615,-0.2,-0.184615384615385,-0.169230769230769,
-0.153846153846154,-0.138461538461538,-0.123076923076923,-0.107692307692308,
-0.0923076923076923,-0.0769230769230769,-0.0615384615384615,-0.0461538461538462,
-0.0307692307692308,-0.0153846153846154,0.),.UNSPECIFIED.)
CURVE()
GEOMETRIC_REPRESENTATION_ITEM()
RATIONAL_B_SPLINE_CURVE((1.,1.,1.,1.,1.,1.,1.,1.,1.,1.,1.,1.,1.,1.,1.,1.,
1.,1.,1.,1.,1.,1.,1.,1.,1.,1.,1.,1.,1.,1.,1.,1.,1.,1.,1.,1.,1.,1.,1.,1.,
1.,1.,1.,1.,1.,1.,1.,1.,1.,1.,1.,1.,1.,1.,1.,1.,1.,1.,1.,1.,1.,1.,1.,1.,
1.,1.,1.,1.,1.,1.))
REPRESENTATION_ITEM('')
);
#106=(
BOUNDED_CURVE()
B_SPLINE_CURVE(5,(#29161,#29162,#29163,#29164,#29165,#29166,#29167,#29168,
#29169,#29170,#29171,#29172,#29173,#29174,#29175,#29176,#29177,#29178,#29179,
#29180,#29181,#29182,#29183,#29184,#29185,#29186,#29187,#29188,#29189,#29190,
#29191,#29192,#29193,#29194,#29195,#29196,#29197,#29198,#29199,#29200,#29201,
#29202,#29203,#29204,#29205,#29206,#29207,#29208,#29209,#29210,#29211,#29212,
#29213,#29214,#29215,#29216,#29217,#29218,#29219,#29220,#29221,#29222,#29223,
#29224,#29225,#29226,#29227,#29228,#29229,#29230),.UNSPECIFIED.,.F.,.F.)
B_SPLINE_CURVE_WITH_KNOTS((6,1,1,1,1,1,1,1,1,1,1,1,1,1,1,1,1,1,1,1,1,1,
1,1,1,1,1,1,1,1,1,1,1,1,1,1,1,1,1,1,1,1,1,1,1,1,1,1,1,1,1,1,1,1,1,1,1,1,
1,1,1,1,1,1,1,6),(-1.,-0.984615384615383,-0.969230769230768,-0.953846153846152,
-0.938461538461537,-0.923076923076922,-0.907692307692306,-0.892307692307691,
-0.876923076923076,-0.86153846153846,-0.846153846153845,-0.83076923076923,
-0.815384615384614,-0.799999999999999,-0.784615384615384,-0.769230769230768,
-0.753846153846153,-0.738461538461538,-0.723076923076922,-0.707692307692307,
-0.692307692307692,-0.676923076923076,-0.661538461538461,-0.646153846153846,
-0.63076923076923,-0.615384615384615,-0.6,-0.584615384615384,-0.569230769230769,
-0.553846153846154,-0.538461538461538,-0.523076923076923,-0.507692307692308,
-0.492307692307692,-0.476923076923077,-0.461538461538462,-0.446153846153846,
-0.430769230769231,-0.415384615384615,-0.4,-0.384615384615385,-0.369230769230769,
-0.353846153846154,-0.338461538461538,-0.323076923076923,-0.307692307692308,
-0.292307692307692,-0.276923076923077,-0.261538461538462,-0.246153846153846,
-0.230769230769231,-0.215384615384615,-0.2,-0.184615384615385,-0.169230769230769,
-0.153846153846154,-0.138461538461538,-0.123076923076923,-0.107692307692308,
-0.0923076923076923,-0.0769230769230769,-0.0615384615384615,-0.0461538461538462,
-0.0307692307692308,-0.0153846153846154,0.),.UNSPECIFIED.)
CURVE()
GEOMETRIC_REPRESENTATION_ITEM()
RATIONAL_B_SPLINE_CURVE((1.,1.,1.,1.,1.,1.,1.,1.,1.,1.,1.,1.,1.,1.,1.,1.,
1.,1.,1.,1.,1.,1.,1.,1.,1.,1.,1.,1.,1.,1.,1.,1.,1.,1.,1.,1.,1.,1.,1.,1.,
1.,1.,1.,1.,1.,1.,1.,1.,1.,1.,1.,1.,1.,1.,1.,1.,1.,1.,1.,1.,1.,1.,1.,1.,
1.,1.,1.,1.,1.,1.))
REPRESENTATION_ITEM('')
);
#107=(
BOUNDED_CURVE()
B_SPLINE_CURVE(5,(#29377,#29378,#29379,#29380,#29381,#29382,#29383,#29384,
#29385,#29386,#29387,#29388,#29389,#29390,#29391,#29392,#29393,#29394,#29395,
#29396,#29397,#29398,#29399,#29400,#29401,#29402,#29403,#29404,#29405,#29406,
#29407,#29408,#29409,#29410,#29411,#29412,#29413,#29414,#29415,#29416,#29417,
#29418,#29419,#29420,#29421,#29422,#29423,#29424,#29425,#29426,#29427,#29428,
#29429,#29430,#29431,#29432,#29433,#29434,#29435,#29436,#29437,#29438,#29439,
#29440,#29441,#29442,#29443,#29444,#29445,#29446),.UNSPECIFIED.,.F.,.F.)
B_SPLINE_CURVE_WITH_KNOTS((6,1,1,1,1,1,1,1,1,1,1,1,1,1,1,1,1,1,1,1,1,1,
1,1,1,1,1,1,1,1,1,1,1,1,1,1,1,1,1,1,1,1,1,1,1,1,1,1,1,1,1,1,1,1,1,1,1,1,
1,1,1,1,1,1,1,6),(-1.,-0.984615384615383,-0.969230769230768,-0.953846153846152,
-0.938461538461537,-0.923076923076922,-0.907692307692306,-0.892307692307691,
-0.876923076923076,-0.86153846153846,-0.846153846153845,-0.83076923076923,
-0.815384615384614,-0.799999999999999,-0.784615384615384,-0.769230769230768,
-0.753846153846153,-0.738461538461538,-0.723076923076922,-0.707692307692307,
-0.692307692307692,-0.676923076923076,-0.661538461538461,-0.646153846153846,
-0.63076923076923,-0.615384615384615,-0.6,-0.584615384615384,-0.569230769230769,
-0.553846153846154,-0.538461538461538,-0.523076923076923,-0.507692307692308,
-0.492307692307692,-0.476923076923077,-0.461538461538462,-0.446153846153846,
-0.430769230769231,-0.415384615384615,-0.4,-0.384615384615385,-0.369230769230769,
-0.353846153846154,-0.338461538461538,-0.323076923076923,-0.307692307692308,
-0.292307692307692,-0.276923076923077,-0.261538461538462,-0.246153846153846,
-0.230769230769231,-0.215384615384615,-0.2,-0.184615384615385,-0.169230769230769,
-0.153846153846154,-0.138461538461538,-0.123076923076923,-0.107692307692308,
-0.0923076923076923,-0.0769230769230769,-0.0615384615384615,-0.0461538461538462,
-0.0307692307692308,-0.0153846153846154,0.),.UNSPECIFIED.)
CURVE()
GEOMETRIC_REPRESENTATION_ITEM()
RATIONAL_B_SPLINE_CURVE((1.,1.,1.,1.,1.,1.,1.,1.,1.,1.,1.,1.,1.,1.,1.,1.,
1.,1.,1.,1.,1.,1.,1.,1.,1.,1.,1.,1.,1.,1.,1.,1.,1.,1.,1.,1.,1.,1.,1.,1.,
1.,1.,1.,1.,1.,1.,1.,1.,1.,1.,1.,1.,1.,1.,1.,1.,1.,1.,1.,1.,1.,1.,1.,1.,
1.,1.,1.,1.,1.,1.))
REPRESENTATION_ITEM('')
);
#108=(
BOUNDED_CURVE()
B_SPLINE_CURVE(5,(#29593,#29594,#29595,#29596,#29597,#29598,#29599,#29600,
#29601,#29602,#29603,#29604,#29605,#29606,#29607,#29608,#29609,#29610,#29611,
#29612,#29613,#29614,#29615,#29616,#29617,#29618,#29619,#29620,#29621,#29622,
#29623,#29624,#29625,#29626,#29627,#29628,#29629,#29630,#29631,#29632,#29633,
#29634,#29635,#29636,#29637,#29638,#29639,#29640,#29641,#29642,#29643,#29644,
#29645,#29646,#29647,#29648,#29649,#29650,#29651,#29652,#29653,#29654,#29655,
#29656,#29657,#29658,#29659,#29660,#29661,#29662),.UNSPECIFIED.,.F.,.F.)
B_SPLINE_CURVE_WITH_KNOTS((6,1,1,1,1,1,1,1,1,1,1,1,1,1,1,1,1,1,1,1,1,1,
1,1,1,1,1,1,1,1,1,1,1,1,1,1,1,1,1,1,1,1,1,1,1,1,1,1,1,1,1,1,1,1,1,1,1,1,
1,1,1,1,1,1,1,6),(-1.,-0.984615384615383,-0.969230769230768,-0.953846153846152,
-0.938461538461537,-0.923076923076922,-0.907692307692306,-0.892307692307691,
-0.876923076923076,-0.86153846153846,-0.846153846153845,-0.83076923076923,
-0.815384615384614,-0.799999999999999,-0.784615384615384,-0.769230769230768,
-0.753846153846153,-0.738461538461538,-0.723076923076922,-0.707692307692307,
-0.692307692307692,-0.676923076923076,-0.661538461538461,-0.646153846153846,
-0.63076923076923,-0.615384615384615,-0.6,-0.584615384615384,-0.569230769230769,
-0.553846153846154,-0.538461538461538,-0.523076923076923,-0.507692307692308,
-0.492307692307692,-0.476923076923077,-0.461538461538462,-0.446153846153846,
-0.430769230769231,-0.415384615384615,-0.4,-0.384615384615385,-0.369230769230769,
-0.353846153846154,-0.338461538461538,-0.323076923076923,-0.307692307692308,
-0.292307692307692,-0.276923076923077,-0.261538461538462,-0.246153846153846,
-0.230769230769231,-0.215384615384615,-0.2,-0.184615384615385,-0.169230769230769,
-0.153846153846154,-0.138461538461538,-0.123076923076923,-0.107692307692308,
-0.0923076923076923,-0.0769230769230769,-0.0615384615384615,-0.0461538461538462,
-0.0307692307692308,-0.0153846153846154,0.),.UNSPECIFIED.)
CURVE()
GEOMETRIC_REPRESENTATION_ITEM()
RATIONAL_B_SPLINE_CURVE((1.,1.,1.,1.,1.,1.,1.,1.,1.,1.,1.,1.,1.,1.,1.,1.,
1.,1.,1.,1.,1.,1.,1.,1.,1.,1.,1.,1.,1.,1.,1.,1.,1.,1.,1.,1.,1.,1.,1.,1.,
1.,1.,1.,1.,1.,1.,1.,1.,1.,1.,1.,1.,1.,1.,1.,1.,1.,1.,1.,1.,1.,1.,1.,1.,
1.,1.,1.,1.,1.,1.))
REPRESENTATION_ITEM('')
);
#109=(
BOUNDED_CURVE()
B_SPLINE_CURVE(5,(#29809,#29810,#29811,#29812,#29813,#29814,#29815,#29816,
#29817,#29818,#29819,#29820,#29821,#29822,#29823,#29824,#29825,#29826,#29827,
#29828,#29829,#29830,#29831,#29832,#29833,#29834,#29835,#29836,#29837,#29838,
#29839,#29840,#29841,#29842,#29843,#29844,#29845,#29846,#29847,#29848,#29849,
#29850,#29851,#29852,#29853,#29854,#29855,#29856,#29857,#29858,#29859,#29860,
#29861,#29862,#29863,#29864,#29865,#29866,#29867,#29868,#29869,#29870,#29871,
#29872,#29873,#29874,#29875,#29876,#29877,#29878),.UNSPECIFIED.,.F.,.F.)
B_SPLINE_CURVE_WITH_KNOTS((6,1,1,1,1,1,1,1,1,1,1,1,1,1,1,1,1,1,1,1,1,1,
1,1,1,1,1,1,1,1,1,1,1,1,1,1,1,1,1,1,1,1,1,1,1,1,1,1,1,1,1,1,1,1,1,1,1,1,
1,1,1,1,1,1,1,6),(-1.,-0.984615384615383,-0.969230769230768,-0.953846153846152,
-0.938461538461537,-0.923076923076922,-0.907692307692306,-0.892307692307691,
-0.876923076923076,-0.86153846153846,-0.846153846153845,-0.83076923076923,
-0.815384615384614,-0.799999999999999,-0.784615384615384,-0.769230769230768,
-0.753846153846153,-0.738461538461538,-0.723076923076922,-0.707692307692307,
-0.692307692307692,-0.676923076923076,-0.661538461538461,-0.646153846153846,
-0.63076923076923,-0.615384615384615,-0.6,-0.584615384615384,-0.569230769230769,
-0.553846153846154,-0.538461538461538,-0.523076923076923,-0.507692307692308,
-0.492307692307692,-0.476923076923077,-0.461538461538462,-0.446153846153846,
-0.430769230769231,-0.415384615384615,-0.4,-0.384615384615385,-0.369230769230769,
-0.353846153846154,-0.338461538461538,-0.323076923076923,-0.307692307692308,
-0.292307692307692,-0.276923076923077,-0.261538461538462,-0.246153846153846,
-0.230769230769231,-0.215384615384615,-0.2,-0.184615384615385,-0.169230769230769,
-0.153846153846154,-0.138461538461538,-0.123076923076923,-0.107692307692308,
-0.0923076923076923,-0.0769230769230769,-0.0615384615384615,-0.0461538461538462,
-0.0307692307692308,-0.0153846153846154,0.),.UNSPECIFIED.)
CURVE()
GEOMETRIC_REPRESENTATION_ITEM()
RATIONAL_B_SPLINE_CURVE((1.,1.,1.,1.,1.,1.,1.,1.,1.,1.,1.,1.,1.,1.,1.,1.,
1.,1.,1.,1.,1.,1.,1.,1.,1.,1.,1.,1.,1.,1.,1.,1.,1.,1.,1.,1.,1.,1.,1.,1.,
1.,1.,1.,1.,1.,1.,1.,1.,1.,1.,1.,1.,1.,1.,1.,1.,1.,1.,1.,1.,1.,1.,1.,1.,
1.,1.,1.,1.,1.,1.))
REPRESENTATION_ITEM('')
);
#110=(
BOUNDED_CURVE()
B_SPLINE_CURVE(5,(#30025,#30026,#30027,#30028,#30029,#30030,#30031,#30032,
#30033,#30034,#30035,#30036,#30037,#30038,#30039,#30040,#30041,#30042,#30043,
#30044,#30045,#30046,#30047,#30048,#30049,#30050,#30051,#30052,#30053,#30054,
#30055,#30056,#30057,#30058,#30059,#30060,#30061,#30062,#30063,#30064,#30065,
#30066,#30067,#30068,#30069,#30070,#30071,#30072,#30073,#30074,#30075,#30076,
#30077,#30078,#30079,#30080,#30081,#30082,#30083,#30084,#30085,#30086,#30087,
#30088,#30089,#30090,#30091,#30092,#30093,#30094),.UNSPECIFIED.,.F.,.F.)
B_SPLINE_CURVE_WITH_KNOTS((6,1,1,1,1,1,1,1,1,1,1,1,1,1,1,1,1,1,1,1,1,1,
1,1,1,1,1,1,1,1,1,1,1,1,1,1,1,1,1,1,1,1,1,1,1,1,1,1,1,1,1,1,1,1,1,1,1,1,
1,1,1,1,1,1,1,6),(-1.,-0.984615384615383,-0.969230769230768,-0.953846153846152,
-0.938461538461537,-0.923076923076922,-0.907692307692306,-0.892307692307691,
-0.876923076923076,-0.86153846153846,-0.846153846153845,-0.83076923076923,
-0.815384615384614,-0.799999999999999,-0.784615384615384,-0.769230769230768,
-0.753846153846153,-0.738461538461538,-0.723076923076922,-0.707692307692307,
-0.692307692307692,-0.676923076923076,-0.661538461538461,-0.646153846153846,
-0.63076923076923,-0.615384615384615,-0.6,-0.584615384615384,-0.569230769230769,
-0.553846153846154,-0.538461538461538,-0.523076923076923,-0.507692307692308,
-0.492307692307692,-0.476923076923077,-0.461538461538462,-0.446153846153846,
-0.430769230769231,-0.415384615384615,-0.4,-0.384615384615385,-0.369230769230769,
-0.353846153846154,-0.338461538461538,-0.323076923076923,-0.307692307692308,
-0.292307692307692,-0.276923076923077,-0.261538461538462,-0.246153846153846,
-0.230769230769231,-0.215384615384615,-0.2,-0.184615384615385,-0.169230769230769,
-0.153846153846154,-0.138461538461538,-0.123076923076923,-0.107692307692308,
-0.0923076923076923,-0.0769230769230769,-0.0615384615384615,-0.0461538461538462,
-0.0307692307692308,-0.0153846153846154,0.),.UNSPECIFIED.)
CURVE()
GEOMETRIC_REPRESENTATION_ITEM()
RATIONAL_B_SPLINE_CURVE((1.,1.,1.,1.,1.,1.,1.,1.,1.,1.,1.,1.,1.,1.,1.,1.,
1.,1.,1.,1.,1.,1.,1.,1.,1.,1.,1.,1.,1.,1.,1.,1.,1.,1.,1.,1.,1.,1.,1.,1.,
1.,1.,1.,1.,1.,1.,1.,1.,1.,1.,1.,1.,1.,1.,1.,1.,1.,1.,1.,1.,1.,1.,1.,1.,
1.,1.,1.,1.,1.,1.))
REPRESENTATION_ITEM('')
);
#111=(
BOUNDED_CURVE()
B_SPLINE_CURVE(5,(#30241,#30242,#30243,#30244,#30245,#30246,#30247,#30248,
#30249,#30250,#30251,#30252,#30253,#30254,#30255,#30256,#30257,#30258,#30259,
#30260,#30261,#30262,#30263,#30264,#30265,#30266,#30267,#30268,#30269,#30270,
#30271,#30272,#30273,#30274,#30275,#30276,#30277,#30278,#30279,#30280,#30281,
#30282,#30283,#30284,#30285,#30286,#30287,#30288,#30289,#30290,#30291,#30292,
#30293,#30294,#30295,#30296,#30297,#30298,#30299,#30300,#30301,#30302,#30303,
#30304,#30305,#30306,#30307,#30308,#30309,#30310),.UNSPECIFIED.,.F.,.F.)
B_SPLINE_CURVE_WITH_KNOTS((6,1,1,1,1,1,1,1,1,1,1,1,1,1,1,1,1,1,1,1,1,1,
1,1,1,1,1,1,1,1,1,1,1,1,1,1,1,1,1,1,1,1,1,1,1,1,1,1,1,1,1,1,1,1,1,1,1,1,
1,1,1,1,1,1,1,6),(-1.,-0.984615384615383,-0.969230769230768,-0.953846153846152,
-0.938461538461537,-0.923076923076922,-0.907692307692306,-0.892307692307691,
-0.876923076923076,-0.86153846153846,-0.846153846153845,-0.83076923076923,
-0.815384615384614,-0.799999999999999,-0.784615384615384,-0.769230769230768,
-0.753846153846153,-0.738461538461538,-0.723076923076922,-0.707692307692307,
-0.692307692307692,-0.676923076923076,-0.661538461538461,-0.646153846153846,
-0.63076923076923,-0.615384615384615,-0.6,-0.584615384615384,-0.569230769230769,
-0.553846153846154,-0.538461538461538,-0.523076923076923,-0.507692307692308,
-0.492307692307692,-0.476923076923077,-0.461538461538462,-0.446153846153846,
-0.430769230769231,-0.415384615384615,-0.4,-0.384615384615385,-0.369230769230769,
-0.353846153846154,-0.338461538461538,-0.323076923076923,-0.307692307692308,
-0.292307692307692,-0.276923076923077,-0.261538461538462,-0.246153846153846,
-0.230769230769231,-0.215384615384615,-0.2,-0.184615384615385,-0.169230769230769,
-0.153846153846154,-0.138461538461538,-0.123076923076923,-0.107692307692308,
-0.0923076923076923,-0.0769230769230769,-0.0615384615384615,-0.0461538461538462,
-0.0307692307692308,-0.0153846153846154,0.),.UNSPECIFIED.)
CURVE()
GEOMETRIC_REPRESENTATION_ITEM()
RATIONAL_B_SPLINE_CURVE((1.,1.,1.,1.,1.,1.,1.,1.,1.,1.,1.,1.,1.,1.,1.,1.,
1.,1.,1.,1.,1.,1.,1.,1.,1.,1.,1.,1.,1.,1.,1.,1.,1.,1.,1.,1.,1.,1.,1.,1.,
1.,1.,1.,1.,1.,1.,1.,1.,1.,1.,1.,1.,1.,1.,1.,1.,1.,1.,1.,1.,1.,1.,1.,1.,
1.,1.,1.,1.,1.,1.))
REPRESENTATION_ITEM('')
);
#112=(
BOUNDED_CURVE()
B_SPLINE_CURVE(5,(#30457,#30458,#30459,#30460,#30461,#30462,#30463,#30464,
#30465,#30466,#30467,#30468,#30469,#30470,#30471,#30472,#30473,#30474,#30475,
#30476,#30477,#30478,#30479,#30480,#30481,#30482,#30483,#30484,#30485,#30486,
#30487,#30488,#30489,#30490,#30491,#30492,#30493,#30494,#30495,#30496,#30497,
#30498,#30499,#30500,#30501,#30502,#30503,#30504,#30505,#30506,#30507,#30508,
#30509,#30510,#30511,#30512,#30513,#30514,#30515,#30516,#30517,#30518,#30519,
#30520,#30521,#30522,#30523,#30524,#30525,#30526),.UNSPECIFIED.,.F.,.F.)
B_SPLINE_CURVE_WITH_KNOTS((6,1,1,1,1,1,1,1,1,1,1,1,1,1,1,1,1,1,1,1,1,1,
1,1,1,1,1,1,1,1,1,1,1,1,1,1,1,1,1,1,1,1,1,1,1,1,1,1,1,1,1,1,1,1,1,1,1,1,
1,1,1,1,1,1,1,6),(-1.,-0.984615384615383,-0.969230769230768,-0.953846153846152,
-0.938461538461537,-0.923076923076922,-0.907692307692306,-0.892307692307691,
-0.876923076923076,-0.86153846153846,-0.846153846153845,-0.83076923076923,
-0.815384615384614,-0.799999999999999,-0.784615384615384,-0.769230769230768,
-0.753846153846153,-0.738461538461538,-0.723076923076922,-0.707692307692307,
-0.692307692307692,-0.676923076923076,-0.661538461538461,-0.646153846153846,
-0.63076923076923,-0.615384615384615,-0.6,-0.584615384615384,-0.569230769230769,
-0.553846153846154,-0.538461538461538,-0.523076923076923,-0.507692307692308,
-0.492307692307692,-0.476923076923077,-0.461538461538462,-0.446153846153846,
-0.430769230769231,-0.415384615384615,-0.4,-0.384615384615385,-0.369230769230769,
-0.353846153846154,-0.338461538461538,-0.323076923076923,-0.307692307692308,
-0.292307692307692,-0.276923076923077,-0.261538461538462,-0.246153846153846,
-0.230769230769231,-0.215384615384615,-0.2,-0.184615384615385,-0.169230769230769,
-0.153846153846154,-0.138461538461538,-0.123076923076923,-0.107692307692308,
-0.0923076923076923,-0.0769230769230769,-0.0615384615384615,-0.0461538461538462,
-0.0307692307692308,-0.0153846153846154,0.),.UNSPECIFIED.)
CURVE()
GEOMETRIC_REPRESENTATION_ITEM()
RATIONAL_B_SPLINE_CURVE((1.,1.,1.,1.,1.,1.,1.,1.,1.,1.,1.,1.,1.,1.,1.,1.,
1.,1.,1.,1.,1.,1.,1.,1.,1.,1.,1.,1.,1.,1.,1.,1.,1.,1.,1.,1.,1.,1.,1.,1.,
1.,1.,1.,1.,1.,1.,1.,1.,1.,1.,1.,1.,1.,1.,1.,1.,1.,1.,1.,1.,1.,1.,1.,1.,
1.,1.,1.,1.,1.,1.))
REPRESENTATION_ITEM('')
);
#113=(
BOUNDED_CURVE()
B_SPLINE_CURVE(5,(#30673,#30674,#30675,#30676,#30677,#30678,#30679,#30680,
#30681,#30682,#30683,#30684,#30685,#30686,#30687,#30688,#30689,#30690,#30691,
#30692,#30693,#30694,#30695,#30696,#30697,#30698,#30699,#30700,#30701,#30702,
#30703,#30704,#30705,#30706,#30707,#30708,#30709,#30710,#30711,#30712,#30713,
#30714,#30715,#30716,#30717,#30718,#30719,#30720,#30721,#30722,#30723,#30724,
#30725,#30726,#30727,#30728,#30729,#30730,#30731,#30732,#30733,#30734,#30735,
#30736,#30737,#30738,#30739,#30740,#30741,#30742),.UNSPECIFIED.,.F.,.F.)
B_SPLINE_CURVE_WITH_KNOTS((6,1,1,1,1,1,1,1,1,1,1,1,1,1,1,1,1,1,1,1,1,1,
1,1,1,1,1,1,1,1,1,1,1,1,1,1,1,1,1,1,1,1,1,1,1,1,1,1,1,1,1,1,1,1,1,1,1,1,
1,1,1,1,1,1,1,6),(-1.,-0.984615384615383,-0.969230769230768,-0.953846153846152,
-0.938461538461537,-0.923076923076922,-0.907692307692306,-0.892307692307691,
-0.876923076923076,-0.86153846153846,-0.846153846153845,-0.83076923076923,
-0.815384615384614,-0.799999999999999,-0.784615384615384,-0.769230769230768,
-0.753846153846153,-0.738461538461538,-0.723076923076922,-0.707692307692307,
-0.692307692307692,-0.676923076923076,-0.661538461538461,-0.646153846153846,
-0.63076923076923,-0.615384615384615,-0.6,-0.584615384615384,-0.569230769230769,
-0.553846153846154,-0.538461538461538,-0.523076923076923,-0.507692307692308,
-0.492307692307692,-0.476923076923077,-0.461538461538462,-0.446153846153846,
-0.430769230769231,-0.415384615384615,-0.4,-0.384615384615385,-0.369230769230769,
-0.353846153846154,-0.338461538461538,-0.323076923076923,-0.307692307692308,
-0.292307692307692,-0.276923076923077,-0.261538461538462,-0.246153846153846,
-0.230769230769231,-0.215384615384615,-0.2,-0.184615384615385,-0.169230769230769,
-0.153846153846154,-0.138461538461538,-0.123076923076923,-0.107692307692308,
-0.0923076923076923,-0.0769230769230769,-0.0615384615384615,-0.0461538461538462,
-0.0307692307692308,-0.0153846153846154,0.),.UNSPECIFIED.)
CURVE()
GEOMETRIC_REPRESENTATION_ITEM()
RATIONAL_B_SPLINE_CURVE((1.,1.,1.,1.,1.,1.,1.,1.,1.,1.,1.,1.,1.,1.,1.,1.,
1.,1.,1.,1.,1.,1.,1.,1.,1.,1.,1.,1.,1.,1.,1.,1.,1.,1.,1.,1.,1.,1.,1.,1.,
1.,1.,1.,1.,1.,1.,1.,1.,1.,1.,1.,1.,1.,1.,1.,1.,1.,1.,1.,1.,1.,1.,1.,1.,
1.,1.,1.,1.,1.,1.))
REPRESENTATION_ITEM('')
);
#114=(
BOUNDED_CURVE()
B_SPLINE_CURVE(5,(#30889,#30890,#30891,#30892,#30893,#30894,#30895,#30896,
#30897,#30898,#30899,#30900,#30901,#30902,#30903,#30904,#30905,#30906,#30907,
#30908,#30909,#30910,#30911,#30912,#30913,#30914,#30915,#30916,#30917,#30918,
#30919,#30920,#30921,#30922,#30923,#30924,#30925,#30926,#30927,#30928,#30929,
#30930,#30931,#30932,#30933,#30934,#30935,#30936,#30937,#30938,#30939,#30940,
#30941,#30942,#30943,#30944,#30945,#30946,#30947,#30948,#30949,#30950,#30951,
#30952,#30953,#30954,#30955,#30956,#30957,#30958),.UNSPECIFIED.,.F.,.F.)
B_SPLINE_CURVE_WITH_KNOTS((6,1,1,1,1,1,1,1,1,1,1,1,1,1,1,1,1,1,1,1,1,1,
1,1,1,1,1,1,1,1,1,1,1,1,1,1,1,1,1,1,1,1,1,1,1,1,1,1,1,1,1,1,1,1,1,1,1,1,
1,1,1,1,1,1,1,6),(-1.,-0.984615384615383,-0.969230769230768,-0.953846153846152,
-0.938461538461537,-0.923076923076922,-0.907692307692306,-0.892307692307691,
-0.876923076923076,-0.86153846153846,-0.846153846153845,-0.83076923076923,
-0.815384615384614,-0.799999999999999,-0.784615384615384,-0.769230769230768,
-0.753846153846153,-0.738461538461538,-0.723076923076922,-0.707692307692307,
-0.692307692307692,-0.676923076923076,-0.661538461538461,-0.646153846153846,
-0.63076923076923,-0.615384615384615,-0.6,-0.584615384615384,-0.569230769230769,
-0.553846153846154,-0.538461538461538,-0.523076923076923,-0.507692307692308,
-0.492307692307692,-0.476923076923077,-0.461538461538462,-0.446153846153846,
-0.430769230769231,-0.415384615384615,-0.4,-0.384615384615385,-0.369230769230769,
-0.353846153846154,-0.338461538461538,-0.323076923076923,-0.307692307692308,
-0.292307692307692,-0.276923076923077,-0.261538461538462,-0.246153846153846,
-0.230769230769231,-0.215384615384615,-0.2,-0.184615384615385,-0.169230769230769,
-0.153846153846154,-0.138461538461538,-0.123076923076923,-0.107692307692308,
-0.0923076923076923,-0.0769230769230769,-0.0615384615384615,-0.0461538461538462,
-0.0307692307692308,-0.0153846153846154,0.),.UNSPECIFIED.)
CURVE()
GEOMETRIC_REPRESENTATION_ITEM()
RATIONAL_B_SPLINE_CURVE((1.,1.,1.,1.,1.,1.,1.,1.,1.,1.,1.,1.,1.,1.,1.,1.,
1.,1.,1.,1.,1.,1.,1.,1.,1.,1.,1.,1.,1.,1.,1.,1.,1.,1.,1.,1.,1.,1.,1.,1.,
1.,1.,1.,1.,1.,1.,1.,1.,1.,1.,1.,1.,1.,1.,1.,1.,1.,1.,1.,1.,1.,1.,1.,1.,
1.,1.,1.,1.,1.,1.))
REPRESENTATION_ITEM('')
);
#115=(
BOUNDED_CURVE()
B_SPLINE_CURVE(5,(#31105,#31106,#31107,#31108,#31109,#31110,#31111,#31112,
#31113,#31114,#31115,#31116,#31117,#31118,#31119,#31120,#31121,#31122,#31123,
#31124,#31125,#31126,#31127,#31128,#31129,#31130,#31131,#31132,#31133,#31134,
#31135,#31136,#31137,#31138,#31139,#31140,#31141,#31142,#31143,#31144,#31145,
#31146,#31147,#31148,#31149,#31150,#31151,#31152,#31153,#31154,#31155,#31156,
#31157,#31158,#31159,#31160,#31161,#31162,#31163,#31164,#31165,#31166,#31167,
#31168,#31169,#31170,#31171,#31172,#31173,#31174),.UNSPECIFIED.,.F.,.F.)
B_SPLINE_CURVE_WITH_KNOTS((6,1,1,1,1,1,1,1,1,1,1,1,1,1,1,1,1,1,1,1,1,1,
1,1,1,1,1,1,1,1,1,1,1,1,1,1,1,1,1,1,1,1,1,1,1,1,1,1,1,1,1,1,1,1,1,1,1,1,
1,1,1,1,1,1,1,6),(-1.,-0.984615384615383,-0.969230769230768,-0.953846153846152,
-0.938461538461537,-0.923076923076922,-0.907692307692306,-0.892307692307691,
-0.876923076923076,-0.86153846153846,-0.846153846153845,-0.83076923076923,
-0.815384615384614,-0.799999999999999,-0.784615384615384,-0.769230769230768,
-0.753846153846153,-0.738461538461538,-0.723076923076922,-0.707692307692307,
-0.692307692307692,-0.676923076923076,-0.661538461538461,-0.646153846153846,
-0.63076923076923,-0.615384615384615,-0.6,-0.584615384615384,-0.569230769230769,
-0.553846153846154,-0.538461538461538,-0.523076923076923,-0.507692307692308,
-0.492307692307692,-0.476923076923077,-0.461538461538462,-0.446153846153846,
-0.430769230769231,-0.415384615384615,-0.4,-0.384615384615385,-0.369230769230769,
-0.353846153846154,-0.338461538461538,-0.323076923076923,-0.307692307692308,
-0.292307692307692,-0.276923076923077,-0.261538461538462,-0.246153846153846,
-0.230769230769231,-0.215384615384615,-0.2,-0.184615384615385,-0.169230769230769,
-0.153846153846154,-0.138461538461538,-0.123076923076923,-0.107692307692308,
-0.0923076923076923,-0.0769230769230769,-0.0615384615384615,-0.0461538461538462,
-0.0307692307692308,-0.0153846153846154,0.),.UNSPECIFIED.)
CURVE()
GEOMETRIC_REPRESENTATION_ITEM()
RATIONAL_B_SPLINE_CURVE((1.,1.,1.,1.,1.,1.,1.,1.,1.,1.,1.,1.,1.,1.,1.,1.,
1.,1.,1.,1.,1.,1.,1.,1.,1.,1.,1.,1.,1.,1.,1.,1.,1.,1.,1.,1.,1.,1.,1.,1.,
1.,1.,1.,1.,1.,1.,1.,1.,1.,1.,1.,1.,1.,1.,1.,1.,1.,1.,1.,1.,1.,1.,1.,1.,
1.,1.,1.,1.,1.,1.))
REPRESENTATION_ITEM('')
);
#116=(
BOUNDED_CURVE()
B_SPLINE_CURVE(5,(#31321,#31322,#31323,#31324,#31325,#31326,#31327,#31328,
#31329,#31330,#31331,#31332,#31333,#31334,#31335,#31336,#31337,#31338,#31339,
#31340,#31341,#31342,#31343,#31344,#31345,#31346,#31347,#31348,#31349,#31350,
#31351,#31352,#31353,#31354,#31355,#31356,#31357,#31358,#31359,#31360,#31361,
#31362,#31363,#31364,#31365,#31366,#31367,#31368,#31369,#31370,#31371,#31372,
#31373,#31374,#31375,#31376,#31377,#31378,#31379,#31380,#31381,#31382,#31383,
#31384,#31385,#31386,#31387,#31388,#31389,#31390),.UNSPECIFIED.,.F.,.F.)
B_SPLINE_CURVE_WITH_KNOTS((6,1,1,1,1,1,1,1,1,1,1,1,1,1,1,1,1,1,1,1,1,1,
1,1,1,1,1,1,1,1,1,1,1,1,1,1,1,1,1,1,1,1,1,1,1,1,1,1,1,1,1,1,1,1,1,1,1,1,
1,1,1,1,1,1,1,6),(-1.,-0.984615384615383,-0.969230769230768,-0.953846153846152,
-0.938461538461537,-0.923076923076922,-0.907692307692306,-0.892307692307691,
-0.876923076923076,-0.86153846153846,-0.846153846153845,-0.83076923076923,
-0.815384615384614,-0.799999999999999,-0.784615384615384,-0.769230769230768,
-0.753846153846153,-0.738461538461538,-0.723076923076922,-0.707692307692307,
-0.692307692307692,-0.676923076923076,-0.661538461538461,-0.646153846153846,
-0.63076923076923,-0.615384615384615,-0.6,-0.584615384615384,-0.569230769230769,
-0.553846153846154,-0.538461538461538,-0.523076923076923,-0.507692307692308,
-0.492307692307692,-0.476923076923077,-0.461538461538462,-0.446153846153846,
-0.430769230769231,-0.415384615384615,-0.4,-0.384615384615385,-0.369230769230769,
-0.353846153846154,-0.338461538461538,-0.323076923076923,-0.307692307692308,
-0.292307692307692,-0.276923076923077,-0.261538461538462,-0.246153846153846,
-0.230769230769231,-0.215384615384615,-0.2,-0.184615384615385,-0.169230769230769,
-0.153846153846154,-0.138461538461538,-0.123076923076923,-0.107692307692308,
-0.0923076923076923,-0.0769230769230769,-0.0615384615384615,-0.0461538461538462,
-0.0307692307692308,-0.0153846153846154,0.),.UNSPECIFIED.)
CURVE()
GEOMETRIC_REPRESENTATION_ITEM()
RATIONAL_B_SPLINE_CURVE((1.,1.,1.,1.,1.,1.,1.,1.,1.,1.,1.,1.,1.,1.,1.,1.,
1.,1.,1.,1.,1.,1.,1.,1.,1.,1.,1.,1.,1.,1.,1.,1.,1.,1.,1.,1.,1.,1.,1.,1.,
1.,1.,1.,1.,1.,1.,1.,1.,1.,1.,1.,1.,1.,1.,1.,1.,1.,1.,1.,1.,1.,1.,1.,1.,
1.,1.,1.,1.,1.,1.))
REPRESENTATION_ITEM('')
);
#117=(
BOUNDED_CURVE()
B_SPLINE_CURVE(5,(#31537,#31538,#31539,#31540,#31541,#31542,#31543,#31544,
#31545,#31546,#31547,#31548,#31549,#31550,#31551,#31552,#31553,#31554,#31555,
#31556,#31557,#31558,#31559,#31560,#31561,#31562,#31563,#31564,#31565,#31566,
#31567,#31568,#31569,#31570,#31571,#31572,#31573,#31574,#31575,#31576,#31577,
#31578,#31579,#31580,#31581,#31582,#31583,#31584,#31585,#31586,#31587,#31588,
#31589,#31590,#31591,#31592,#31593,#31594,#31595,#31596,#31597,#31598,#31599,
#31600,#31601,#31602,#31603,#31604,#31605,#31606),.UNSPECIFIED.,.F.,.F.)
B_SPLINE_CURVE_WITH_KNOTS((6,1,1,1,1,1,1,1,1,1,1,1,1,1,1,1,1,1,1,1,1,1,
1,1,1,1,1,1,1,1,1,1,1,1,1,1,1,1,1,1,1,1,1,1,1,1,1,1,1,1,1,1,1,1,1,1,1,1,
1,1,1,1,1,1,1,6),(-1.,-0.984615384615383,-0.969230769230768,-0.953846153846152,
-0.938461538461537,-0.923076923076922,-0.907692307692306,-0.892307692307691,
-0.876923076923076,-0.86153846153846,-0.846153846153845,-0.83076923076923,
-0.815384615384614,-0.799999999999999,-0.784615384615384,-0.769230769230768,
-0.753846153846153,-0.738461538461538,-0.723076923076922,-0.707692307692307,
-0.692307692307692,-0.676923076923076,-0.661538461538461,-0.646153846153846,
-0.63076923076923,-0.615384615384615,-0.6,-0.584615384615384,-0.569230769230769,
-0.553846153846154,-0.538461538461538,-0.523076923076923,-0.507692307692308,
-0.492307692307692,-0.476923076923077,-0.461538461538462,-0.446153846153846,
-0.430769230769231,-0.415384615384615,-0.4,-0.384615384615385,-0.369230769230769,
-0.353846153846154,-0.338461538461538,-0.323076923076923,-0.307692307692308,
-0.292307692307692,-0.276923076923077,-0.261538461538462,-0.246153846153846,
-0.230769230769231,-0.215384615384615,-0.2,-0.184615384615385,-0.169230769230769,
-0.153846153846154,-0.138461538461538,-0.123076923076923,-0.107692307692308,
-0.0923076923076923,-0.0769230769230769,-0.0615384615384615,-0.0461538461538462,
-0.0307692307692308,-0.0153846153846154,0.),.UNSPECIFIED.)
CURVE()
GEOMETRIC_REPRESENTATION_ITEM()
RATIONAL_B_SPLINE_CURVE((1.,1.,1.,1.,1.,1.,1.,1.,1.,1.,1.,1.,1.,1.,1.,1.,
1.,1.,1.,1.,1.,1.,1.,1.,1.,1.,1.,1.,1.,1.,1.,1.,1.,1.,1.,1.,1.,1.,1.,1.,
1.,1.,1.,1.,1.,1.,1.,1.,1.,1.,1.,1.,1.,1.,1.,1.,1.,1.,1.,1.,1.,1.,1.,1.,
1.,1.,1.,1.,1.,1.))
REPRESENTATION_ITEM('')
);
#118=(
BOUNDED_CURVE()
B_SPLINE_CURVE(5,(#31753,#31754,#31755,#31756,#31757,#31758,#31759,#31760,
#31761,#31762,#31763,#31764,#31765,#31766,#31767,#31768,#31769,#31770,#31771,
#31772,#31773,#31774,#31775,#31776,#31777,#31778,#31779,#31780,#31781,#31782,
#31783,#31784,#31785,#31786,#31787,#31788,#31789,#31790,#31791,#31792,#31793,
#31794,#31795,#31796,#31797,#31798,#31799,#31800,#31801,#31802,#31803,#31804,
#31805,#31806,#31807,#31808,#31809,#31810,#31811,#31812,#31813,#31814,#31815,
#31816,#31817,#31818,#31819,#31820,#31821,#31822),.UNSPECIFIED.,.F.,.F.)
B_SPLINE_CURVE_WITH_KNOTS((6,1,1,1,1,1,1,1,1,1,1,1,1,1,1,1,1,1,1,1,1,1,
1,1,1,1,1,1,1,1,1,1,1,1,1,1,1,1,1,1,1,1,1,1,1,1,1,1,1,1,1,1,1,1,1,1,1,1,
1,1,1,1,1,1,1,6),(-1.,-0.984615384615383,-0.969230769230768,-0.953846153846152,
-0.938461538461537,-0.923076923076922,-0.907692307692306,-0.892307692307691,
-0.876923076923076,-0.86153846153846,-0.846153846153845,-0.83076923076923,
-0.815384615384614,-0.799999999999999,-0.784615384615384,-0.769230769230768,
-0.753846153846153,-0.738461538461538,-0.723076923076922,-0.707692307692307,
-0.692307692307692,-0.676923076923076,-0.661538461538461,-0.646153846153846,
-0.63076923076923,-0.615384615384615,-0.6,-0.584615384615384,-0.569230769230769,
-0.553846153846154,-0.538461538461538,-0.523076923076923,-0.507692307692308,
-0.492307692307692,-0.476923076923077,-0.461538461538462,-0.446153846153846,
-0.430769230769231,-0.415384615384615,-0.4,-0.384615384615385,-0.369230769230769,
-0.353846153846154,-0.338461538461538,-0.323076923076923,-0.307692307692308,
-0.292307692307692,-0.276923076923077,-0.261538461538462,-0.246153846153846,
-0.230769230769231,-0.215384615384615,-0.2,-0.184615384615385,-0.169230769230769,
-0.153846153846154,-0.138461538461538,-0.123076923076923,-0.107692307692308,
-0.0923076923076923,-0.0769230769230769,-0.0615384615384615,-0.0461538461538462,
-0.0307692307692308,-0.0153846153846154,0.),.UNSPECIFIED.)
CURVE()
GEOMETRIC_REPRESENTATION_ITEM()
RATIONAL_B_SPLINE_CURVE((1.,1.,1.,1.,1.,1.,1.,1.,1.,1.,1.,1.,1.,1.,1.,1.,
1.,1.,1.,1.,1.,1.,1.,1.,1.,1.,1.,1.,1.,1.,1.,1.,1.,1.,1.,1.,1.,1.,1.,1.,
1.,1.,1.,1.,1.,1.,1.,1.,1.,1.,1.,1.,1.,1.,1.,1.,1.,1.,1.,1.,1.,1.,1.,1.,
1.,1.,1.,1.,1.,1.))
REPRESENTATION_ITEM('')
);
#119=(
BOUNDED_CURVE()
B_SPLINE_CURVE(5,(#31969,#31970,#31971,#31972,#31973,#31974,#31975,#31976,
#31977,#31978,#31979,#31980,#31981,#31982,#31983,#31984,#31985,#31986,#31987,
#31988,#31989,#31990,#31991,#31992,#31993,#31994,#31995,#31996,#31997,#31998,
#31999,#32000,#32001,#32002,#32003,#32004,#32005,#32006,#32007,#32008,#32009,
#32010,#32011,#32012,#32013,#32014,#32015,#32016,#32017,#32018,#32019,#32020,
#32021,#32022,#32023,#32024,#32025,#32026,#32027,#32028,#32029,#32030,#32031,
#32032,#32033,#32034,#32035,#32036,#32037,#32038),.UNSPECIFIED.,.F.,.F.)
B_SPLINE_CURVE_WITH_KNOTS((6,1,1,1,1,1,1,1,1,1,1,1,1,1,1,1,1,1,1,1,1,1,
1,1,1,1,1,1,1,1,1,1,1,1,1,1,1,1,1,1,1,1,1,1,1,1,1,1,1,1,1,1,1,1,1,1,1,1,
1,1,1,1,1,1,1,6),(-1.,-0.984615384615383,-0.969230769230768,-0.953846153846152,
-0.938461538461537,-0.923076923076922,-0.907692307692306,-0.892307692307691,
-0.876923076923076,-0.86153846153846,-0.846153846153845,-0.83076923076923,
-0.815384615384614,-0.799999999999999,-0.784615384615384,-0.769230769230768,
-0.753846153846153,-0.738461538461538,-0.723076923076922,-0.707692307692307,
-0.692307692307692,-0.676923076923076,-0.661538461538461,-0.646153846153846,
-0.63076923076923,-0.615384615384615,-0.6,-0.584615384615384,-0.569230769230769,
-0.553846153846154,-0.538461538461538,-0.523076923076923,-0.507692307692308,
-0.492307692307692,-0.476923076923077,-0.461538461538462,-0.446153846153846,
-0.430769230769231,-0.415384615384615,-0.4,-0.384615384615385,-0.369230769230769,
-0.353846153846154,-0.338461538461538,-0.323076923076923,-0.307692307692308,
-0.292307692307692,-0.276923076923077,-0.261538461538462,-0.246153846153846,
-0.230769230769231,-0.215384615384615,-0.2,-0.184615384615385,-0.169230769230769,
-0.153846153846154,-0.138461538461538,-0.123076923076923,-0.107692307692308,
-0.0923076923076923,-0.0769230769230769,-0.0615384615384615,-0.0461538461538462,
-0.0307692307692308,-0.0153846153846154,0.),.UNSPECIFIED.)
CURVE()
GEOMETRIC_REPRESENTATION_ITEM()
RATIONAL_B_SPLINE_CURVE((1.,1.,1.,1.,1.,1.,1.,1.,1.,1.,1.,1.,1.,1.,1.,1.,
1.,1.,1.,1.,1.,1.,1.,1.,1.,1.,1.,1.,1.,1.,1.,1.,1.,1.,1.,1.,1.,1.,1.,1.,
1.,1.,1.,1.,1.,1.,1.,1.,1.,1.,1.,1.,1.,1.,1.,1.,1.,1.,1.,1.,1.,1.,1.,1.,
1.,1.,1.,1.,1.,1.))
REPRESENTATION_ITEM('')
);
#120=(
BOUNDED_CURVE()
B_SPLINE_CURVE(5,(#32185,#32186,#32187,#32188,#32189,#32190,#32191,#32192,
#32193,#32194,#32195,#32196,#32197,#32198,#32199,#32200,#32201,#32202,#32203,
#32204,#32205,#32206,#32207,#32208,#32209,#32210,#32211,#32212,#32213,#32214,
#32215,#32216,#32217,#32218,#32219,#32220,#32221,#32222,#32223,#32224,#32225,
#32226,#32227,#32228,#32229,#32230,#32231,#32232,#32233,#32234,#32235,#32236,
#32237,#32238,#32239,#32240,#32241,#32242,#32243,#32244,#32245,#32246,#32247,
#32248,#32249,#32250,#32251,#32252,#32253,#32254),.UNSPECIFIED.,.F.,.F.)
B_SPLINE_CURVE_WITH_KNOTS((6,1,1,1,1,1,1,1,1,1,1,1,1,1,1,1,1,1,1,1,1,1,
1,1,1,1,1,1,1,1,1,1,1,1,1,1,1,1,1,1,1,1,1,1,1,1,1,1,1,1,1,1,1,1,1,1,1,1,
1,1,1,1,1,1,1,6),(-1.,-0.984615384615383,-0.969230769230768,-0.953846153846152,
-0.938461538461537,-0.923076923076922,-0.907692307692306,-0.892307692307691,
-0.876923076923076,-0.86153846153846,-0.846153846153845,-0.83076923076923,
-0.815384615384614,-0.799999999999999,-0.784615384615384,-0.769230769230768,
-0.753846153846153,-0.738461538461538,-0.723076923076922,-0.707692307692307,
-0.692307692307692,-0.676923076923076,-0.661538461538461,-0.646153846153846,
-0.63076923076923,-0.615384615384615,-0.6,-0.584615384615384,-0.569230769230769,
-0.553846153846154,-0.538461538461538,-0.523076923076923,-0.507692307692308,
-0.492307692307692,-0.476923076923077,-0.461538461538462,-0.446153846153846,
-0.430769230769231,-0.415384615384615,-0.4,-0.384615384615385,-0.369230769230769,
-0.353846153846154,-0.338461538461538,-0.323076923076923,-0.307692307692308,
-0.292307692307692,-0.276923076923077,-0.261538461538462,-0.246153846153846,
-0.230769230769231,-0.215384615384615,-0.2,-0.184615384615385,-0.169230769230769,
-0.153846153846154,-0.138461538461538,-0.123076923076923,-0.107692307692308,
-0.0923076923076923,-0.0769230769230769,-0.0615384615384615,-0.0461538461538462,
-0.0307692307692308,-0.0153846153846154,0.),.UNSPECIFIED.)
CURVE()
GEOMETRIC_REPRESENTATION_ITEM()
RATIONAL_B_SPLINE_CURVE((1.,1.,1.,1.,1.,1.,1.,1.,1.,1.,1.,1.,1.,1.,1.,1.,
1.,1.,1.,1.,1.,1.,1.,1.,1.,1.,1.,1.,1.,1.,1.,1.,1.,1.,1.,1.,1.,1.,1.,1.,
1.,1.,1.,1.,1.,1.,1.,1.,1.,1.,1.,1.,1.,1.,1.,1.,1.,1.,1.,1.,1.,1.,1.,1.,
1.,1.,1.,1.,1.,1.))
REPRESENTATION_ITEM('')
);
#121=(
BOUNDED_CURVE()
B_SPLINE_CURVE(5,(#32401,#32402,#32403,#32404,#32405,#32406,#32407,#32408,
#32409,#32410,#32411,#32412,#32413,#32414,#32415,#32416,#32417,#32418,#32419,
#32420,#32421,#32422,#32423,#32424,#32425,#32426,#32427,#32428,#32429,#32430,
#32431,#32432,#32433,#32434,#32435,#32436,#32437,#32438,#32439,#32440,#32441,
#32442,#32443,#32444,#32445,#32446,#32447,#32448,#32449,#32450,#32451,#32452,
#32453,#32454,#32455,#32456,#32457,#32458,#32459,#32460,#32461,#32462,#32463,
#32464,#32465,#32466,#32467,#32468,#32469,#32470),.UNSPECIFIED.,.F.,.F.)
B_SPLINE_CURVE_WITH_KNOTS((6,1,1,1,1,1,1,1,1,1,1,1,1,1,1,1,1,1,1,1,1,1,
1,1,1,1,1,1,1,1,1,1,1,1,1,1,1,1,1,1,1,1,1,1,1,1,1,1,1,1,1,1,1,1,1,1,1,1,
1,1,1,1,1,1,1,6),(-1.,-0.984615384615383,-0.969230769230768,-0.953846153846152,
-0.938461538461537,-0.923076923076922,-0.907692307692306,-0.892307692307691,
-0.876923076923076,-0.86153846153846,-0.846153846153845,-0.83076923076923,
-0.815384615384614,-0.799999999999999,-0.784615384615384,-0.769230769230768,
-0.753846153846153,-0.738461538461538,-0.723076923076922,-0.707692307692307,
-0.692307692307692,-0.676923076923076,-0.661538461538461,-0.646153846153846,
-0.63076923076923,-0.615384615384615,-0.6,-0.584615384615384,-0.569230769230769,
-0.553846153846154,-0.538461538461538,-0.523076923076923,-0.507692307692308,
-0.492307692307692,-0.476923076923077,-0.461538461538462,-0.446153846153846,
-0.430769230769231,-0.415384615384615,-0.4,-0.384615384615385,-0.369230769230769,
-0.353846153846154,-0.338461538461538,-0.323076923076923,-0.307692307692308,
-0.292307692307692,-0.276923076923077,-0.261538461538462,-0.246153846153846,
-0.230769230769231,-0.215384615384615,-0.2,-0.184615384615385,-0.169230769230769,
-0.153846153846154,-0.138461538461538,-0.123076923076923,-0.107692307692308,
-0.0923076923076923,-0.0769230769230769,-0.0615384615384615,-0.0461538461538462,
-0.0307692307692308,-0.0153846153846154,0.),.UNSPECIFIED.)
CURVE()
GEOMETRIC_REPRESENTATION_ITEM()
RATIONAL_B_SPLINE_CURVE((1.,1.,1.,1.,1.,1.,1.,1.,1.,1.,1.,1.,1.,1.,1.,1.,
1.,1.,1.,1.,1.,1.,1.,1.,1.,1.,1.,1.,1.,1.,1.,1.,1.,1.,1.,1.,1.,1.,1.,1.,
1.,1.,1.,1.,1.,1.,1.,1.,1.,1.,1.,1.,1.,1.,1.,1.,1.,1.,1.,1.,1.,1.,1.,1.,
1.,1.,1.,1.,1.,1.))
REPRESENTATION_ITEM('')
);
#122=(
BOUNDED_CURVE()
B_SPLINE_CURVE(5,(#32617,#32618,#32619,#32620,#32621,#32622,#32623,#32624,
#32625,#32626,#32627,#32628,#32629,#32630,#32631,#32632,#32633,#32634,#32635,
#32636,#32637,#32638,#32639,#32640,#32641,#32642,#32643,#32644,#32645,#32646,
#32647,#32648,#32649,#32650,#32651,#32652,#32653,#32654,#32655,#32656,#32657,
#32658,#32659,#32660,#32661,#32662,#32663,#32664,#32665,#32666,#32667,#32668,
#32669,#32670,#32671,#32672,#32673,#32674,#32675,#32676,#32677,#32678,#32679,
#32680,#32681,#32682,#32683,#32684,#32685,#32686),.UNSPECIFIED.,.F.,.F.)
B_SPLINE_CURVE_WITH_KNOTS((6,1,1,1,1,1,1,1,1,1,1,1,1,1,1,1,1,1,1,1,1,1,
1,1,1,1,1,1,1,1,1,1,1,1,1,1,1,1,1,1,1,1,1,1,1,1,1,1,1,1,1,1,1,1,1,1,1,1,
1,1,1,1,1,1,1,6),(-1.,-0.984615384615383,-0.969230769230768,-0.953846153846152,
-0.938461538461537,-0.923076923076922,-0.907692307692306,-0.892307692307691,
-0.876923076923076,-0.86153846153846,-0.846153846153845,-0.83076923076923,
-0.815384615384614,-0.799999999999999,-0.784615384615384,-0.769230769230768,
-0.753846153846153,-0.738461538461538,-0.723076923076922,-0.707692307692307,
-0.692307692307692,-0.676923076923076,-0.661538461538461,-0.646153846153846,
-0.63076923076923,-0.615384615384615,-0.6,-0.584615384615384,-0.569230769230769,
-0.553846153846154,-0.538461538461538,-0.523076923076923,-0.507692307692308,
-0.492307692307692,-0.476923076923077,-0.461538461538462,-0.446153846153846,
-0.430769230769231,-0.415384615384615,-0.4,-0.384615384615385,-0.369230769230769,
-0.353846153846154,-0.338461538461538,-0.323076923076923,-0.307692307692308,
-0.292307692307692,-0.276923076923077,-0.261538461538462,-0.246153846153846,
-0.230769230769231,-0.215384615384615,-0.2,-0.184615384615385,-0.169230769230769,
-0.153846153846154,-0.138461538461538,-0.123076923076923,-0.107692307692308,
-0.0923076923076923,-0.0769230769230769,-0.0615384615384615,-0.0461538461538462,
-0.0307692307692308,-0.0153846153846154,0.),.UNSPECIFIED.)
CURVE()
GEOMETRIC_REPRESENTATION_ITEM()
RATIONAL_B_SPLINE_CURVE((1.,1.,1.,1.,1.,1.,1.,1.,1.,1.,1.,1.,1.,1.,1.,1.,
1.,1.,1.,1.,1.,1.,1.,1.,1.,1.,1.,1.,1.,1.,1.,1.,1.,1.,1.,1.,1.,1.,1.,1.,
1.,1.,1.,1.,1.,1.,1.,1.,1.,1.,1.,1.,1.,1.,1.,1.,1.,1.,1.,1.,1.,1.,1.,1.,
1.,1.,1.,1.,1.,1.))
REPRESENTATION_ITEM('')
);
#123=(
BOUNDED_CURVE()
B_SPLINE_CURVE(5,(#32833,#32834,#32835,#32836,#32837,#32838,#32839,#32840,
#32841,#32842,#32843,#32844,#32845,#32846,#32847,#32848,#32849,#32850,#32851,
#32852,#32853,#32854,#32855,#32856,#32857,#32858,#32859,#32860,#32861,#32862,
#32863,#32864,#32865,#32866,#32867,#32868,#32869,#32870,#32871,#32872,#32873,
#32874,#32875,#32876,#32877,#32878,#32879,#32880,#32881,#32882,#32883,#32884,
#32885,#32886,#32887,#32888,#32889,#32890,#32891,#32892,#32893,#32894,#32895,
#32896,#32897,#32898,#32899,#32900,#32901,#32902),.UNSPECIFIED.,.F.,.F.)
B_SPLINE_CURVE_WITH_KNOTS((6,1,1,1,1,1,1,1,1,1,1,1,1,1,1,1,1,1,1,1,1,1,
1,1,1,1,1,1,1,1,1,1,1,1,1,1,1,1,1,1,1,1,1,1,1,1,1,1,1,1,1,1,1,1,1,1,1,1,
1,1,1,1,1,1,1,6),(-1.,-0.984615384615383,-0.969230769230768,-0.953846153846152,
-0.938461538461537,-0.923076923076922,-0.907692307692306,-0.892307692307691,
-0.876923076923076,-0.86153846153846,-0.846153846153845,-0.83076923076923,
-0.815384615384614,-0.799999999999999,-0.784615384615384,-0.769230769230768,
-0.753846153846153,-0.738461538461538,-0.723076923076922,-0.707692307692307,
-0.692307692307692,-0.676923076923076,-0.661538461538461,-0.646153846153846,
-0.63076923076923,-0.615384615384615,-0.6,-0.584615384615384,-0.569230769230769,
-0.553846153846154,-0.538461538461538,-0.523076923076923,-0.507692307692308,
-0.492307692307692,-0.476923076923077,-0.461538461538462,-0.446153846153846,
-0.430769230769231,-0.415384615384615,-0.4,-0.384615384615385,-0.369230769230769,
-0.353846153846154,-0.338461538461538,-0.323076923076923,-0.307692307692308,
-0.292307692307692,-0.276923076923077,-0.261538461538462,-0.246153846153846,
-0.230769230769231,-0.215384615384615,-0.2,-0.184615384615385,-0.169230769230769,
-0.153846153846154,-0.138461538461538,-0.123076923076923,-0.107692307692308,
-0.0923076923076923,-0.0769230769230769,-0.0615384615384615,-0.0461538461538462,
-0.0307692307692308,-0.0153846153846154,0.),.UNSPECIFIED.)
CURVE()
GEOMETRIC_REPRESENTATION_ITEM()
RATIONAL_B_SPLINE_CURVE((1.,1.,1.,1.,1.,1.,1.,1.,1.,1.,1.,1.,1.,1.,1.,1.,
1.,1.,1.,1.,1.,1.,1.,1.,1.,1.,1.,1.,1.,1.,1.,1.,1.,1.,1.,1.,1.,1.,1.,1.,
1.,1.,1.,1.,1.,1.,1.,1.,1.,1.,1.,1.,1.,1.,1.,1.,1.,1.,1.,1.,1.,1.,1.,1.,
1.,1.,1.,1.,1.,1.))
REPRESENTATION_ITEM('')
);
#124=(
BOUNDED_CURVE()
B_SPLINE_CURVE(5,(#33049,#33050,#33051,#33052,#33053,#33054,#33055,#33056,
#33057,#33058,#33059,#33060,#33061,#33062,#33063,#33064,#33065,#33066,#33067,
#33068,#33069,#33070,#33071,#33072,#33073,#33074,#33075,#33076,#33077,#33078,
#33079,#33080,#33081,#33082,#33083,#33084,#33085,#33086,#33087,#33088,#33089,
#33090,#33091,#33092,#33093,#33094,#33095,#33096,#33097,#33098,#33099,#33100,
#33101,#33102,#33103,#33104,#33105,#33106,#33107,#33108,#33109,#33110,#33111,
#33112,#33113,#33114,#33115,#33116,#33117,#33118),.UNSPECIFIED.,.F.,.F.)
B_SPLINE_CURVE_WITH_KNOTS((6,1,1,1,1,1,1,1,1,1,1,1,1,1,1,1,1,1,1,1,1,1,
1,1,1,1,1,1,1,1,1,1,1,1,1,1,1,1,1,1,1,1,1,1,1,1,1,1,1,1,1,1,1,1,1,1,1,1,
1,1,1,1,1,1,1,6),(-1.,-0.984615384615383,-0.969230769230768,-0.953846153846152,
-0.938461538461537,-0.923076923076922,-0.907692307692306,-0.892307692307691,
-0.876923076923076,-0.86153846153846,-0.846153846153845,-0.83076923076923,
-0.815384615384614,-0.799999999999999,-0.784615384615384,-0.769230769230768,
-0.753846153846153,-0.738461538461538,-0.723076923076922,-0.707692307692307,
-0.692307692307692,-0.676923076923076,-0.661538461538461,-0.646153846153846,
-0.63076923076923,-0.615384615384615,-0.6,-0.584615384615384,-0.569230769230769,
-0.553846153846154,-0.538461538461538,-0.523076923076923,-0.507692307692308,
-0.492307692307692,-0.476923076923077,-0.461538461538462,-0.446153846153846,
-0.430769230769231,-0.415384615384615,-0.4,-0.384615384615385,-0.369230769230769,
-0.353846153846154,-0.338461538461538,-0.323076923076923,-0.307692307692308,
-0.292307692307692,-0.276923076923077,-0.261538461538462,-0.246153846153846,
-0.230769230769231,-0.215384615384615,-0.2,-0.184615384615385,-0.169230769230769,
-0.153846153846154,-0.138461538461538,-0.123076923076923,-0.107692307692308,
-0.0923076923076923,-0.0769230769230769,-0.0615384615384615,-0.0461538461538462,
-0.0307692307692308,-0.0153846153846154,0.),.UNSPECIFIED.)
CURVE()
GEOMETRIC_REPRESENTATION_ITEM()
RATIONAL_B_SPLINE_CURVE((1.,1.,1.,1.,1.,1.,1.,1.,1.,1.,1.,1.,1.,1.,1.,1.,
1.,1.,1.,1.,1.,1.,1.,1.,1.,1.,1.,1.,1.,1.,1.,1.,1.,1.,1.,1.,1.,1.,1.,1.,
1.,1.,1.,1.,1.,1.,1.,1.,1.,1.,1.,1.,1.,1.,1.,1.,1.,1.,1.,1.,1.,1.,1.,1.,
1.,1.,1.,1.,1.,1.))
REPRESENTATION_ITEM('')
);
#125=(
BOUNDED_CURVE()
B_SPLINE_CURVE(5,(#33265,#33266,#33267,#33268,#33269,#33270,#33271,#33272,
#33273,#33274,#33275,#33276,#33277,#33278,#33279,#33280,#33281,#33282,#33283,
#33284,#33285,#33286,#33287,#33288,#33289,#33290,#33291,#33292,#33293,#33294,
#33295,#33296,#33297,#33298,#33299,#33300,#33301,#33302,#33303,#33304,#33305,
#33306,#33307,#33308,#33309,#33310,#33311,#33312,#33313,#33314,#33315,#33316,
#33317,#33318,#33319,#33320,#33321,#33322,#33323,#33324,#33325,#33326,#33327,
#33328,#33329,#33330,#33331,#33332,#33333,#33334),.UNSPECIFIED.,.F.,.F.)
B_SPLINE_CURVE_WITH_KNOTS((6,1,1,1,1,1,1,1,1,1,1,1,1,1,1,1,1,1,1,1,1,1,
1,1,1,1,1,1,1,1,1,1,1,1,1,1,1,1,1,1,1,1,1,1,1,1,1,1,1,1,1,1,1,1,1,1,1,1,
1,1,1,1,1,1,1,6),(-1.,-0.984615384615383,-0.969230769230768,-0.953846153846152,
-0.938461538461537,-0.923076923076922,-0.907692307692306,-0.892307692307691,
-0.876923076923076,-0.86153846153846,-0.846153846153845,-0.83076923076923,
-0.815384615384614,-0.799999999999999,-0.784615384615384,-0.769230769230768,
-0.753846153846153,-0.738461538461538,-0.723076923076922,-0.707692307692307,
-0.692307692307692,-0.676923076923076,-0.661538461538461,-0.646153846153846,
-0.63076923076923,-0.615384615384615,-0.6,-0.584615384615384,-0.569230769230769,
-0.553846153846154,-0.538461538461538,-0.523076923076923,-0.507692307692308,
-0.492307692307692,-0.476923076923077,-0.461538461538462,-0.446153846153846,
-0.430769230769231,-0.415384615384615,-0.4,-0.384615384615385,-0.369230769230769,
-0.353846153846154,-0.338461538461538,-0.323076923076923,-0.307692307692308,
-0.292307692307692,-0.276923076923077,-0.261538461538462,-0.246153846153846,
-0.230769230769231,-0.215384615384615,-0.2,-0.184615384615385,-0.169230769230769,
-0.153846153846154,-0.138461538461538,-0.123076923076923,-0.107692307692308,
-0.0923076923076923,-0.0769230769230769,-0.0615384615384615,-0.0461538461538462,
-0.0307692307692308,-0.0153846153846154,0.),.UNSPECIFIED.)
CURVE()
GEOMETRIC_REPRESENTATION_ITEM()
RATIONAL_B_SPLINE_CURVE((1.,1.,1.,1.,1.,1.,1.,1.,1.,1.,1.,1.,1.,1.,1.,1.,
1.,1.,1.,1.,1.,1.,1.,1.,1.,1.,1.,1.,1.,1.,1.,1.,1.,1.,1.,1.,1.,1.,1.,1.,
1.,1.,1.,1.,1.,1.,1.,1.,1.,1.,1.,1.,1.,1.,1.,1.,1.,1.,1.,1.,1.,1.,1.,1.,
1.,1.,1.,1.,1.,1.))
REPRESENTATION_ITEM('')
);
#126=(
BOUNDED_CURVE()
B_SPLINE_CURVE(5,(#33481,#33482,#33483,#33484,#33485,#33486,#33487,#33488,
#33489,#33490,#33491,#33492,#33493,#33494,#33495,#33496,#33497,#33498,#33499,
#33500,#33501,#33502,#33503,#33504,#33505,#33506,#33507,#33508,#33509,#33510,
#33511,#33512,#33513,#33514,#33515,#33516,#33517,#33518,#33519,#33520,#33521,
#33522,#33523,#33524,#33525,#33526,#33527,#33528,#33529,#33530,#33531,#33532,
#33533,#33534,#33535,#33536,#33537,#33538,#33539,#33540,#33541,#33542,#33543,
#33544,#33545,#33546,#33547,#33548,#33549,#33550),.UNSPECIFIED.,.F.,.F.)
B_SPLINE_CURVE_WITH_KNOTS((6,1,1,1,1,1,1,1,1,1,1,1,1,1,1,1,1,1,1,1,1,1,
1,1,1,1,1,1,1,1,1,1,1,1,1,1,1,1,1,1,1,1,1,1,1,1,1,1,1,1,1,1,1,1,1,1,1,1,
1,1,1,1,1,1,1,6),(-1.,-0.984615384615383,-0.969230769230768,-0.953846153846152,
-0.938461538461537,-0.923076923076922,-0.907692307692306,-0.892307692307691,
-0.876923076923076,-0.86153846153846,-0.846153846153845,-0.83076923076923,
-0.815384615384614,-0.799999999999999,-0.784615384615384,-0.769230769230768,
-0.753846153846153,-0.738461538461538,-0.723076923076922,-0.707692307692307,
-0.692307692307692,-0.676923076923076,-0.661538461538461,-0.646153846153846,
-0.63076923076923,-0.615384615384615,-0.6,-0.584615384615384,-0.569230769230769,
-0.553846153846154,-0.538461538461538,-0.523076923076923,-0.507692307692308,
-0.492307692307692,-0.476923076923077,-0.461538461538462,-0.446153846153846,
-0.430769230769231,-0.415384615384615,-0.4,-0.384615384615385,-0.369230769230769,
-0.353846153846154,-0.338461538461538,-0.323076923076923,-0.307692307692308,
-0.292307692307692,-0.276923076923077,-0.261538461538462,-0.246153846153846,
-0.230769230769231,-0.215384615384615,-0.2,-0.184615384615385,-0.169230769230769,
-0.153846153846154,-0.138461538461538,-0.123076923076923,-0.107692307692308,
-0.0923076923076923,-0.0769230769230769,-0.0615384615384615,-0.0461538461538462,
-0.0307692307692308,-0.0153846153846154,0.),.UNSPECIFIED.)
CURVE()
GEOMETRIC_REPRESENTATION_ITEM()
RATIONAL_B_SPLINE_CURVE((1.,1.,1.,1.,1.,1.,1.,1.,1.,1.,1.,1.,1.,1.,1.,1.,
1.,1.,1.,1.,1.,1.,1.,1.,1.,1.,1.,1.,1.,1.,1.,1.,1.,1.,1.,1.,1.,1.,1.,1.,
1.,1.,1.,1.,1.,1.,1.,1.,1.,1.,1.,1.,1.,1.,1.,1.,1.,1.,1.,1.,1.,1.,1.,1.,
1.,1.,1.,1.,1.,1.))
REPRESENTATION_ITEM('')
);
#127=(
BOUNDED_CURVE()
B_SPLINE_CURVE(5,(#33697,#33698,#33699,#33700,#33701,#33702,#33703,#33704,
#33705,#33706,#33707,#33708,#33709,#33710,#33711,#33712,#33713,#33714,#33715,
#33716,#33717,#33718,#33719,#33720,#33721,#33722,#33723,#33724,#33725,#33726,
#33727,#33728,#33729,#33730,#33731,#33732,#33733,#33734,#33735,#33736,#33737,
#33738,#33739,#33740,#33741,#33742,#33743,#33744,#33745,#33746,#33747,#33748,
#33749,#33750,#33751,#33752,#33753,#33754,#33755,#33756,#33757,#33758,#33759,
#33760,#33761,#33762,#33763,#33764,#33765,#33766),.UNSPECIFIED.,.F.,.F.)
B_SPLINE_CURVE_WITH_KNOTS((6,1,1,1,1,1,1,1,1,1,1,1,1,1,1,1,1,1,1,1,1,1,
1,1,1,1,1,1,1,1,1,1,1,1,1,1,1,1,1,1,1,1,1,1,1,1,1,1,1,1,1,1,1,1,1,1,1,1,
1,1,1,1,1,1,1,6),(-1.,-0.984615384615383,-0.969230769230768,-0.953846153846152,
-0.938461538461537,-0.923076923076922,-0.907692307692306,-0.892307692307691,
-0.876923076923076,-0.86153846153846,-0.846153846153845,-0.83076923076923,
-0.815384615384614,-0.799999999999999,-0.784615384615384,-0.769230769230768,
-0.753846153846153,-0.738461538461538,-0.723076923076922,-0.707692307692307,
-0.692307692307692,-0.676923076923076,-0.661538461538461,-0.646153846153846,
-0.63076923076923,-0.615384615384615,-0.6,-0.584615384615384,-0.569230769230769,
-0.553846153846154,-0.538461538461538,-0.523076923076923,-0.507692307692308,
-0.492307692307692,-0.476923076923077,-0.461538461538462,-0.446153846153846,
-0.430769230769231,-0.415384615384615,-0.4,-0.384615384615385,-0.369230769230769,
-0.353846153846154,-0.338461538461538,-0.323076923076923,-0.307692307692308,
-0.292307692307692,-0.276923076923077,-0.261538461538462,-0.246153846153846,
-0.230769230769231,-0.215384615384615,-0.2,-0.184615384615385,-0.169230769230769,
-0.153846153846154,-0.138461538461538,-0.123076923076923,-0.107692307692308,
-0.0923076923076923,-0.0769230769230769,-0.0615384615384615,-0.0461538461538462,
-0.0307692307692308,-0.0153846153846154,0.),.UNSPECIFIED.)
CURVE()
GEOMETRIC_REPRESENTATION_ITEM()
RATIONAL_B_SPLINE_CURVE((1.,1.,1.,1.,1.,1.,1.,1.,1.,1.,1.,1.,1.,1.,1.,1.,
1.,1.,1.,1.,1.,1.,1.,1.,1.,1.,1.,1.,1.,1.,1.,1.,1.,1.,1.,1.,1.,1.,1.,1.,
1.,1.,1.,1.,1.,1.,1.,1.,1.,1.,1.,1.,1.,1.,1.,1.,1.,1.,1.,1.,1.,1.,1.,1.,
1.,1.,1.,1.,1.,1.))
REPRESENTATION_ITEM('')
);
#128=(
BOUNDED_CURVE()
B_SPLINE_CURVE(5,(#33913,#33914,#33915,#33916,#33917,#33918,#33919,#33920,
#33921,#33922,#33923,#33924,#33925,#33926,#33927,#33928,#33929,#33930,#33931,
#33932,#33933,#33934,#33935,#33936,#33937,#33938,#33939,#33940,#33941,#33942,
#33943,#33944,#33945,#33946,#33947,#33948,#33949,#33950,#33951,#33952,#33953,
#33954,#33955,#33956,#33957,#33958,#33959,#33960,#33961,#33962,#33963,#33964,
#33965,#33966,#33967,#33968,#33969,#33970,#33971,#33972,#33973,#33974,#33975,
#33976,#33977,#33978,#33979,#33980,#33981,#33982),.UNSPECIFIED.,.F.,.F.)
B_SPLINE_CURVE_WITH_KNOTS((6,1,1,1,1,1,1,1,1,1,1,1,1,1,1,1,1,1,1,1,1,1,
1,1,1,1,1,1,1,1,1,1,1,1,1,1,1,1,1,1,1,1,1,1,1,1,1,1,1,1,1,1,1,1,1,1,1,1,
1,1,1,1,1,1,1,6),(-1.,-0.984615384615383,-0.969230769230768,-0.953846153846152,
-0.938461538461537,-0.923076923076922,-0.907692307692306,-0.892307692307691,
-0.876923076923076,-0.86153846153846,-0.846153846153845,-0.83076923076923,
-0.815384615384614,-0.799999999999999,-0.784615384615384,-0.769230769230768,
-0.753846153846153,-0.738461538461538,-0.723076923076922,-0.707692307692307,
-0.692307692307692,-0.676923076923076,-0.661538461538461,-0.646153846153846,
-0.63076923076923,-0.615384615384615,-0.6,-0.584615384615384,-0.569230769230769,
-0.553846153846154,-0.538461538461538,-0.523076923076923,-0.507692307692308,
-0.492307692307692,-0.476923076923077,-0.461538461538462,-0.446153846153846,
-0.430769230769231,-0.415384615384615,-0.4,-0.384615384615385,-0.369230769230769,
-0.353846153846154,-0.338461538461538,-0.323076923076923,-0.307692307692308,
-0.292307692307692,-0.276923076923077,-0.261538461538462,-0.246153846153846,
-0.230769230769231,-0.215384615384615,-0.2,-0.184615384615385,-0.169230769230769,
-0.153846153846154,-0.138461538461538,-0.123076923076923,-0.107692307692308,
-0.0923076923076923,-0.0769230769230769,-0.0615384615384615,-0.0461538461538462,
-0.0307692307692308,-0.0153846153846154,0.),.UNSPECIFIED.)
CURVE()
GEOMETRIC_REPRESENTATION_ITEM()
RATIONAL_B_SPLINE_CURVE((1.,1.,1.,1.,1.,1.,1.,1.,1.,1.,1.,1.,1.,1.,1.,1.,
1.,1.,1.,1.,1.,1.,1.,1.,1.,1.,1.,1.,1.,1.,1.,1.,1.,1.,1.,1.,1.,1.,1.,1.,
1.,1.,1.,1.,1.,1.,1.,1.,1.,1.,1.,1.,1.,1.,1.,1.,1.,1.,1.,1.,1.,1.,1.,1.,
1.,1.,1.,1.,1.,1.))
REPRESENTATION_ITEM('')
);
#129=(
BOUNDED_CURVE()
B_SPLINE_CURVE(5,(#34129,#34130,#34131,#34132,#34133,#34134,#34135,#34136,
#34137,#34138,#34139,#34140,#34141,#34142,#34143,#34144,#34145,#34146,#34147,
#34148,#34149,#34150,#34151,#34152,#34153,#34154,#34155,#34156,#34157,#34158,
#34159,#34160,#34161,#34162,#34163,#34164,#34165,#34166,#34167,#34168,#34169,
#34170,#34171,#34172,#34173,#34174,#34175,#34176,#34177,#34178,#34179,#34180,
#34181,#34182,#34183,#34184,#34185,#34186,#34187,#34188,#34189,#34190,#34191,
#34192,#34193,#34194,#34195,#34196,#34197,#34198),.UNSPECIFIED.,.F.,.F.)
B_SPLINE_CURVE_WITH_KNOTS((6,1,1,1,1,1,1,1,1,1,1,1,1,1,1,1,1,1,1,1,1,1,
1,1,1,1,1,1,1,1,1,1,1,1,1,1,1,1,1,1,1,1,1,1,1,1,1,1,1,1,1,1,1,1,1,1,1,1,
1,1,1,1,1,1,1,6),(-1.,-0.984615384615383,-0.969230769230768,-0.953846153846152,
-0.938461538461537,-0.923076923076922,-0.907692307692306,-0.892307692307691,
-0.876923076923076,-0.86153846153846,-0.846153846153845,-0.83076923076923,
-0.815384615384614,-0.799999999999999,-0.784615384615384,-0.769230769230768,
-0.753846153846153,-0.738461538461538,-0.723076923076922,-0.707692307692307,
-0.692307692307692,-0.676923076923076,-0.661538461538461,-0.646153846153846,
-0.63076923076923,-0.615384615384615,-0.6,-0.584615384615384,-0.569230769230769,
-0.553846153846154,-0.538461538461538,-0.523076923076923,-0.507692307692308,
-0.492307692307692,-0.476923076923077,-0.461538461538462,-0.446153846153846,
-0.430769230769231,-0.415384615384615,-0.4,-0.384615384615385,-0.369230769230769,
-0.353846153846154,-0.338461538461538,-0.323076923076923,-0.307692307692308,
-0.292307692307692,-0.276923076923077,-0.261538461538462,-0.246153846153846,
-0.230769230769231,-0.215384615384615,-0.2,-0.184615384615385,-0.169230769230769,
-0.153846153846154,-0.138461538461538,-0.123076923076923,-0.107692307692308,
-0.0923076923076923,-0.0769230769230769,-0.0615384615384615,-0.0461538461538462,
-0.0307692307692308,-0.0153846153846154,0.),.UNSPECIFIED.)
CURVE()
GEOMETRIC_REPRESENTATION_ITEM()
RATIONAL_B_SPLINE_CURVE((1.,1.,1.,1.,1.,1.,1.,1.,1.,1.,1.,1.,1.,1.,1.,1.,
1.,1.,1.,1.,1.,1.,1.,1.,1.,1.,1.,1.,1.,1.,1.,1.,1.,1.,1.,1.,1.,1.,1.,1.,
1.,1.,1.,1.,1.,1.,1.,1.,1.,1.,1.,1.,1.,1.,1.,1.,1.,1.,1.,1.,1.,1.,1.,1.,
1.,1.,1.,1.,1.,1.))
REPRESENTATION_ITEM('')
);
#130=(
BOUNDED_CURVE()
B_SPLINE_CURVE(5,(#34345,#34346,#34347,#34348,#34349,#34350,#34351,#34352,
#34353,#34354,#34355,#34356,#34357,#34358,#34359,#34360,#34361,#34362,#34363,
#34364,#34365,#34366,#34367,#34368,#34369,#34370,#34371,#34372,#34373,#34374,
#34375,#34376,#34377,#34378,#34379,#34380,#34381,#34382,#34383,#34384,#34385,
#34386,#34387,#34388,#34389,#34390,#34391,#34392,#34393,#34394,#34395,#34396,
#34397,#34398,#34399,#34400,#34401,#34402,#34403,#34404,#34405,#34406,#34407,
#34408,#34409,#34410,#34411,#34412,#34413,#34414),.UNSPECIFIED.,.F.,.F.)
B_SPLINE_CURVE_WITH_KNOTS((6,1,1,1,1,1,1,1,1,1,1,1,1,1,1,1,1,1,1,1,1,1,
1,1,1,1,1,1,1,1,1,1,1,1,1,1,1,1,1,1,1,1,1,1,1,1,1,1,1,1,1,1,1,1,1,1,1,1,
1,1,1,1,1,1,1,6),(-1.,-0.984615384615383,-0.969230769230768,-0.953846153846152,
-0.938461538461537,-0.923076923076922,-0.907692307692306,-0.892307692307691,
-0.876923076923076,-0.86153846153846,-0.846153846153845,-0.83076923076923,
-0.815384615384614,-0.799999999999999,-0.784615384615384,-0.769230769230768,
-0.753846153846153,-0.738461538461538,-0.723076923076922,-0.707692307692307,
-0.692307692307692,-0.676923076923076,-0.661538461538461,-0.646153846153846,
-0.63076923076923,-0.615384615384615,-0.6,-0.584615384615384,-0.569230769230769,
-0.553846153846154,-0.538461538461538,-0.523076923076923,-0.507692307692308,
-0.492307692307692,-0.476923076923077,-0.461538461538462,-0.446153846153846,
-0.430769230769231,-0.415384615384615,-0.4,-0.384615384615385,-0.369230769230769,
-0.353846153846154,-0.338461538461538,-0.323076923076923,-0.307692307692308,
-0.292307692307692,-0.276923076923077,-0.261538461538462,-0.246153846153846,
-0.230769230769231,-0.215384615384615,-0.2,-0.184615384615385,-0.169230769230769,
-0.153846153846154,-0.138461538461538,-0.123076923076923,-0.107692307692308,
-0.0923076923076923,-0.0769230769230769,-0.0615384615384615,-0.0461538461538462,
-0.0307692307692308,-0.0153846153846154,0.),.UNSPECIFIED.)
CURVE()
GEOMETRIC_REPRESENTATION_ITEM()
RATIONAL_B_SPLINE_CURVE((1.,1.,1.,1.,1.,1.,1.,1.,1.,1.,1.,1.,1.,1.,1.,1.,
1.,1.,1.,1.,1.,1.,1.,1.,1.,1.,1.,1.,1.,1.,1.,1.,1.,1.,1.,1.,1.,1.,1.,1.,
1.,1.,1.,1.,1.,1.,1.,1.,1.,1.,1.,1.,1.,1.,1.,1.,1.,1.,1.,1.,1.,1.,1.,1.,
1.,1.,1.,1.,1.,1.))
REPRESENTATION_ITEM('')
);
#680=SHAPE_REPRESENTATION_RELATIONSHIP('SRR','None',#35119,#726);
#726=ADVANCED_BREP_SHAPE_REPRESENTATION('',(#829),#34844);
#779=STYLED_ITEM('',(#35425),#829);
#829=MANIFOLD_SOLID_BREP('Body1',#13802);
#1035=FACE_BOUND('',#3079,.T.);
#1036=FACE_BOUND('',#3083,.T.);
#1037=FACE_BOUND('',#3164,.T.);
#1473=PLANE('',#15323);
#1474=PLANE('',#15324);
#1475=PLANE('',#15325);
#1476=PLANE('',#15326);
#1477=PLANE('',#15353);
#1478=PLANE('',#15354);
#1479=PLANE('',#15357);
#1480=PLANE('',#15360);
#1481=PLANE('',#15363);
#1482=PLANE('',#15366);
#1483=PLANE('',#15369);
#1484=PLANE('',#15372);
#1485=PLANE('',#15375);
#1486=PLANE('',#15378);
#1487=PLANE('',#15381);
#1488=PLANE('',#15384);
#1489=PLANE('',#15387);
#1490=PLANE('',#15390);
#1491=PLANE('',#15393);
#1492=PLANE('',#15396);
#1493=PLANE('',#15399);
#1494=PLANE('',#15402);
#1495=PLANE('',#15405);
#1496=PLANE('',#15408);
#1497=PLANE('',#15411);
#1498=PLANE('',#15412);
#2134=FACE_OUTER_BOUND('',#3075,.T.);
#2135=FACE_OUTER_BOUND('',#3076,.T.);
#2136=FACE_OUTER_BOUND('',#3077,.T.);
#2137=FACE_OUTER_BOUND('',#3078,.T.);
#2138=FACE_OUTER_BOUND('',#3080,.T.);
#2139=FACE_OUTER_BOUND('',#3081,.T.);
#2140=FACE_OUTER_BOUND('',#3082,.T.);
#2141=FACE_OUTER_BOUND('',#3084,.T.);
#2142=FACE_OUTER_BOUND('',#3085,.T.);
#2143=FACE_OUTER_BOUND('',#3086,.T.);
#2144=FACE_OUTER_BOUND('',#3087,.T.);
#2145=FACE_OUTER_BOUND('',#3088,.T.);
#2146=FACE_OUTER_BOUND('',#3089,.T.);
#2147=FACE_OUTER_BOUND('',#3090,.T.);
#2148=FACE_OUTER_BOUND('',#3091,.T.);
#2149=FACE_OUTER_BOUND('',#3092,.T.);
#2150=FACE_OUTER_BOUND('',#3093,.T.);
#2151=FACE_OUTER_BOUND('',#3094,.T.);
#2152=FACE_OUTER_BOUND('',#3095,.T.);
#2153=FACE_OUTER_BOUND('',#3096,.T.);
#2154=FACE_OUTER_BOUND('',#3097,.T.);
#2155=FACE_OUTER_BOUND('',#3098,.T.);
#2156=FACE_OUTER_BOUND('',#3099,.T.);
#2157=FACE_OUTER_BOUND('',#3100,.T.);
#2158=FACE_OUTER_BOUND('',#3101,.T.);
#2159=FACE_OUTER_BOUND('',#3102,.T.);
#2160=FACE_OUTER_BOUND('',#3103,.T.);
#2161=FACE_OUTER_BOUND('',#3104,.T.);
#2162=FACE_OUTER_BOUND('',#3105,.T.);
#2163=FACE_OUTER_BOUND('',#3106,.T.);
#2164=FACE_OUTER_BOUND('',#3107,.T.);
#2165=FACE_OUTER_BOUND('',#3108,.T.);
#2166=FACE_OUTER_BOUND('',#3109,.T.);
#2167=FACE_OUTER_BOUND('',#3110,.T.);
#2168=FACE_OUTER_BOUND('',#3111,.T.);
#2169=FACE_OUTER_BOUND('',#3112,.T.);
#2170=FACE_OUTER_BOUND('',#3113,.T.);
#2171=FACE_OUTER_BOUND('',#3114,.T.);
#2172=FACE_OUTER_BOUND('',#3115,.T.);
#2173=FACE_OUTER_BOUND('',#3116,.T.);
#2174=FACE_OUTER_BOUND('',#3117,.T.);
#2175=FACE_OUTER_BOUND('',#3118,.T.);
#2176=FACE_OUTER_BOUND('',#3119,.T.);
#2177=FACE_OUTER_BOUND('',#3120,.T.);
#2178=FACE_OUTER_BOUND('',#3121,.T.);
#2179=FACE_OUTER_BOUND('',#3122,.T.);
#2180=FACE_OUTER_BOUND('',#3123,.T.);
#2181=FACE_OUTER_BOUND('',#3124,.T.);
#2182=FACE_OUTER_BOUND('',#3125,.T.);
#2183=FACE_OUTER_BOUND('',#3126,.T.);
#2184=FACE_OUTER_BOUND('',#3127,.T.);
#2185=FACE_OUTER_BOUND('',#3128,.T.);
#2186=FACE_OUTER_BOUND('',#3129,.T.);
#2187=FACE_OUTER_BOUND('',#3130,.T.);
#2188=FACE_OUTER_BOUND('',#3131,.T.);
#2189=FACE_OUTER_BOUND('',#3132,.T.);
#2190=FACE_OUTER_BOUND('',#3133,.T.);
#2191=FACE_OUTER_BOUND('',#3134,.T.);
#2192=FACE_OUTER_BOUND('',#3135,.T.);
#2193=FACE_OUTER_BOUND('',#3136,.T.);
#2194=FACE_OUTER_BOUND('',#3137,.T.);
#2195=FACE_OUTER_BOUND('',#3138,.T.);
#2196=FACE_OUTER_BOUND('',#3139,.T.);
#2197=FACE_OUTER_BOUND('',#3140,.T.);
#2198=FACE_OUTER_BOUND('',#3141,.T.);
#2199=FACE_OUTER_BOUND('',#3142,.T.);
#2200=FACE_OUTER_BOUND('',#3143,.T.);
#2201=FACE_OUTER_BOUND('',#3144,.T.);
#2202=FACE_OUTER_BOUND('',#3145,.T.);
#2203=FACE_OUTER_BOUND('',#3146,.T.);
#2204=FACE_OUTER_BOUND('',#3147,.T.);
#2205=FACE_OUTER_BOUND('',#3148,.T.);
#2206=FACE_OUTER_BOUND('',#3149,.T.);
#2207=FACE_OUTER_BOUND('',#3150,.T.);
#2208=FACE_OUTER_BOUND('',#3151,.T.);
#2209=FACE_OUTER_BOUND('',#3152,.T.);
#2210=FACE_OUTER_BOUND('',#3153,.T.);
#2211=FACE_OUTER_BOUND('',#3154,.T.);
#2212=FACE_OUTER_BOUND('',#3155,.T.);
#2213=FACE_OUTER_BOUND('',#3156,.T.);
#2214=FACE_OUTER_BOUND('',#3157,.T.);
#2215=FACE_OUTER_BOUND('',#3158,.T.);
#2216=FACE_OUTER_BOUND('',#3159,.T.);
#2217=FACE_OUTER_BOUND('',#3160,.T.);
#2218=FACE_OUTER_BOUND('',#3161,.T.);
#2219=FACE_OUTER_BOUND('',#3162,.T.);
#2220=FACE_OUTER_BOUND('',#3163,.T.);
#2221=FACE_OUTER_BOUND('',#3165,.T.);
#3075=EDGE_LOOP('',(#12134,#12135,#12136,#12137));
#3076=EDGE_LOOP('',(#12138,#12139,#12140,#12141));
#3077=EDGE_LOOP('',(#12142,#12143,#12144,#12145));
#3078=EDGE_LOOP('',(#12146,#12147,#12148,#12149,#12150,#12151,#12152,#12153,
#12154,#12155,#12156,#12157,#12158,#12159,#12160,#12161,#12162,#12163,#12164,
#12165,#12166,#12167,#12168,#12169,#12170,#12171,#12172,#12173,#12174,#12175,
#12176,#12177,#12178,#12179,#12180,#12181,#12182,#12183,#12184,#12185,#12186,
#12187,#12188,#12189,#12190,#12191,#12192,#12193,#12194,#12195,#12196,#12197,
#12198,#12199,#12200,#12201,#12202,#12203,#12204,#12205,#12206,#12207,#12208,
#12209,#12210,#12211,#12212,#12213,#12214,#12215,#12216,#12217,#12218,#12219,
#12220,#12221,#12222,#12223,#12224,#12225));
#3079=EDGE_LOOP('',(#12226,#12227,#12228,#12229));
#3080=EDGE_LOOP('',(#12230,#12231,#12232,#12233));
#3081=EDGE_LOOP('',(#12234,#12235,#12236,#12237));
#3082=EDGE_LOOP('',(#12238));
#3083=EDGE_LOOP('',(#12239,#12240,#12241,#12242));
#3084=EDGE_LOOP('',(#12243,#12244,#12245,#12246));
#3085=EDGE_LOOP('',(#12247,#12248,#12249,#12250));
#3086=EDGE_LOOP('',(#12251,#12252,#12253,#12254));
#3087=EDGE_LOOP('',(#12255,#12256,#12257,#12258));
#3088=EDGE_LOOP('',(#12259,#12260,#12261,#12262));
#3089=EDGE_LOOP('',(#12263,#12264,#12265,#12266));
#3090=EDGE_LOOP('',(#12267,#12268,#12269,#12270));
#3091=EDGE_LOOP('',(#12271,#12272,#12273,#12274));
#3092=EDGE_LOOP('',(#12275,#12276,#12277,#12278));
#3093=EDGE_LOOP('',(#12279,#12280,#12281,#12282));
#3094=EDGE_LOOP('',(#12283,#12284,#12285,#12286));
#3095=EDGE_LOOP('',(#12287,#12288,#12289,#12290));
#3096=EDGE_LOOP('',(#12291,#12292,#12293,#12294));
#3097=EDGE_LOOP('',(#12295,#12296,#12297,#12298));
#3098=EDGE_LOOP('',(#12299,#12300,#12301,#12302));
#3099=EDGE_LOOP('',(#12303,#12304,#12305,#12306));
#3100=EDGE_LOOP('',(#12307,#12308,#12309,#12310));
#3101=EDGE_LOOP('',(#12311,#12312,#12313,#12314));
#3102=EDGE_LOOP('',(#12315,#12316,#12317,#12318));
#3103=EDGE_LOOP('',(#12319,#12320,#12321,#12322));
#3104=EDGE_LOOP('',(#12323,#12324,#12325,#12326));
#3105=EDGE_LOOP('',(#12327,#12328,#12329,#12330));
#3106=EDGE_LOOP('',(#12331,#12332,#12333,#12334));
#3107=EDGE_LOOP('',(#12335,#12336,#12337,#12338));
#3108=EDGE_LOOP('',(#12339,#12340,#12341,#12342));
#3109=EDGE_LOOP('',(#12343,#12344,#12345,#12346));
#3110=EDGE_LOOP('',(#12347,#12348,#12349,#12350));
#3111=EDGE_LOOP('',(#12351,#12352,#12353,#12354));
#3112=EDGE_LOOP('',(#12355,#12356,#12357,#12358));
#3113=EDGE_LOOP('',(#12359,#12360,#12361,#12362));
#3114=EDGE_LOOP('',(#12363,#12364,#12365,#12366));
#3115=EDGE_LOOP('',(#12367,#12368,#12369,#12370));
#3116=EDGE_LOOP('',(#12371,#12372,#12373,#12374));
#3117=EDGE_LOOP('',(#12375,#12376,#12377,#12378));
#3118=EDGE_LOOP('',(#12379,#12380,#12381,#12382));
#3119=EDGE_LOOP('',(#12383,#12384,#12385,#12386));
#3120=EDGE_LOOP('',(#12387,#12388,#12389,#12390));
#3121=EDGE_LOOP('',(#12391,#12392,#12393,#12394));
#3122=EDGE_LOOP('',(#12395,#12396,#12397,#12398));
#3123=EDGE_LOOP('',(#12399,#12400,#12401,#12402));
#3124=EDGE_LOOP('',(#12403,#12404,#12405,#12406));
#3125=EDGE_LOOP('',(#12407,#12408,#12409,#12410));
#3126=EDGE_LOOP('',(#12411,#12412,#12413,#12414));
#3127=EDGE_LOOP('',(#12415,#12416,#12417,#12418));
#3128=EDGE_LOOP('',(#12419,#12420,#12421,#12422));
#3129=EDGE_LOOP('',(#12423,#12424,#12425,#12426));
#3130=EDGE_LOOP('',(#12427,#12428,#12429,#12430));
#3131=EDGE_LOOP('',(#12431,#12432,#12433,#12434));
#3132=EDGE_LOOP('',(#12435,#12436,#12437,#12438));
#3133=EDGE_LOOP('',(#12439,#12440,#12441,#12442));
#3134=EDGE_LOOP('',(#12443,#12444,#12445,#12446));
#3135=EDGE_LOOP('',(#12447,#12448,#12449,#12450));
#3136=EDGE_LOOP('',(#12451,#12452,#12453,#12454));
#3137=EDGE_LOOP('',(#12455,#12456,#12457,#12458));
#3138=EDGE_LOOP('',(#12459,#12460,#12461,#12462));
#3139=EDGE_LOOP('',(#12463,#12464,#12465,#12466));
#3140=EDGE_LOOP('',(#12467,#12468,#12469,#12470));
#3141=EDGE_LOOP('',(#12471,#12472,#12473,#12474));
#3142=EDGE_LOOP('',(#12475,#12476,#12477,#12478));
#3143=EDGE_LOOP('',(#12479,#12480,#12481,#12482));
#3144=EDGE_LOOP('',(#12483,#12484,#12485,#12486));
#3145=EDGE_LOOP('',(#12487,#12488,#12489,#12490));
#3146=EDGE_LOOP('',(#12491,#12492,#12493,#12494));
#3147=EDGE_LOOP('',(#12495,#12496,#12497,#12498));
#3148=EDGE_LOOP('',(#12499,#12500,#12501,#12502));
#3149=EDGE_LOOP('',(#12503,#12504,#12505,#12506));
#3150=EDGE_LOOP('',(#12507,#12508,#12509,#12510));
#3151=EDGE_LOOP('',(#12511,#12512,#12513,#12514));
#3152=EDGE_LOOP('',(#12515,#12516,#12517,#12518));
#3153=EDGE_LOOP('',(#12519,#12520,#12521,#12522));
#3154=EDGE_LOOP('',(#12523,#12524,#12525,#12526));
#3155=EDGE_LOOP('',(#12527,#12528,#12529,#12530));
#3156=EDGE_LOOP('',(#12531,#12532,#12533,#12534));
#3157=EDGE_LOOP('',(#12535,#12536,#12537,#12538));
#3158=EDGE_LOOP('',(#12539,#12540,#12541,#12542));
#3159=EDGE_LOOP('',(#12543,#12544,#12545,#12546));
#3160=EDGE_LOOP('',(#12547,#12548,#12549,#12550));
#3161=EDGE_LOOP('',(#12551,#12552,#12553,#12554));
#3162=EDGE_LOOP('',(#12555,#12556,#12557,#12558));
#3163=EDGE_LOOP('',(#12559,#12560,#12561,#12562,#12563,#12564,#12565,#12566,
#12567,#12568,#12569,#12570,#12571,#12572,#12573,#12574,#12575,#12576,#12577,
#12578,#12579,#12580,#12581,#12582,#12583,#12584,#12585,#12586,#12587,#12588,
#12589,#12590,#12591,#12592,#12593,#12594,#12595,#12596,#12597,#12598,#12599,
#12600,#12601,#12602,#12603,#12604,#12605,#12606,#12607,#12608,#12609,#12610,
#12611,#12612,#12613,#12614,#12615,#12616,#12617,#12618,#12619,#12620,#12621,
#12622,#12623,#12624,#12625,#12626,#12627,#12628,#12629,#12630,#12631,#12632,
#12633,#12634,#12635,#12636,#12637,#12638));
#3164=EDGE_LOOP('',(#12639));
#3165=EDGE_LOOP('',(#12640,#12641,#12642,#12643));
#4308=LINE('',#22829,#5599);
#4309=LINE('',#22831,#5600);
#4310=LINE('',#22833,#5601);
#4311=LINE('',#22834,#5602);
#4312=LINE('',#22837,#5603);
#4313=LINE('',#22839,#5604);
#4314=LINE('',#22840,#5605);
#4315=LINE('',#22843,#5606);
#4316=LINE('',#22845,#5607);
#4317=LINE('',#22846,#5608);
#4318=LINE('',#22923,#5609);
#4319=LINE('',#23069,#5610);
#4320=LINE('',#23215,#5611);
#4321=LINE('',#23361,#5612);
#4322=LINE('',#23507,#5613);
#4323=LINE('',#23653,#5614);
#4324=LINE('',#23799,#5615);
#4325=LINE('',#23945,#5616);
#4326=LINE('',#24091,#5617);
#4327=LINE('',#24237,#5618);
#4328=LINE('',#24383,#5619);
#4329=LINE('',#24529,#5620);
#4330=LINE('',#24675,#5621);
#4331=LINE('',#24821,#5622);
#4332=LINE('',#24967,#5623);
#4333=LINE('',#25113,#5624);
#4334=LINE('',#25259,#5625);
#4335=LINE('',#25405,#5626);
#4336=LINE('',#25551,#5627);
#4337=LINE('',#25697,#5628);
#4338=LINE('',#25775,#5629);
#4339=LINE('',#25919,#5630);
#4340=LINE('',#25991,#5631);
#4341=LINE('',#25994,#5632);
#4342=LINE('',#25995,#5633);
#4343=LINE('',#26207,#5634);
#4344=LINE('',#26211,#5635);
#4345=LINE('',#26423,#5636);
#4346=LINE('',#26426,#5637);
#4347=LINE('',#26427,#5638);
#4348=LINE('',#26639,#5639);
#4349=LINE('',#26643,#5640);
#4350=LINE('',#26855,#5641);
#4351=LINE('',#26858,#5642);
#4352=LINE('',#26859,#5643);
#4353=LINE('',#27071,#5644);
#4354=LINE('',#27075,#5645);
#4355=LINE('',#27287,#5646);
#4356=LINE('',#27290,#5647);
#4357=LINE('',#27291,#5648);
#4358=LINE('',#27503,#5649);
#4359=LINE('',#27507,#5650);
#4360=LINE('',#27719,#5651);
#4361=LINE('',#27722,#5652);
#4362=LINE('',#27723,#5653);
#4363=LINE('',#27935,#5654);
#4364=LINE('',#27939,#5655);
#4365=LINE('',#28151,#5656);
#4366=LINE('',#28154,#5657);
#4367=LINE('',#28155,#5658);
#4368=LINE('',#28367,#5659);
#4369=LINE('',#28371,#5660);
#4370=LINE('',#28583,#5661);
#4371=LINE('',#28586,#5662);
#4372=LINE('',#28587,#5663);
#4373=LINE('',#28799,#5664);
#4374=LINE('',#28803,#5665);
#4375=LINE('',#29015,#5666);
#4376=LINE('',#29018,#5667);
#4377=LINE('',#29019,#5668);
#4378=LINE('',#29231,#5669);
#4379=LINE('',#29235,#5670);
#4380=LINE('',#29447,#5671);
#4381=LINE('',#29450,#5672);
#4382=LINE('',#29451,#5673);
#4383=LINE('',#29663,#5674);
#4384=LINE('',#29667,#5675);
#4385=LINE('',#29879,#5676);
#4386=LINE('',#29882,#5677);
#4387=LINE('',#29883,#5678);
#4388=LINE('',#30095,#5679);
#4389=LINE('',#30099,#5680);
#4390=LINE('',#30311,#5681);
#4391=LINE('',#30314,#5682);
#4392=LINE('',#30315,#5683);
#4393=LINE('',#30527,#5684);
#4394=LINE('',#30531,#5685);
#4395=LINE('',#30743,#5686);
#4396=LINE('',#30746,#5687);
#4397=LINE('',#30747,#5688);
#4398=LINE('',#30959,#5689);
#4399=LINE('',#30963,#5690);
#4400=LINE('',#31175,#5691);
#4401=LINE('',#31178,#5692);
#4402=LINE('',#31179,#5693);
#4403=LINE('',#31391,#5694);
#4404=LINE('',#31395,#5695);
#4405=LINE('',#31607,#5696);
#4406=LINE('',#31610,#5697);
#4407=LINE('',#31611,#5698);
#4408=LINE('',#31823,#5699);
#4409=LINE('',#31827,#5700);
#4410=LINE('',#32039,#5701);
#4411=LINE('',#32042,#5702);
#4412=LINE('',#32043,#5703);
#4413=LINE('',#32255,#5704);
#4414=LINE('',#32259,#5705);
#4415=LINE('',#32471,#5706);
#4416=LINE('',#32474,#5707);
#4417=LINE('',#32475,#5708);
#4418=LINE('',#32687,#5709);
#4419=LINE('',#32691,#5710);
#4420=LINE('',#32903,#5711);
#4421=LINE('',#32906,#5712);
#4422=LINE('',#32907,#5713);
#4423=LINE('',#33119,#5714);
#4424=LINE('',#33123,#5715);
#4425=LINE('',#33335,#5716);
#4426=LINE('',#33338,#5717);
#4427=LINE('',#33339,#5718);
#4428=LINE('',#33551,#5719);
#4429=LINE('',#33555,#5720);
#4430=LINE('',#33767,#5721);
#4431=LINE('',#33770,#5722);
#4432=LINE('',#33771,#5723);
#4433=LINE('',#33983,#5724);
#4434=LINE('',#33987,#5725);
#4435=LINE('',#34199,#5726);
#4436=LINE('',#34202,#5727);
#4437=LINE('',#34203,#5728);
#4438=LINE('',#34415,#5729);
#5599=VECTOR('',#18698,1.);
#5600=VECTOR('',#18699,1.);
#5601=VECTOR('',#18700,1.);
#5602=VECTOR('',#18701,1.);
#5603=VECTOR('',#18704,1.);
#5604=VECTOR('',#18705,1.);
#5605=VECTOR('',#18706,1.);
#5606=VECTOR('',#18709,1.);
#5607=VECTOR('',#18710,1.);
#5608=VECTOR('',#18711,1.);
#5609=VECTOR('',#18716,1.);
#5610=VECTOR('',#18719,1.);
#5611=VECTOR('',#18722,1.);
#5612=VECTOR('',#18725,1.);
#5613=VECTOR('',#18728,1.);
#5614=VECTOR('',#18731,1.);
#5615=VECTOR('',#18734,1.);
#5616=VECTOR('',#18737,1.);
#5617=VECTOR('',#18740,1.);
#5618=VECTOR('',#18743,1.);
#5619=VECTOR('',#18746,1.);
#5620=VECTOR('',#18749,1.);
#5621=VECTOR('',#18752,1.);
#5622=VECTOR('',#18755,1.);
#5623=VECTOR('',#18758,1.);
#5624=VECTOR('',#18761,1.);
#5625=VECTOR('',#18764,1.);
#5626=VECTOR('',#18767,1.);
#5627=VECTOR('',#18770,1.);
#5628=VECTOR('',#18773,1.);
#5629=VECTOR('',#18784,1.4);
#5630=VECTOR('',#18789,1.);
#5631=VECTOR('',#18790,1.);
#5632=VECTOR('',#18793,1.);
#5633=VECTOR('',#18794,1.);
#5634=VECTOR('',#18795,1.);
#5635=VECTOR('',#18800,1.);
#5636=VECTOR('',#18801,1.);
#5637=VECTOR('',#18804,1.);
#5638=VECTOR('',#18805,1.);
#5639=VECTOR('',#18806,1.);
#5640=VECTOR('',#18811,1.);
#5641=VECTOR('',#18812,1.);
#5642=VECTOR('',#18815,1.);
#5643=VECTOR('',#18816,1.);
#5644=VECTOR('',#18817,1.);
#5645=VECTOR('',#18822,1.);
#5646=VECTOR('',#18823,1.);
#5647=VECTOR('',#18826,1.);
#5648=VECTOR('',#18827,1.);
#5649=VECTOR('',#18828,1.);
#5650=VECTOR('',#18833,1.);
#5651=VECTOR('',#18834,1.);
#5652=VECTOR('',#18837,1.);
#5653=VECTOR('',#18838,1.);
#5654=VECTOR('',#18839,1.);
#5655=VECTOR('',#18844,1.);
#5656=VECTOR('',#18845,1.);
#5657=VECTOR('',#18848,1.);
#5658=VECTOR('',#18849,1.);
#5659=VECTOR('',#18850,1.);
#5660=VECTOR('',#18855,1.);
#5661=VECTOR('',#18856,1.);
#5662=VECTOR('',#18859,1.);
#5663=VECTOR('',#18860,1.);
#5664=VECTOR('',#18861,1.);
#5665=VECTOR('',#18866,1.);
#5666=VECTOR('',#18867,1.);
#5667=VECTOR('',#18870,1.);
#5668=VECTOR('',#18871,1.);
#5669=VECTOR('',#18872,1.);
#5670=VECTOR('',#18877,1.);
#5671=VECTOR('',#18878,1.);
#5672=VECTOR('',#18881,1.);
#5673=VECTOR('',#18882,1.);
#5674=VECTOR('',#18883,1.);
#5675=VECTOR('',#18888,1.);
#5676=VECTOR('',#18889,1.);
#5677=VECTOR('',#18892,1.);
#5678=VECTOR('',#18893,1.);
#5679=VECTOR('',#18894,1.);
#5680=VECTOR('',#18899,1.);
#5681=VECTOR('',#18900,1.);
#5682=VECTOR('',#18903,1.);
#5683=VECTOR('',#18904,1.);
#5684=VECTOR('',#18905,1.);
#5685=VECTOR('',#18910,1.);
#5686=VECTOR('',#18911,1.);
#5687=VECTOR('',#18914,1.);
#5688=VECTOR('',#18915,1.);
#5689=VECTOR('',#18916,1.);
#5690=VECTOR('',#18921,1.);
#5691=VECTOR('',#18922,1.);
#5692=VECTOR('',#18925,1.);
#5693=VECTOR('',#18926,1.);
#5694=VECTOR('',#18927,1.);
#5695=VECTOR('',#18932,1.);
#5696=VECTOR('',#18933,1.);
#5697=VECTOR('',#18936,1.);
#5698=VECTOR('',#18937,1.);
#5699=VECTOR('',#18938,1.);
#5700=VECTOR('',#18943,1.);
#5701=VECTOR('',#18944,1.);
#5702=VECTOR('',#18947,1.);
#5703=VECTOR('',#18948,1.);
#5704=VECTOR('',#18949,1.);
#5705=VECTOR('',#18954,1.);
#5706=VECTOR('',#18955,1.);
#5707=VECTOR('',#18958,1.);
#5708=VECTOR('',#18959,1.);
#5709=VECTOR('',#18960,1.);
#5710=VECTOR('',#18965,1.);
#5711=VECTOR('',#18966,1.);
#5712=VECTOR('',#18969,1.);
#5713=VECTOR('',#18970,1.);
#5714=VECTOR('',#18971,1.);
#5715=VECTOR('',#18976,1.);
#5716=VECTOR('',#18977,1.);
#5717=VECTOR('',#18980,1.);
#5718=VECTOR('',#18981,1.);
#5719=VECTOR('',#18982,1.);
#5720=VECTOR('',#18987,1.);
#5721=VECTOR('',#18988,1.);
#5722=VECTOR('',#18991,1.);
#5723=VECTOR('',#18992,1.);
#5724=VECTOR('',#18993,1.);
#5725=VECTOR('',#18998,1.);
#5726=VECTOR('',#18999,1.);
#5727=VECTOR('',#19002,1.);
#5728=VECTOR('',#19003,1.);
#5729=VECTOR('',#19004,1.);
#6156=CIRCLE('',#15327,1.75);
#6157=CIRCLE('',#15328,1.75);
#6158=CIRCLE('',#15329,1.75);
#6159=CIRCLE('',#15330,1.75);
#6160=CIRCLE('',#15331,1.75);
#6161=CIRCLE('',#15332,1.75);
#6162=CIRCLE('',#15333,1.75);
#6163=CIRCLE('',#15334,1.75);
#6164=CIRCLE('',#15335,1.75);
#6165=CIRCLE('',#15336,1.75);
#6166=CIRCLE('',#15337,1.75);
#6167=CIRCLE('',#15338,1.75);
#6168=CIRCLE('',#15339,1.75);
#6169=CIRCLE('',#15340,1.75);
#6170=CIRCLE('',#15341,1.75);
#6171=CIRCLE('',#15342,1.75);
#6172=CIRCLE('',#15343,1.75);
#6173=CIRCLE('',#15344,1.75);
#6174=CIRCLE('',#15345,1.75);
#6175=CIRCLE('',#15346,1.75);
#6176=CIRCLE('',#15347,0.6);
#6177=CIRCLE('',#15349,0.6);
#6178=CIRCLE('',#15351,1.4);
#6179=CIRCLE('',#15352,1.4);
#6180=CIRCLE('',#15356,1.75);
#6181=CIRCLE('',#15359,1.75);
#6182=CIRCLE('',#15362,1.75);
#6183=CIRCLE('',#15365,1.75);
#6184=CIRCLE('',#15368,1.75);
#6185=CIRCLE('',#15371,1.75);
#6186=CIRCLE('',#15374,1.75);
#6187=CIRCLE('',#15377,1.75);
#6188=CIRCLE('',#15380,1.75);
#6189=CIRCLE('',#15383,1.75);
#6190=CIRCLE('',#15386,1.75);
#6191=CIRCLE('',#15389,1.75);
#6192=CIRCLE('',#15392,1.75);
#6193=CIRCLE('',#15395,1.75);
#6194=CIRCLE('',#15398,1.75);
#6195=CIRCLE('',#15401,1.75);
#6196=CIRCLE('',#15404,1.75);
#6197=CIRCLE('',#15407,1.75);
#6198=CIRCLE('',#15410,1.75);
#6199=CIRCLE('',#15413,1.75);
#7195=VERTEX_POINT('',#22827);
#7196=VERTEX_POINT('',#22828);
#7197=VERTEX_POINT('',#22830);
#7198=VERTEX_POINT('',#22832);
#7199=VERTEX_POINT('',#22836);
#7200=VERTEX_POINT('',#22838);
#7201=VERTEX_POINT('',#22842);
#7202=VERTEX_POINT('',#22844);
#7203=VERTEX_POINT('',#22848);
#7204=VERTEX_POINT('',#22849);
#7205=VERTEX_POINT('',#22851);
#7206=VERTEX_POINT('',#22922);
#7207=VERTEX_POINT('',#22924);
#7208=VERTEX_POINT('',#22995);
#7209=VERTEX_POINT('',#22997);
#7210=VERTEX_POINT('',#23068);
#7211=VERTEX_POINT('',#23070);
#7212=VERTEX_POINT('',#23141);
#7213=VERTEX_POINT('',#23143);
#7214=VERTEX_POINT('',#23214);
#7215=VERTEX_POINT('',#23216);
#7216=VERTEX_POINT('',#23287);
#7217=VERTEX_POINT('',#23289);
#7218=VERTEX_POINT('',#23360);
#7219=VERTEX_POINT('',#23362);
#7220=VERTEX_POINT('',#23433);
#7221=VERTEX_POINT('',#23435);
#7222=VERTEX_POINT('',#23506);
#7223=VERTEX_POINT('',#23508);
#7224=VERTEX_POINT('',#23579);
#7225=VERTEX_POINT('',#23581);
#7226=VERTEX_POINT('',#23652);
#7227=VERTEX_POINT('',#23654);
#7228=VERTEX_POINT('',#23725);
#7229=VERTEX_POINT('',#23727);
#7230=VERTEX_POINT('',#23798);
#7231=VERTEX_POINT('',#23800);
#7232=VERTEX_POINT('',#23871);
#7233=VERTEX_POINT('',#23873);
#7234=VERTEX_POINT('',#23944);
#7235=VERTEX_POINT('',#23946);
#7236=VERTEX_POINT('',#24017);
#7237=VERTEX_POINT('',#24019);
#7238=VERTEX_POINT('',#24090);
#7239=VERTEX_POINT('',#24092);
#7240=VERTEX_POINT('',#24163);
#7241=VERTEX_POINT('',#24165);
#7242=VERTEX_POINT('',#24236);
#7243=VERTEX_POINT('',#24238);
#7244=VERTEX_POINT('',#24309);
#7245=VERTEX_POINT('',#24311);
#7246=VERTEX_POINT('',#24382);
#7247=VERTEX_POINT('',#24384);
#7248=VERTEX_POINT('',#24455);
#7249=VERTEX_POINT('',#24457);
#7250=VERTEX_POINT('',#24528);
#7251=VERTEX_POINT('',#24530);
#7252=VERTEX_POINT('',#24601);
#7253=VERTEX_POINT('',#24603);
#7254=VERTEX_POINT('',#24674);
#7255=VERTEX_POINT('',#24676);
#7256=VERTEX_POINT('',#24747);
#7257=VERTEX_POINT('',#24749);
#7258=VERTEX_POINT('',#24820);
#7259=VERTEX_POINT('',#24822);
#7260=VERTEX_POINT('',#24893);
#7261=VERTEX_POINT('',#24895);
#7262=VERTEX_POINT('',#24966);
#7263=VERTEX_POINT('',#24968);
#7264=VERTEX_POINT('',#25039);
#7265=VERTEX_POINT('',#25041);
#7266=VERTEX_POINT('',#25112);
#7267=VERTEX_POINT('',#25114);
#7268=VERTEX_POINT('',#25185);
#7269=VERTEX_POINT('',#25187);
#7270=VERTEX_POINT('',#25258);
#7271=VERTEX_POINT('',#25260);
#7272=VERTEX_POINT('',#25331);
#7273=VERTEX_POINT('',#25333);
#7274=VERTEX_POINT('',#25404);
#7275=VERTEX_POINT('',#25406);
#7276=VERTEX_POINT('',#25477);
#7277=VERTEX_POINT('',#25479);
#7278=VERTEX_POINT('',#25550);
#7279=VERTEX_POINT('',#25552);
#7280=VERTEX_POINT('',#25623);
#7281=VERTEX_POINT('',#25625);
#7282=VERTEX_POINT('',#25696);
#7283=VERTEX_POINT('',#25772);
#7284=VERTEX_POINT('',#25774);
#7285=VERTEX_POINT('',#25918);
#7286=VERTEX_POINT('',#25920);
#7287=VERTEX_POINT('',#25993);
#7288=VERTEX_POINT('',#26136);
#7289=VERTEX_POINT('',#26209);
#7290=VERTEX_POINT('',#26352);
#7291=VERTEX_POINT('',#26425);
#7292=VERTEX_POINT('',#26568);
#7293=VERTEX_POINT('',#26641);
#7294=VERTEX_POINT('',#26784);
#7295=VERTEX_POINT('',#26857);
#7296=VERTEX_POINT('',#27000);
#7297=VERTEX_POINT('',#27073);
#7298=VERTEX_POINT('',#27216);
#7299=VERTEX_POINT('',#27289);
#7300=VERTEX_POINT('',#27432);
#7301=VERTEX_POINT('',#27505);
#7302=VERTEX_POINT('',#27648);
#7303=VERTEX_POINT('',#27721);
#7304=VERTEX_POINT('',#27864);
#7305=VERTEX_POINT('',#27937);
#7306=VERTEX_POINT('',#28080);
#7307=VERTEX_POINT('',#28153);
#7308=VERTEX_POINT('',#28296);
#7309=VERTEX_POINT('',#28369);
#7310=VERTEX_POINT('',#28512);
#7311=VERTEX_POINT('',#28585);
#7312=VERTEX_POINT('',#28728);
#7313=VERTEX_POINT('',#28801);
#7314=VERTEX_POINT('',#28944);
#7315=VERTEX_POINT('',#29017);
#7316=VERTEX_POINT('',#29160);
#7317=VERTEX_POINT('',#29233);
#7318=VERTEX_POINT('',#29376);
#7319=VERTEX_POINT('',#29449);
#7320=VERTEX_POINT('',#29592);
#7321=VERTEX_POINT('',#29665);
#7322=VERTEX_POINT('',#29808);
#7323=VERTEX_POINT('',#29881);
#7324=VERTEX_POINT('',#30024);
#7325=VERTEX_POINT('',#30097);
#7326=VERTEX_POINT('',#30240);
#7327=VERTEX_POINT('',#30313);
#7328=VERTEX_POINT('',#30456);
#7329=VERTEX_POINT('',#30529);
#7330=VERTEX_POINT('',#30672);
#7331=VERTEX_POINT('',#30745);
#7332=VERTEX_POINT('',#30888);
#7333=VERTEX_POINT('',#30961);
#7334=VERTEX_POINT('',#31104);
#7335=VERTEX_POINT('',#31177);
#7336=VERTEX_POINT('',#31320);
#7337=VERTEX_POINT('',#31393);
#7338=VERTEX_POINT('',#31536);
#7339=VERTEX_POINT('',#31609);
#7340=VERTEX_POINT('',#31752);
#7341=VERTEX_POINT('',#31825);
#7342=VERTEX_POINT('',#31968);
#7343=VERTEX_POINT('',#32041);
#7344=VERTEX_POINT('',#32184);
#7345=VERTEX_POINT('',#32257);
#7346=VERTEX_POINT('',#32400);
#7347=VERTEX_POINT('',#32473);
#7348=VERTEX_POINT('',#32616);
#7349=VERTEX_POINT('',#32689);
#7350=VERTEX_POINT('',#32832);
#7351=VERTEX_POINT('',#32905);
#7352=VERTEX_POINT('',#33048);
#7353=VERTEX_POINT('',#33121);
#7354=VERTEX_POINT('',#33264);
#7355=VERTEX_POINT('',#33337);
#7356=VERTEX_POINT('',#33480);
#7357=VERTEX_POINT('',#33553);
#7358=VERTEX_POINT('',#33696);
#7359=VERTEX_POINT('',#33769);
#7360=VERTEX_POINT('',#33912);
#7361=VERTEX_POINT('',#33985);
#7362=VERTEX_POINT('',#34128);
#7363=VERTEX_POINT('',#34201);
#7364=VERTEX_POINT('',#34344);
#8879=EDGE_CURVE('',#7195,#7196,#4308,.T.);
#8880=EDGE_CURVE('',#7197,#7195,#4309,.T.);
#8881=EDGE_CURVE('',#7198,#7197,#4310,.T.);
#8882=EDGE_CURVE('',#7196,#7198,#4311,.T.);
#8883=EDGE_CURVE('',#7199,#7195,#4312,.T.);
#8884=EDGE_CURVE('',#7199,#7200,#4313,.T.);
#8885=EDGE_CURVE('',#7197,#7200,#4314,.T.);
#8886=EDGE_CURVE('',#7201,#7199,#4315,.T.);
#8887=EDGE_CURVE('',#7202,#7201,#4316,.T.);
#8888=EDGE_CURVE('',#7200,#7202,#4317,.T.);
#8889=EDGE_CURVE('',#7203,#7204,#6156,.T.);
#8890=EDGE_CURVE('',#7204,#7205,#51,.T.);
#8891=EDGE_CURVE('',#7205,#7206,#4318,.T.);
#8892=EDGE_CURVE('',#7206,#7207,#52,.T.);
#8893=EDGE_CURVE('',#7207,#7208,#6157,.T.);
#8894=EDGE_CURVE('',#7208,#7209,#53,.T.);
#8895=EDGE_CURVE('',#7209,#7210,#4319,.T.);
#8896=EDGE_CURVE('',#7210,#7211,#54,.T.);
#8897=EDGE_CURVE('',#7211,#7212,#6158,.T.);
#8898=EDGE_CURVE('',#7212,#7213,#55,.T.);
#8899=EDGE_CURVE('',#7213,#7214,#4320,.T.);
#8900=EDGE_CURVE('',#7214,#7215,#56,.T.);
#8901=EDGE_CURVE('',#7215,#7216,#6159,.T.);
#8902=EDGE_CURVE('',#7216,#7217,#57,.T.);
#8903=EDGE_CURVE('',#7217,#7218,#4321,.T.);
#8904=EDGE_CURVE('',#7218,#7219,#58,.T.);
#8905=EDGE_CURVE('',#7219,#7220,#6160,.T.);
#8906=EDGE_CURVE('',#7220,#7221,#59,.T.);
#8907=EDGE_CURVE('',#7221,#7222,#4322,.T.);
#8908=EDGE_CURVE('',#7222,#7223,#60,.T.);
#8909=EDGE_CURVE('',#7223,#7224,#6161,.T.);
#8910=EDGE_CURVE('',#7224,#7225,#61,.T.);
#8911=EDGE_CURVE('',#7225,#7226,#4323,.T.);
#8912=EDGE_CURVE('',#7226,#7227,#62,.T.);
#8913=EDGE_CURVE('',#7227,#7228,#6162,.T.);
#8914=EDGE_CURVE('',#7228,#7229,#63,.T.);
#8915=EDGE_CURVE('',#7229,#7230,#4324,.T.);
#8916=EDGE_CURVE('',#7230,#7231,#64,.T.);
#8917=EDGE_CURVE('',#7231,#7232,#6163,.T.);
#8918=EDGE_CURVE('',#7232,#7233,#65,.T.);
#8919=EDGE_CURVE('',#7233,#7234,#4325,.T.);
#8920=EDGE_CURVE('',#7234,#7235,#66,.T.);
#8921=EDGE_CURVE('',#7235,#7236,#6164,.T.);
#8922=EDGE_CURVE('',#7236,#7237,#67,.T.);
#8923=EDGE_CURVE('',#7237,#7238,#4326,.T.);
#8924=EDGE_CURVE('',#7238,#7239,#68,.T.);
#8925=EDGE_CURVE('',#7239,#7240,#6165,.T.);
#8926=EDGE_CURVE('',#7240,#7241,#69,.T.);
#8927=EDGE_CURVE('',#7241,#7242,#4327,.T.);
#8928=EDGE_CURVE('',#7242,#7243,#70,.T.);
#8929=EDGE_CURVE('',#7243,#7244,#6166,.T.);
#8930=EDGE_CURVE('',#7244,#7245,#71,.T.);
#8931=EDGE_CURVE('',#7245,#7246,#4328,.T.);
#8932=EDGE_CURVE('',#7246,#7247,#72,.T.);
#8933=EDGE_CURVE('',#7247,#7248,#6167,.T.);
#8934=EDGE_CURVE('',#7248,#7249,#73,.T.);
#8935=EDGE_CURVE('',#7249,#7250,#4329,.T.);
#8936=EDGE_CURVE('',#7250,#7251,#74,.T.);
#8937=EDGE_CURVE('',#7251,#7252,#6168,.T.);
#8938=EDGE_CURVE('',#7252,#7253,#75,.T.);
#8939=EDGE_CURVE('',#7253,#7254,#4330,.T.);
#8940=EDGE_CURVE('',#7254,#7255,#76,.T.);
#8941=EDGE_CURVE('',#7255,#7256,#6169,.T.);
#8942=EDGE_CURVE('',#7256,#7257,#77,.T.);
#8943=EDGE_CURVE('',#7257,#7258,#4331,.T.);
#8944=EDGE_CURVE('',#7258,#7259,#78,.T.);
#8945=EDGE_CURVE('',#7259,#7260,#6170,.T.);
#8946=EDGE_CURVE('',#7260,#7261,#79,.T.);
#8947=EDGE_CURVE('',#7261,#7262,#4332,.T.);
#8948=EDGE_CURVE('',#7262,#7263,#80,.T.);
#8949=EDGE_CURVE('',#7263,#7264,#6171,.T.);
#8950=EDGE_CURVE('',#7264,#7265,#81,.T.);
#8951=EDGE_CURVE('',#7265,#7266,#4333,.T.);
#8952=EDGE_CURVE('',#7266,#7267,#82,.T.);
#8953=EDGE_CURVE('',#7267,#7268,#6172,.T.);
#8954=EDGE_CURVE('',#7268,#7269,#83,.T.);
#8955=EDGE_CURVE('',#7269,#7270,#4334,.T.);
#8956=EDGE_CURVE('',#7270,#7271,#84,.T.);
#8957=EDGE_CURVE('',#7271,#7272,#6173,.T.);
#8958=EDGE_CURVE('',#7272,#7273,#85,.T.);
#8959=EDGE_CURVE('',#7273,#7274,#4335,.T.);
#8960=EDGE_CURVE('',#7274,#7275,#86,.T.);
#8961=EDGE_CURVE('',#7275,#7276,#6174,.T.);
#8962=EDGE_CURVE('',#7276,#7277,#87,.T.);
#8963=EDGE_CURVE('',#7277,#7278,#4336,.T.);
#8964=EDGE_CURVE('',#7278,#7279,#88,.T.);
#8965=EDGE_CURVE('',#7279,#7280,#6175,.T.);
#8966=EDGE_CURVE('',#7280,#7281,#89,.T.);
#8967=EDGE_CURVE('',#7281,#7282,#4337,.T.);
#8968=EDGE_CURVE('',#7282,#7203,#90,.T.);
#8969=EDGE_CURVE('',#7202,#7198,#6176,.T.);
#8970=EDGE_CURVE('',#7196,#7201,#6177,.T.);
#8971=EDGE_CURVE('',#7283,#7283,#6178,.T.);
#8972=EDGE_CURVE('',#7283,#7284,#4338,.T.);
#8973=EDGE_CURVE('',#7284,#7284,#6179,.T.);
#8974=EDGE_CURVE('',#7285,#7280,#4339,.T.);
#8975=EDGE_CURVE('',#7286,#7285,#91,.T.);
#8976=EDGE_CURVE('',#7281,#7286,#4340,.T.);
#8977=EDGE_CURVE('',#7287,#7286,#4341,.T.);
#8978=EDGE_CURVE('',#7282,#7287,#4342,.T.);
#8979=EDGE_CURVE('',#7288,#7287,#92,.T.);
#8980=EDGE_CURVE('',#7203,#7288,#4343,.T.);
#8981=EDGE_CURVE('',#7289,#7288,#6180,.T.);
#8982=EDGE_CURVE('',#7289,#7204,#4344,.T.);
#8983=EDGE_CURVE('',#7290,#7289,#93,.T.);
#8984=EDGE_CURVE('',#7205,#7290,#4345,.T.);
#8985=EDGE_CURVE('',#7291,#7290,#4346,.T.);
#8986=EDGE_CURVE('',#7206,#7291,#4347,.T.);
#8987=EDGE_CURVE('',#7292,#7291,#94,.T.);
#8988=EDGE_CURVE('',#7207,#7292,#4348,.T.);
#8989=EDGE_CURVE('',#7293,#7292,#6181,.T.);
#8990=EDGE_CURVE('',#7293,#7208,#4349,.T.);
#8991=EDGE_CURVE('',#7294,#7293,#95,.T.);
#8992=EDGE_CURVE('',#7209,#7294,#4350,.T.);
#8993=EDGE_CURVE('',#7295,#7294,#4351,.T.);
#8994=EDGE_CURVE('',#7210,#7295,#4352,.T.);
#8995=EDGE_CURVE('',#7296,#7295,#96,.T.);
#8996=EDGE_CURVE('',#7211,#7296,#4353,.T.);
#8997=EDGE_CURVE('',#7297,#7296,#6182,.T.);
#8998=EDGE_CURVE('',#7297,#7212,#4354,.T.);
#8999=EDGE_CURVE('',#7298,#7297,#97,.T.);
#9000=EDGE_CURVE('',#7213,#7298,#4355,.T.);
#9001=EDGE_CURVE('',#7299,#7298,#4356,.T.);
#9002=EDGE_CURVE('',#7214,#7299,#4357,.T.);
#9003=EDGE_CURVE('',#7300,#7299,#98,.T.);
#9004=EDGE_CURVE('',#7215,#7300,#4358,.T.);
#9005=EDGE_CURVE('',#7301,#7300,#6183,.T.);
#9006=EDGE_CURVE('',#7301,#7216,#4359,.T.);
#9007=EDGE_CURVE('',#7302,#7301,#99,.T.);
#9008=EDGE_CURVE('',#7217,#7302,#4360,.T.);
#9009=EDGE_CURVE('',#7303,#7302,#4361,.T.);
#9010=EDGE_CURVE('',#7218,#7303,#4362,.T.);
#9011=EDGE_CURVE('',#7304,#7303,#100,.T.);
#9012=EDGE_CURVE('',#7219,#7304,#4363,.T.);
#9013=EDGE_CURVE('',#7305,#7304,#6184,.T.);
#9014=EDGE_CURVE('',#7305,#7220,#4364,.T.);
#9015=EDGE_CURVE('',#7306,#7305,#101,.T.);
#9016=EDGE_CURVE('',#7221,#7306,#4365,.T.);
#9017=EDGE_CURVE('',#7307,#7306,#4366,.T.);
#9018=EDGE_CURVE('',#7222,#7307,#4367,.T.);
#9019=EDGE_CURVE('',#7308,#7307,#102,.T.);
#9020=EDGE_CURVE('',#7223,#7308,#4368,.T.);
#9021=EDGE_CURVE('',#7309,#7308,#6185,.T.);
#9022=EDGE_CURVE('',#7309,#7224,#4369,.T.);
#9023=EDGE_CURVE('',#7310,#7309,#103,.T.);
#9024=EDGE_CURVE('',#7225,#7310,#4370,.T.);
#9025=EDGE_CURVE('',#7311,#7310,#4371,.T.);
#9026=EDGE_CURVE('',#7226,#7311,#4372,.T.);
#9027=EDGE_CURVE('',#7312,#7311,#104,.T.);
#9028=EDGE_CURVE('',#7227,#7312,#4373,.T.);
#9029=EDGE_CURVE('',#7313,#7312,#6186,.T.);
#9030=EDGE_CURVE('',#7313,#7228,#4374,.T.);
#9031=EDGE_CURVE('',#7314,#7313,#105,.T.);
#9032=EDGE_CURVE('',#7229,#7314,#4375,.T.);
#9033=EDGE_CURVE('',#7315,#7314,#4376,.T.);
#9034=EDGE_CURVE('',#7230,#7315,#4377,.T.);
#9035=EDGE_CURVE('',#7316,#7315,#106,.T.);
#9036=EDGE_CURVE('',#7231,#7316,#4378,.T.);
#9037=EDGE_CURVE('',#7317,#7316,#6187,.T.);
#9038=EDGE_CURVE('',#7317,#7232,#4379,.T.);
#9039=EDGE_CURVE('',#7318,#7317,#107,.T.);
#9040=EDGE_CURVE('',#7233,#7318,#4380,.T.);
#9041=EDGE_CURVE('',#7319,#7318,#4381,.T.);
#9042=EDGE_CURVE('',#7234,#7319,#4382,.T.);
#9043=EDGE_CURVE('',#7320,#7319,#108,.T.);
#9044=EDGE_CURVE('',#7235,#7320,#4383,.T.);
#9045=EDGE_CURVE('',#7321,#7320,#6188,.T.);
#9046=EDGE_CURVE('',#7321,#7236,#4384,.T.);
#9047=EDGE_CURVE('',#7322,#7321,#109,.T.);
#9048=EDGE_CURVE('',#7237,#7322,#4385,.T.);
#9049=EDGE_CURVE('',#7323,#7322,#4386,.T.);
#9050=EDGE_CURVE('',#7238,#7323,#4387,.T.);
#9051=EDGE_CURVE('',#7324,#7323,#110,.T.);
#9052=EDGE_CURVE('',#7239,#7324,#4388,.T.);
#9053=EDGE_CURVE('',#7325,#7324,#6189,.T.);
#9054=EDGE_CURVE('',#7325,#7240,#4389,.T.);
#9055=EDGE_CURVE('',#7326,#7325,#111,.T.);
#9056=EDGE_CURVE('',#7241,#7326,#4390,.T.);
#9057=EDGE_CURVE('',#7327,#7326,#4391,.T.);
#9058=EDGE_CURVE('',#7242,#7327,#4392,.T.);
#9059=EDGE_CURVE('',#7328,#7327,#112,.T.);
#9060=EDGE_CURVE('',#7243,#7328,#4393,.T.);
#9061=EDGE_CURVE('',#7329,#7328,#6190,.T.);
#9062=EDGE_CURVE('',#7329,#7244,#4394,.T.);
#9063=EDGE_CURVE('',#7330,#7329,#113,.T.);
#9064=EDGE_CURVE('',#7245,#7330,#4395,.T.);
#9065=EDGE_CURVE('',#7331,#7330,#4396,.T.);
#9066=EDGE_CURVE('',#7246,#7331,#4397,.T.);
#9067=EDGE_CURVE('',#7332,#7331,#114,.T.);
#9068=EDGE_CURVE('',#7247,#7332,#4398,.T.);
#9069=EDGE_CURVE('',#7333,#7332,#6191,.T.);
#9070=EDGE_CURVE('',#7333,#7248,#4399,.T.);
#9071=EDGE_CURVE('',#7334,#7333,#115,.T.);
#9072=EDGE_CURVE('',#7249,#7334,#4400,.T.);
#9073=EDGE_CURVE('',#7335,#7334,#4401,.T.);
#9074=EDGE_CURVE('',#7250,#7335,#4402,.T.);
#9075=EDGE_CURVE('',#7336,#7335,#116,.T.);
#9076=EDGE_CURVE('',#7251,#7336,#4403,.T.);
#9077=EDGE_CURVE('',#7337,#7336,#6192,.T.);
#9078=EDGE_CURVE('',#7337,#7252,#4404,.T.);
#9079=EDGE_CURVE('',#7338,#7337,#117,.T.);
#9080=EDGE_CURVE('',#7253,#7338,#4405,.T.);
#9081=EDGE_CURVE('',#7339,#7338,#4406,.T.);
#9082=EDGE_CURVE('',#7254,#7339,#4407,.T.);
#9083=EDGE_CURVE('',#7340,#7339,#118,.T.);
#9084=EDGE_CURVE('',#7255,#7340,#4408,.T.);
#9085=EDGE_CURVE('',#7341,#7340,#6193,.T.);
#9086=EDGE_CURVE('',#7341,#7256,#4409,.T.);
#9087=EDGE_CURVE('',#7342,#7341,#119,.T.);
#9088=EDGE_CURVE('',#7257,#7342,#4410,.T.);
#9089=EDGE_CURVE('',#7343,#7342,#4411,.T.);
#9090=EDGE_CURVE('',#7258,#7343,#4412,.T.);
#9091=EDGE_CURVE('',#7344,#7343,#120,.T.);
#9092=EDGE_CURVE('',#7259,#7344,#4413,.T.);
#9093=EDGE_CURVE('',#7345,#7344,#6194,.T.);
#9094=EDGE_CURVE('',#7345,#7260,#4414,.T.);
#9095=EDGE_CURVE('',#7346,#7345,#121,.T.);
#9096=EDGE_CURVE('',#7261,#7346,#4415,.T.);
#9097=EDGE_CURVE('',#7347,#7346,#4416,.T.);
#9098=EDGE_CURVE('',#7262,#7347,#4417,.T.);
#9099=EDGE_CURVE('',#7348,#7347,#122,.T.);
#9100=EDGE_CURVE('',#7263,#7348,#4418,.T.);
#9101=EDGE_CURVE('',#7349,#7348,#6195,.T.);
#9102=EDGE_CURVE('',#7349,#7264,#4419,.T.);
#9103=EDGE_CURVE('',#7350,#7349,#123,.T.);
#9104=EDGE_CURVE('',#7265,#7350,#4420,.T.);
#9105=EDGE_CURVE('',#7351,#7350,#4421,.T.);
#9106=EDGE_CURVE('',#7266,#7351,#4422,.T.);
#9107=EDGE_CURVE('',#7352,#7351,#124,.T.);
#9108=EDGE_CURVE('',#7267,#7352,#4423,.T.);
#9109=EDGE_CURVE('',#7353,#7352,#6196,.T.);
#9110=EDGE_CURVE('',#7353,#7268,#4424,.T.);
#9111=EDGE_CURVE('',#7354,#7353,#125,.T.);
#9112=EDGE_CURVE('',#7269,#7354,#4425,.T.);
#9113=EDGE_CURVE('',#7355,#7354,#4426,.T.);
#9114=EDGE_CURVE('',#7270,#7355,#4427,.T.);
#9115=EDGE_CURVE('',#7356,#7355,#126,.T.);
#9116=EDGE_CURVE('',#7271,#7356,#4428,.T.);
#9117=EDGE_CURVE('',#7357,#7356,#6197,.T.);
#9118=EDGE_CURVE('',#7357,#7272,#4429,.T.);
#9119=EDGE_CURVE('',#7358,#7357,#127,.T.);
#9120=EDGE_CURVE('',#7273,#7358,#4430,.T.);
#9121=EDGE_CURVE('',#7359,#7358,#4431,.T.);
#9122=EDGE_CURVE('',#7274,#7359,#4432,.T.);
#9123=EDGE_CURVE('',#7360,#7359,#128,.T.);
#9124=EDGE_CURVE('',#7275,#7360,#4433,.T.);
#9125=EDGE_CURVE('',#7361,#7360,#6198,.T.);
#9126=EDGE_CURVE('',#7361,#7276,#4434,.T.);
#9127=EDGE_CURVE('',#7362,#7361,#129,.T.);
#9128=EDGE_CURVE('',#7277,#7362,#4435,.T.);
#9129=EDGE_CURVE('',#7363,#7362,#4436,.T.);
#9130=EDGE_CURVE('',#7278,#7363,#4437,.T.);
#9131=EDGE_CURVE('',#7364,#7363,#130,.T.);
#9132=EDGE_CURVE('',#7279,#7364,#4438,.T.);
#9133=EDGE_CURVE('',#7285,#7364,#6199,.T.);
#12134=ORIENTED_EDGE('',*,*,#8879,.F.);
#12135=ORIENTED_EDGE('',*,*,#8880,.F.);
#12136=ORIENTED_EDGE('',*,*,#8881,.F.);
#12137=ORIENTED_EDGE('',*,*,#8882,.F.);
#12138=ORIENTED_EDGE('',*,*,#8883,.F.);
#12139=ORIENTED_EDGE('',*,*,#8884,.T.);
#12140=ORIENTED_EDGE('',*,*,#8885,.F.);
#12141=ORIENTED_EDGE('',*,*,#8880,.T.);
#12142=ORIENTED_EDGE('',*,*,#8886,.F.);
#12143=ORIENTED_EDGE('',*,*,#8887,.F.);
#12144=ORIENTED_EDGE('',*,*,#8888,.F.);
#12145=ORIENTED_EDGE('',*,*,#8884,.F.);
#12146=ORIENTED_EDGE('',*,*,#8889,.T.);
#12147=ORIENTED_EDGE('',*,*,#8890,.T.);
#12148=ORIENTED_EDGE('',*,*,#8891,.T.);
#12149=ORIENTED_EDGE('',*,*,#8892,.T.);
#12150=ORIENTED_EDGE('',*,*,#8893,.T.);
#12151=ORIENTED_EDGE('',*,*,#8894,.T.);
#12152=ORIENTED_EDGE('',*,*,#8895,.T.);
#12153=ORIENTED_EDGE('',*,*,#8896,.T.);
#12154=ORIENTED_EDGE('',*,*,#8897,.T.);
#12155=ORIENTED_EDGE('',*,*,#8898,.T.);
#12156=ORIENTED_EDGE('',*,*,#8899,.T.);
#12157=ORIENTED_EDGE('',*,*,#8900,.T.);
#12158=ORIENTED_EDGE('',*,*,#8901,.T.);
#12159=ORIENTED_EDGE('',*,*,#8902,.T.);
#12160=ORIENTED_EDGE('',*,*,#8903,.T.);
#12161=ORIENTED_EDGE('',*,*,#8904,.T.);
#12162=ORIENTED_EDGE('',*,*,#8905,.T.);
#12163=ORIENTED_EDGE('',*,*,#8906,.T.);
#12164=ORIENTED_EDGE('',*,*,#8907,.T.);
#12165=ORIENTED_EDGE('',*,*,#8908,.T.);
#12166=ORIENTED_EDGE('',*,*,#8909,.T.);
#12167=ORIENTED_EDGE('',*,*,#8910,.T.);
#12168=ORIENTED_EDGE('',*,*,#8911,.T.);
#12169=ORIENTED_EDGE('',*,*,#8912,.T.);
#12170=ORIENTED_EDGE('',*,*,#8913,.T.);
#12171=ORIENTED_EDGE('',*,*,#8914,.T.);
#12172=ORIENTED_EDGE('',*,*,#8915,.T.);
#12173=ORIENTED_EDGE('',*,*,#8916,.T.);
#12174=ORIENTED_EDGE('',*,*,#8917,.T.);
#12175=ORIENTED_EDGE('',*,*,#8918,.T.);
#12176=ORIENTED_EDGE('',*,*,#8919,.T.);
#12177=ORIENTED_EDGE('',*,*,#8920,.T.);
#12178=ORIENTED_EDGE('',*,*,#8921,.T.);
#12179=ORIENTED_EDGE('',*,*,#8922,.T.);
#12180=ORIENTED_EDGE('',*,*,#8923,.T.);
#12181=ORIENTED_EDGE('',*,*,#8924,.T.);
#12182=ORIENTED_EDGE('',*,*,#8925,.T.);
#12183=ORIENTED_EDGE('',*,*,#8926,.T.);
#12184=ORIENTED_EDGE('',*,*,#8927,.T.);
#12185=ORIENTED_EDGE('',*,*,#8928,.T.);
#12186=ORIENTED_EDGE('',*,*,#8929,.T.);
#12187=ORIENTED_EDGE('',*,*,#8930,.T.);
#12188=ORIENTED_EDGE('',*,*,#8931,.T.);
#12189=ORIENTED_EDGE('',*,*,#8932,.T.);
#12190=ORIENTED_EDGE('',*,*,#8933,.T.);
#12191=ORIENTED_EDGE('',*,*,#8934,.T.);
#12192=ORIENTED_EDGE('',*,*,#8935,.T.);
#12193=ORIENTED_EDGE('',*,*,#8936,.T.);
#12194=ORIENTED_EDGE('',*,*,#8937,.T.);
#12195=ORIENTED_EDGE('',*,*,#8938,.T.);
#12196=ORIENTED_EDGE('',*,*,#8939,.T.);
#12197=ORIENTED_EDGE('',*,*,#8940,.T.);
#12198=ORIENTED_EDGE('',*,*,#8941,.T.);
#12199=ORIENTED_EDGE('',*,*,#8942,.T.);
#12200=ORIENTED_EDGE('',*,*,#8943,.T.);
#12201=ORIENTED_EDGE('',*,*,#8944,.T.);
#12202=ORIENTED_EDGE('',*,*,#8945,.T.);
#12203=ORIENTED_EDGE('',*,*,#8946,.T.);
#12204=ORIENTED_EDGE('',*,*,#8947,.T.);
#12205=ORIENTED_EDGE('',*,*,#8948,.T.);
#12206=ORIENTED_EDGE('',*,*,#8949,.T.);
#12207=ORIENTED_EDGE('',*,*,#8950,.T.);
#12208=ORIENTED_EDGE('',*,*,#8951,.T.);
#12209=ORIENTED_EDGE('',*,*,#8952,.T.);
#12210=ORIENTED_EDGE('',*,*,#8953,.T.);
#12211=ORIENTED_EDGE('',*,*,#8954,.T.);
#12212=ORIENTED_EDGE('',*,*,#8955,.T.);
#12213=ORIENTED_EDGE('',*,*,#8956,.T.);
#12214=ORIENTED_EDGE('',*,*,#8957,.T.);
#12215=ORIENTED_EDGE('',*,*,#8958,.T.);
#12216=ORIENTED_EDGE('',*,*,#8959,.T.);
#12217=ORIENTED_EDGE('',*,*,#8960,.T.);
#12218=ORIENTED_EDGE('',*,*,#8961,.T.);
#12219=ORIENTED_EDGE('',*,*,#8962,.T.);
#12220=ORIENTED_EDGE('',*,*,#8963,.T.);
#12221=ORIENTED_EDGE('',*,*,#8964,.T.);
#12222=ORIENTED_EDGE('',*,*,#8965,.T.);
#12223=ORIENTED_EDGE('',*,*,#8966,.T.);
#12224=ORIENTED_EDGE('',*,*,#8967,.T.);
#12225=ORIENTED_EDGE('',*,*,#8968,.T.);
#12226=ORIENTED_EDGE('',*,*,#8881,.T.);
#12227=ORIENTED_EDGE('',*,*,#8885,.T.);
#12228=ORIENTED_EDGE('',*,*,#8888,.T.);
#12229=ORIENTED_EDGE('',*,*,#8969,.T.);
#12230=ORIENTED_EDGE('',*,*,#8882,.T.);
#12231=ORIENTED_EDGE('',*,*,#8969,.F.);
#12232=ORIENTED_EDGE('',*,*,#8887,.T.);
#12233=ORIENTED_EDGE('',*,*,#8970,.F.);
#12234=ORIENTED_EDGE('',*,*,#8971,.F.);
#12235=ORIENTED_EDGE('',*,*,#8972,.T.);
#12236=ORIENTED_EDGE('',*,*,#8973,.F.);
#12237=ORIENTED_EDGE('',*,*,#8972,.F.);
#12238=ORIENTED_EDGE('',*,*,#8971,.T.);
#12239=ORIENTED_EDGE('',*,*,#8879,.T.);
#12240=ORIENTED_EDGE('',*,*,#8970,.T.);
#12241=ORIENTED_EDGE('',*,*,#8886,.T.);
#12242=ORIENTED_EDGE('',*,*,#8883,.T.);
#12243=ORIENTED_EDGE('',*,*,#8974,.F.);
#12244=ORIENTED_EDGE('',*,*,#8975,.F.);
#12245=ORIENTED_EDGE('',*,*,#8976,.F.);
#12246=ORIENTED_EDGE('',*,*,#8966,.F.);
#12247=ORIENTED_EDGE('',*,*,#8976,.T.);
#12248=ORIENTED_EDGE('',*,*,#8977,.F.);
#12249=ORIENTED_EDGE('',*,*,#8978,.F.);
#12250=ORIENTED_EDGE('',*,*,#8967,.F.);
#12251=ORIENTED_EDGE('',*,*,#8978,.T.);
#12252=ORIENTED_EDGE('',*,*,#8979,.F.);
#12253=ORIENTED_EDGE('',*,*,#8980,.F.);
#12254=ORIENTED_EDGE('',*,*,#8968,.F.);
#12255=ORIENTED_EDGE('',*,*,#8980,.T.);
#12256=ORIENTED_EDGE('',*,*,#8981,.F.);
#12257=ORIENTED_EDGE('',*,*,#8982,.T.);
#12258=ORIENTED_EDGE('',*,*,#8889,.F.);
#12259=ORIENTED_EDGE('',*,*,#8982,.F.);
#12260=ORIENTED_EDGE('',*,*,#8983,.F.);
#12261=ORIENTED_EDGE('',*,*,#8984,.F.);
#12262=ORIENTED_EDGE('',*,*,#8890,.F.);
#12263=ORIENTED_EDGE('',*,*,#8984,.T.);
#12264=ORIENTED_EDGE('',*,*,#8985,.F.);
#12265=ORIENTED_EDGE('',*,*,#8986,.F.);
#12266=ORIENTED_EDGE('',*,*,#8891,.F.);
#12267=ORIENTED_EDGE('',*,*,#8986,.T.);
#12268=ORIENTED_EDGE('',*,*,#8987,.F.);
#12269=ORIENTED_EDGE('',*,*,#8988,.F.);
#12270=ORIENTED_EDGE('',*,*,#8892,.F.);
#12271=ORIENTED_EDGE('',*,*,#8988,.T.);
#12272=ORIENTED_EDGE('',*,*,#8989,.F.);
#12273=ORIENTED_EDGE('',*,*,#8990,.T.);
#12274=ORIENTED_EDGE('',*,*,#8893,.F.);
#12275=ORIENTED_EDGE('',*,*,#8990,.F.);
#12276=ORIENTED_EDGE('',*,*,#8991,.F.);
#12277=ORIENTED_EDGE('',*,*,#8992,.F.);
#12278=ORIENTED_EDGE('',*,*,#8894,.F.);
#12279=ORIENTED_EDGE('',*,*,#8992,.T.);
#12280=ORIENTED_EDGE('',*,*,#8993,.F.);
#12281=ORIENTED_EDGE('',*,*,#8994,.F.);
#12282=ORIENTED_EDGE('',*,*,#8895,.F.);
#12283=ORIENTED_EDGE('',*,*,#8994,.T.);
#12284=ORIENTED_EDGE('',*,*,#8995,.F.);
#12285=ORIENTED_EDGE('',*,*,#8996,.F.);
#12286=ORIENTED_EDGE('',*,*,#8896,.F.);
#12287=ORIENTED_EDGE('',*,*,#8996,.T.);
#12288=ORIENTED_EDGE('',*,*,#8997,.F.);
#12289=ORIENTED_EDGE('',*,*,#8998,.T.);
#12290=ORIENTED_EDGE('',*,*,#8897,.F.);
#12291=ORIENTED_EDGE('',*,*,#8998,.F.);
#12292=ORIENTED_EDGE('',*,*,#8999,.F.);
#12293=ORIENTED_EDGE('',*,*,#9000,.F.);
#12294=ORIENTED_EDGE('',*,*,#8898,.F.);
#12295=ORIENTED_EDGE('',*,*,#9000,.T.);
#12296=ORIENTED_EDGE('',*,*,#9001,.F.);
#12297=ORIENTED_EDGE('',*,*,#9002,.F.);
#12298=ORIENTED_EDGE('',*,*,#8899,.F.);
#12299=ORIENTED_EDGE('',*,*,#9002,.T.);
#12300=ORIENTED_EDGE('',*,*,#9003,.F.);
#12301=ORIENTED_EDGE('',*,*,#9004,.F.);
#12302=ORIENTED_EDGE('',*,*,#8900,.F.);
#12303=ORIENTED_EDGE('',*,*,#9004,.T.);
#12304=ORIENTED_EDGE('',*,*,#9005,.F.);
#12305=ORIENTED_EDGE('',*,*,#9006,.T.);
#12306=ORIENTED_EDGE('',*,*,#8901,.F.);
#12307=ORIENTED_EDGE('',*,*,#9006,.F.);
#12308=ORIENTED_EDGE('',*,*,#9007,.F.);
#12309=ORIENTED_EDGE('',*,*,#9008,.F.);
#12310=ORIENTED_EDGE('',*,*,#8902,.F.);
#12311=ORIENTED_EDGE('',*,*,#9008,.T.);
#12312=ORIENTED_EDGE('',*,*,#9009,.F.);
#12313=ORIENTED_EDGE('',*,*,#9010,.F.);
#12314=ORIENTED_EDGE('',*,*,#8903,.F.);
#12315=ORIENTED_EDGE('',*,*,#9010,.T.);
#12316=ORIENTED_EDGE('',*,*,#9011,.F.);
#12317=ORIENTED_EDGE('',*,*,#9012,.F.);
#12318=ORIENTED_EDGE('',*,*,#8904,.F.);
#12319=ORIENTED_EDGE('',*,*,#9012,.T.);
#12320=ORIENTED_EDGE('',*,*,#9013,.F.);
#12321=ORIENTED_EDGE('',*,*,#9014,.T.);
#12322=ORIENTED_EDGE('',*,*,#8905,.F.);
#12323=ORIENTED_EDGE('',*,*,#9014,.F.);
#12324=ORIENTED_EDGE('',*,*,#9015,.F.);
#12325=ORIENTED_EDGE('',*,*,#9016,.F.);
#12326=ORIENTED_EDGE('',*,*,#8906,.F.);
#12327=ORIENTED_EDGE('',*,*,#9016,.T.);
#12328=ORIENTED_EDGE('',*,*,#9017,.F.);
#12329=ORIENTED_EDGE('',*,*,#9018,.F.);
#12330=ORIENTED_EDGE('',*,*,#8907,.F.);
#12331=ORIENTED_EDGE('',*,*,#9018,.T.);
#12332=ORIENTED_EDGE('',*,*,#9019,.F.);
#12333=ORIENTED_EDGE('',*,*,#9020,.F.);
#12334=ORIENTED_EDGE('',*,*,#8908,.F.);
#12335=ORIENTED_EDGE('',*,*,#9020,.T.);
#12336=ORIENTED_EDGE('',*,*,#9021,.F.);
#12337=ORIENTED_EDGE('',*,*,#9022,.T.);
#12338=ORIENTED_EDGE('',*,*,#8909,.F.);
#12339=ORIENTED_EDGE('',*,*,#9022,.F.);
#12340=ORIENTED_EDGE('',*,*,#9023,.F.);
#12341=ORIENTED_EDGE('',*,*,#9024,.F.);
#12342=ORIENTED_EDGE('',*,*,#8910,.F.);
#12343=ORIENTED_EDGE('',*,*,#9024,.T.);
#12344=ORIENTED_EDGE('',*,*,#9025,.F.);
#12345=ORIENTED_EDGE('',*,*,#9026,.F.);
#12346=ORIENTED_EDGE('',*,*,#8911,.F.);
#12347=ORIENTED_EDGE('',*,*,#9026,.T.);
#12348=ORIENTED_EDGE('',*,*,#9027,.F.);
#12349=ORIENTED_EDGE('',*,*,#9028,.F.);
#12350=ORIENTED_EDGE('',*,*,#8912,.F.);
#12351=ORIENTED_EDGE('',*,*,#9028,.T.);
#12352=ORIENTED_EDGE('',*,*,#9029,.F.);
#12353=ORIENTED_EDGE('',*,*,#9030,.T.);
#12354=ORIENTED_EDGE('',*,*,#8913,.F.);
#12355=ORIENTED_EDGE('',*,*,#9030,.F.);
#12356=ORIENTED_EDGE('',*,*,#9031,.F.);
#12357=ORIENTED_EDGE('',*,*,#9032,.F.);
#12358=ORIENTED_EDGE('',*,*,#8914,.F.);
#12359=ORIENTED_EDGE('',*,*,#9032,.T.);
#12360=ORIENTED_EDGE('',*,*,#9033,.F.);
#12361=ORIENTED_EDGE('',*,*,#9034,.F.);
#12362=ORIENTED_EDGE('',*,*,#8915,.F.);
#12363=ORIENTED_EDGE('',*,*,#9034,.T.);
#12364=ORIENTED_EDGE('',*,*,#9035,.F.);
#12365=ORIENTED_EDGE('',*,*,#9036,.F.);
#12366=ORIENTED_EDGE('',*,*,#8916,.F.);
#12367=ORIENTED_EDGE('',*,*,#9036,.T.);
#12368=ORIENTED_EDGE('',*,*,#9037,.F.);
#12369=ORIENTED_EDGE('',*,*,#9038,.T.);
#12370=ORIENTED_EDGE('',*,*,#8917,.F.);
#12371=ORIENTED_EDGE('',*,*,#9038,.F.);
#12372=ORIENTED_EDGE('',*,*,#9039,.F.);
#12373=ORIENTED_EDGE('',*,*,#9040,.F.);
#12374=ORIENTED_EDGE('',*,*,#8918,.F.);
#12375=ORIENTED_EDGE('',*,*,#9040,.T.);
#12376=ORIENTED_EDGE('',*,*,#9041,.F.);
#12377=ORIENTED_EDGE('',*,*,#9042,.F.);
#12378=ORIENTED_EDGE('',*,*,#8919,.F.);
#12379=ORIENTED_EDGE('',*,*,#9042,.T.);
#12380=ORIENTED_EDGE('',*,*,#9043,.F.);
#12381=ORIENTED_EDGE('',*,*,#9044,.F.);
#12382=ORIENTED_EDGE('',*,*,#8920,.F.);
#12383=ORIENTED_EDGE('',*,*,#9044,.T.);
#12384=ORIENTED_EDGE('',*,*,#9045,.F.);
#12385=ORIENTED_EDGE('',*,*,#9046,.T.);
#12386=ORIENTED_EDGE('',*,*,#8921,.F.);
#12387=ORIENTED_EDGE('',*,*,#9046,.F.);
#12388=ORIENTED_EDGE('',*,*,#9047,.F.);
#12389=ORIENTED_EDGE('',*,*,#9048,.F.);
#12390=ORIENTED_EDGE('',*,*,#8922,.F.);
#12391=ORIENTED_EDGE('',*,*,#9048,.T.);
#12392=ORIENTED_EDGE('',*,*,#9049,.F.);
#12393=ORIENTED_EDGE('',*,*,#9050,.F.);
#12394=ORIENTED_EDGE('',*,*,#8923,.F.);
#12395=ORIENTED_EDGE('',*,*,#9050,.T.);
#12396=ORIENTED_EDGE('',*,*,#9051,.F.);
#12397=ORIENTED_EDGE('',*,*,#9052,.F.);
#12398=ORIENTED_EDGE('',*,*,#8924,.F.);
#12399=ORIENTED_EDGE('',*,*,#9052,.T.);
#12400=ORIENTED_EDGE('',*,*,#9053,.F.);
#12401=ORIENTED_EDGE('',*,*,#9054,.T.);
#12402=ORIENTED_EDGE('',*,*,#8925,.F.);
#12403=ORIENTED_EDGE('',*,*,#9054,.F.);
#12404=ORIENTED_EDGE('',*,*,#9055,.F.);
#12405=ORIENTED_EDGE('',*,*,#9056,.F.);
#12406=ORIENTED_EDGE('',*,*,#8926,.F.);
#12407=ORIENTED_EDGE('',*,*,#9056,.T.);
#12408=ORIENTED_EDGE('',*,*,#9057,.F.);
#12409=ORIENTED_EDGE('',*,*,#9058,.F.);
#12410=ORIENTED_EDGE('',*,*,#8927,.F.);
#12411=ORIENTED_EDGE('',*,*,#9058,.T.);
#12412=ORIENTED_EDGE('',*,*,#9059,.F.);
#12413=ORIENTED_EDGE('',*,*,#9060,.F.);
#12414=ORIENTED_EDGE('',*,*,#8928,.F.);
#12415=ORIENTED_EDGE('',*,*,#9060,.T.);
#12416=ORIENTED_EDGE('',*,*,#9061,.F.);
#12417=ORIENTED_EDGE('',*,*,#9062,.T.);
#12418=ORIENTED_EDGE('',*,*,#8929,.F.);
#12419=ORIENTED_EDGE('',*,*,#9062,.F.);
#12420=ORIENTED_EDGE('',*,*,#9063,.F.);
#12421=ORIENTED_EDGE('',*,*,#9064,.F.);
#12422=ORIENTED_EDGE('',*,*,#8930,.F.);
#12423=ORIENTED_EDGE('',*,*,#9064,.T.);
#12424=ORIENTED_EDGE('',*,*,#9065,.F.);
#12425=ORIENTED_EDGE('',*,*,#9066,.F.);
#12426=ORIENTED_EDGE('',*,*,#8931,.F.);
#12427=ORIENTED_EDGE('',*,*,#9066,.T.);
#12428=ORIENTED_EDGE('',*,*,#9067,.F.);
#12429=ORIENTED_EDGE('',*,*,#9068,.F.);
#12430=ORIENTED_EDGE('',*,*,#8932,.F.);
#12431=ORIENTED_EDGE('',*,*,#9068,.T.);
#12432=ORIENTED_EDGE('',*,*,#9069,.F.);
#12433=ORIENTED_EDGE('',*,*,#9070,.T.);
#12434=ORIENTED_EDGE('',*,*,#8933,.F.);
#12435=ORIENTED_EDGE('',*,*,#9070,.F.);
#12436=ORIENTED_EDGE('',*,*,#9071,.F.);
#12437=ORIENTED_EDGE('',*,*,#9072,.F.);
#12438=ORIENTED_EDGE('',*,*,#8934,.F.);
#12439=ORIENTED_EDGE('',*,*,#9072,.T.);
#12440=ORIENTED_EDGE('',*,*,#9073,.F.);
#12441=ORIENTED_EDGE('',*,*,#9074,.F.);
#12442=ORIENTED_EDGE('',*,*,#8935,.F.);
#12443=ORIENTED_EDGE('',*,*,#9074,.T.);
#12444=ORIENTED_EDGE('',*,*,#9075,.F.);
#12445=ORIENTED_EDGE('',*,*,#9076,.F.);
#12446=ORIENTED_EDGE('',*,*,#8936,.F.);
#12447=ORIENTED_EDGE('',*,*,#9076,.T.);
#12448=ORIENTED_EDGE('',*,*,#9077,.F.);
#12449=ORIENTED_EDGE('',*,*,#9078,.T.);
#12450=ORIENTED_EDGE('',*,*,#8937,.F.);
#12451=ORIENTED_EDGE('',*,*,#9078,.F.);
#12452=ORIENTED_EDGE('',*,*,#9079,.F.);
#12453=ORIENTED_EDGE('',*,*,#9080,.F.);
#12454=ORIENTED_EDGE('',*,*,#8938,.F.);
#12455=ORIENTED_EDGE('',*,*,#9080,.T.);
#12456=ORIENTED_EDGE('',*,*,#9081,.F.);
#12457=ORIENTED_EDGE('',*,*,#9082,.F.);
#12458=ORIENTED_EDGE('',*,*,#8939,.F.);
#12459=ORIENTED_EDGE('',*,*,#9082,.T.);
#12460=ORIENTED_EDGE('',*,*,#9083,.F.);
#12461=ORIENTED_EDGE('',*,*,#9084,.F.);
#12462=ORIENTED_EDGE('',*,*,#8940,.F.);
#12463=ORIENTED_EDGE('',*,*,#9084,.T.);
#12464=ORIENTED_EDGE('',*,*,#9085,.F.);
#12465=ORIENTED_EDGE('',*,*,#9086,.T.);
#12466=ORIENTED_EDGE('',*,*,#8941,.F.);
#12467=ORIENTED_EDGE('',*,*,#9086,.F.);
#12468=ORIENTED_EDGE('',*,*,#9087,.F.);
#12469=ORIENTED_EDGE('',*,*,#9088,.F.);
#12470=ORIENTED_EDGE('',*,*,#8942,.F.);
#12471=ORIENTED_EDGE('',*,*,#9088,.T.);
#12472=ORIENTED_EDGE('',*,*,#9089,.F.);
#12473=ORIENTED_EDGE('',*,*,#9090,.F.);
#12474=ORIENTED_EDGE('',*,*,#8943,.F.);
#12475=ORIENTED_EDGE('',*,*,#9090,.T.);
#12476=ORIENTED_EDGE('',*,*,#9091,.F.);
#12477=ORIENTED_EDGE('',*,*,#9092,.F.);
#12478=ORIENTED_EDGE('',*,*,#8944,.F.);
#12479=ORIENTED_EDGE('',*,*,#9092,.T.);
#12480=ORIENTED_EDGE('',*,*,#9093,.F.);
#12481=ORIENTED_EDGE('',*,*,#9094,.T.);
#12482=ORIENTED_EDGE('',*,*,#8945,.F.);
#12483=ORIENTED_EDGE('',*,*,#9094,.F.);
#12484=ORIENTED_EDGE('',*,*,#9095,.F.);
#12485=ORIENTED_EDGE('',*,*,#9096,.F.);
#12486=ORIENTED_EDGE('',*,*,#8946,.F.);
#12487=ORIENTED_EDGE('',*,*,#9096,.T.);
#12488=ORIENTED_EDGE('',*,*,#9097,.F.);
#12489=ORIENTED_EDGE('',*,*,#9098,.F.);
#12490=ORIENTED_EDGE('',*,*,#8947,.F.);
#12491=ORIENTED_EDGE('',*,*,#9098,.T.);
#12492=ORIENTED_EDGE('',*,*,#9099,.F.);
#12493=ORIENTED_EDGE('',*,*,#9100,.F.);
#12494=ORIENTED_EDGE('',*,*,#8948,.F.);
#12495=ORIENTED_EDGE('',*,*,#9100,.T.);
#12496=ORIENTED_EDGE('',*,*,#9101,.F.);
#12497=ORIENTED_EDGE('',*,*,#9102,.T.);
#12498=ORIENTED_EDGE('',*,*,#8949,.F.);
#12499=ORIENTED_EDGE('',*,*,#9102,.F.);
#12500=ORIENTED_EDGE('',*,*,#9103,.F.);
#12501=ORIENTED_EDGE('',*,*,#9104,.F.);
#12502=ORIENTED_EDGE('',*,*,#8950,.F.);
#12503=ORIENTED_EDGE('',*,*,#9104,.T.);
#12504=ORIENTED_EDGE('',*,*,#9105,.F.);
#12505=ORIENTED_EDGE('',*,*,#9106,.F.);
#12506=ORIENTED_EDGE('',*,*,#8951,.F.);
#12507=ORIENTED_EDGE('',*,*,#9106,.T.);
#12508=ORIENTED_EDGE('',*,*,#9107,.F.);
#12509=ORIENTED_EDGE('',*,*,#9108,.F.);
#12510=ORIENTED_EDGE('',*,*,#8952,.F.);
#12511=ORIENTED_EDGE('',*,*,#9108,.T.);
#12512=ORIENTED_EDGE('',*,*,#9109,.F.);
#12513=ORIENTED_EDGE('',*,*,#9110,.T.);
#12514=ORIENTED_EDGE('',*,*,#8953,.F.);
#12515=ORIENTED_EDGE('',*,*,#9110,.F.);
#12516=ORIENTED_EDGE('',*,*,#9111,.F.);
#12517=ORIENTED_EDGE('',*,*,#9112,.F.);
#12518=ORIENTED_EDGE('',*,*,#8954,.F.);
#12519=ORIENTED_EDGE('',*,*,#9112,.T.);
#12520=ORIENTED_EDGE('',*,*,#9113,.F.);
#12521=ORIENTED_EDGE('',*,*,#9114,.F.);
#12522=ORIENTED_EDGE('',*,*,#8955,.F.);
#12523=ORIENTED_EDGE('',*,*,#9114,.T.);
#12524=ORIENTED_EDGE('',*,*,#9115,.F.);
#12525=ORIENTED_EDGE('',*,*,#9116,.F.);
#12526=ORIENTED_EDGE('',*,*,#8956,.F.);
#12527=ORIENTED_EDGE('',*,*,#9116,.T.);
#12528=ORIENTED_EDGE('',*,*,#9117,.F.);
#12529=ORIENTED_EDGE('',*,*,#9118,.T.);
#12530=ORIENTED_EDGE('',*,*,#8957,.F.);
#12531=ORIENTED_EDGE('',*,*,#9118,.F.);
#12532=ORIENTED_EDGE('',*,*,#9119,.F.);
#12533=ORIENTED_EDGE('',*,*,#9120,.F.);
#12534=ORIENTED_EDGE('',*,*,#8958,.F.);
#12535=ORIENTED_EDGE('',*,*,#9120,.T.);
#12536=ORIENTED_EDGE('',*,*,#9121,.F.);
#12537=ORIENTED_EDGE('',*,*,#9122,.F.);
#12538=ORIENTED_EDGE('',*,*,#8959,.F.);
#12539=ORIENTED_EDGE('',*,*,#9122,.T.);
#12540=ORIENTED_EDGE('',*,*,#9123,.F.);
#12541=ORIENTED_EDGE('',*,*,#9124,.F.);
#12542=ORIENTED_EDGE('',*,*,#8960,.F.);
#12543=ORIENTED_EDGE('',*,*,#9124,.T.);
#12544=ORIENTED_EDGE('',*,*,#9125,.F.);
#12545=ORIENTED_EDGE('',*,*,#9126,.T.);
#12546=ORIENTED_EDGE('',*,*,#8961,.F.);
#12547=ORIENTED_EDGE('',*,*,#9126,.F.);
#12548=ORIENTED_EDGE('',*,*,#9127,.F.);
#12549=ORIENTED_EDGE('',*,*,#9128,.F.);
#12550=ORIENTED_EDGE('',*,*,#8962,.F.);
#12551=ORIENTED_EDGE('',*,*,#9128,.T.);
#12552=ORIENTED_EDGE('',*,*,#9129,.F.);
#12553=ORIENTED_EDGE('',*,*,#9130,.F.);
#12554=ORIENTED_EDGE('',*,*,#8963,.F.);
#12555=ORIENTED_EDGE('',*,*,#9130,.T.);
#12556=ORIENTED_EDGE('',*,*,#9131,.F.);
#12557=ORIENTED_EDGE('',*,*,#9132,.F.);
#12558=ORIENTED_EDGE('',*,*,#8964,.F.);
#12559=ORIENTED_EDGE('',*,*,#9133,.T.);
#12560=ORIENTED_EDGE('',*,*,#9131,.T.);
#12561=ORIENTED_EDGE('',*,*,#9129,.T.);
#12562=ORIENTED_EDGE('',*,*,#9127,.T.);
#12563=ORIENTED_EDGE('',*,*,#9125,.T.);
#12564=ORIENTED_EDGE('',*,*,#9123,.T.);
#12565=ORIENTED_EDGE('',*,*,#9121,.T.);
#12566=ORIENTED_EDGE('',*,*,#9119,.T.);
#12567=ORIENTED_EDGE('',*,*,#9117,.T.);
#12568=ORIENTED_EDGE('',*,*,#9115,.T.);
#12569=ORIENTED_EDGE('',*,*,#9113,.T.);
#12570=ORIENTED_EDGE('',*,*,#9111,.T.);
#12571=ORIENTED_EDGE('',*,*,#9109,.T.);
#12572=ORIENTED_EDGE('',*,*,#9107,.T.);
#12573=ORIENTED_EDGE('',*,*,#9105,.T.);
#12574=ORIENTED_EDGE('',*,*,#9103,.T.);
#12575=ORIENTED_EDGE('',*,*,#9101,.T.);
#12576=ORIENTED_EDGE('',*,*,#9099,.T.);
#12577=ORIENTED_EDGE('',*,*,#9097,.T.);
#12578=ORIENTED_EDGE('',*,*,#9095,.T.);
#12579=ORIENTED_EDGE('',*,*,#9093,.T.);
#12580=ORIENTED_EDGE('',*,*,#9091,.T.);
#12581=ORIENTED_EDGE('',*,*,#9089,.T.);
#12582=ORIENTED_EDGE('',*,*,#9087,.T.);
#12583=ORIENTED_EDGE('',*,*,#9085,.T.);
#12584=ORIENTED_EDGE('',*,*,#9083,.T.);
#12585=ORIENTED_EDGE('',*,*,#9081,.T.);
#12586=ORIENTED_EDGE('',*,*,#9079,.T.);
#12587=ORIENTED_EDGE('',*,*,#9077,.T.);
#12588=ORIENTED_EDGE('',*,*,#9075,.T.);
#12589=ORIENTED_EDGE('',*,*,#9073,.T.);
#12590=ORIENTED_EDGE('',*,*,#9071,.T.);
#12591=ORIENTED_EDGE('',*,*,#9069,.T.);
#12592=ORIENTED_EDGE('',*,*,#9067,.T.);
#12593=ORIENTED_EDGE('',*,*,#9065,.T.);
#12594=ORIENTED_EDGE('',*,*,#9063,.T.);
#12595=ORIENTED_EDGE('',*,*,#9061,.T.);
#12596=ORIENTED_EDGE('',*,*,#9059,.T.);
#12597=ORIENTED_EDGE('',*,*,#9057,.T.);
#12598=ORIENTED_EDGE('',*,*,#9055,.T.);
#12599=ORIENTED_EDGE('',*,*,#9053,.T.);
#12600=ORIENTED_EDGE('',*,*,#9051,.T.);
#12601=ORIENTED_EDGE('',*,*,#9049,.T.);
#12602=ORIENTED_EDGE('',*,*,#9047,.T.);
#12603=ORIENTED_EDGE('',*,*,#9045,.T.);
#12604=ORIENTED_EDGE('',*,*,#9043,.T.);
#12605=ORIENTED_EDGE('',*,*,#9041,.T.);
#12606=ORIENTED_EDGE('',*,*,#9039,.T.);
#12607=ORIENTED_EDGE('',*,*,#9037,.T.);
#12608=ORIENTED_EDGE('',*,*,#9035,.T.);
#12609=ORIENTED_EDGE('',*,*,#9033,.T.);
#12610=ORIENTED_EDGE('',*,*,#9031,.T.);
#12611=ORIENTED_EDGE('',*,*,#9029,.T.);
#12612=ORIENTED_EDGE('',*,*,#9027,.T.);
#12613=ORIENTED_EDGE('',*,*,#9025,.T.);
#12614=ORIENTED_EDGE('',*,*,#9023,.T.);
#12615=ORIENTED_EDGE('',*,*,#9021,.T.);
#12616=ORIENTED_EDGE('',*,*,#9019,.T.);
#12617=ORIENTED_EDGE('',*,*,#9017,.T.);
#12618=ORIENTED_EDGE('',*,*,#9015,.T.);
#12619=ORIENTED_EDGE('',*,*,#9013,.T.);
#12620=ORIENTED_EDGE('',*,*,#9011,.T.);
#12621=ORIENTED_EDGE('',*,*,#9009,.T.);
#12622=ORIENTED_EDGE('',*,*,#9007,.T.);
#12623=ORIENTED_EDGE('',*,*,#9005,.T.);
#12624=ORIENTED_EDGE('',*,*,#9003,.T.);
#12625=ORIENTED_EDGE('',*,*,#9001,.T.);
#12626=ORIENTED_EDGE('',*,*,#8999,.T.);
#12627=ORIENTED_EDGE('',*,*,#8997,.T.);
#12628=ORIENTED_EDGE('',*,*,#8995,.T.);
#12629=ORIENTED_EDGE('',*,*,#8993,.T.);
#12630=ORIENTED_EDGE('',*,*,#8991,.T.);
#12631=ORIENTED_EDGE('',*,*,#8989,.T.);
#12632=ORIENTED_EDGE('',*,*,#8987,.T.);
#12633=ORIENTED_EDGE('',*,*,#8985,.T.);
#12634=ORIENTED_EDGE('',*,*,#8983,.T.);
#12635=ORIENTED_EDGE('',*,*,#8981,.T.);
#12636=ORIENTED_EDGE('',*,*,#8979,.T.);
#12637=ORIENTED_EDGE('',*,*,#8977,.T.);
#12638=ORIENTED_EDGE('',*,*,#8975,.T.);
#12639=ORIENTED_EDGE('',*,*,#8973,.T.);
#12640=ORIENTED_EDGE('',*,*,#8974,.T.);
#12641=ORIENTED_EDGE('',*,*,#8965,.F.);
#12642=ORIENTED_EDGE('',*,*,#9132,.T.);
#12643=ORIENTED_EDGE('',*,*,#9133,.F.);
#12983=CYLINDRICAL_SURFACE('',#15348,0.6);
#12984=CYLINDRICAL_SURFACE('',#15350,1.4);
#12985=CYLINDRICAL_SURFACE('',#15355,1.75);
#12986=CYLINDRICAL_SURFACE('',#15358,1.75);
#12987=CYLINDRICAL_SURFACE('',#15361,1.75);
#12988=CYLINDRICAL_SURFACE('',#15364,1.75);
#12989=CYLINDRICAL_SURFACE('',#15367,1.75);
#12990=CYLINDRICAL_SURFACE('',#15370,1.75);
#12991=CYLINDRICAL_SURFACE('',#15373,1.75);
#12992=CYLINDRICAL_SURFACE('',#15376,1.75);
#12993=CYLINDRICAL_SURFACE('',#15379,1.75);
#12994=CYLINDRICAL_SURFACE('',#15382,1.75);
#12995=CYLINDRICAL_SURFACE('',#15385,1.75);
#12996=CYLINDRICAL_SURFACE('',#15388,1.75);
#12997=CYLINDRICAL_SURFACE('',#15391,1.75);
#12998=CYLINDRICAL_SURFACE('',#15394,1.75);
#12999=CYLINDRICAL_SURFACE('',#15397,1.75);
#13000=CYLINDRICAL_SURFACE('',#15400,1.75);
#13001=CYLINDRICAL_SURFACE('',#15403,1.75);
#13002=CYLINDRICAL_SURFACE('',#15406,1.75);
#13003=CYLINDRICAL_SURFACE('',#15409,1.75);
#13004=CYLINDRICAL_SURFACE('',#15414,1.75);
#13612=ADVANCED_FACE('',(#2134),#1473,.F.);
#13613=ADVANCED_FACE('',(#2135),#1474,.F.);
#13614=ADVANCED_FACE('',(#2136),#1475,.F.);
#13615=ADVANCED_FACE('',(#2137,#1035),#1476,.F.);
#13616=ADVANCED_FACE('',(#2138),#12983,.F.);
#13617=ADVANCED_FACE('',(#2139),#12984,.T.);
#13618=ADVANCED_FACE('',(#2140,#1036),#1477,.T.);
#13619=ADVANCED_FACE('',(#2141),#11,.T.);
#13620=ADVANCED_FACE('',(#2142),#1478,.T.);
#13621=ADVANCED_FACE('',(#2143),#12,.T.);
#13622=ADVANCED_FACE('',(#2144),#12985,.T.);
#13623=ADVANCED_FACE('',(#2145),#13,.T.);
#13624=ADVANCED_FACE('',(#2146),#1479,.T.);
#13625=ADVANCED_FACE('',(#2147),#14,.T.);
#13626=ADVANCED_FACE('',(#2148),#12986,.T.);
#13627=ADVANCED_FACE('',(#2149),#15,.T.);
#13628=ADVANCED_FACE('',(#2150),#1480,.T.);
#13629=ADVANCED_FACE('',(#2151),#16,.T.);
#13630=ADVANCED_FACE('',(#2152),#12987,.T.);
#13631=ADVANCED_FACE('',(#2153),#17,.T.);
#13632=ADVANCED_FACE('',(#2154),#1481,.T.);
#13633=ADVANCED_FACE('',(#2155),#18,.T.);
#13634=ADVANCED_FACE('',(#2156),#12988,.T.);
#13635=ADVANCED_FACE('',(#2157),#19,.T.);
#13636=ADVANCED_FACE('',(#2158),#1482,.T.);
#13637=ADVANCED_FACE('',(#2159),#20,.T.);
#13638=ADVANCED_FACE('',(#2160),#12989,.T.);
#13639=ADVANCED_FACE('',(#2161),#21,.T.);
#13640=ADVANCED_FACE('',(#2162),#1483,.T.);
#13641=ADVANCED_FACE('',(#2163),#22,.T.);
#13642=ADVANCED_FACE('',(#2164),#12990,.T.);
#13643=ADVANCED_FACE('',(#2165),#23,.T.);
#13644=ADVANCED_FACE('',(#2166),#1484,.T.);
#13645=ADVANCED_FACE('',(#2167),#24,.T.);
#13646=ADVANCED_FACE('',(#2168),#12991,.T.);
#13647=ADVANCED_FACE('',(#2169),#25,.T.);
#13648=ADVANCED_FACE('',(#2170),#1485,.T.);
#13649=ADVANCED_FACE('',(#2171),#26,.T.);
#13650=ADVANCED_FACE('',(#2172),#12992,.T.);
#13651=ADVANCED_FACE('',(#2173),#27,.T.);
#13652=ADVANCED_FACE('',(#2174),#1486,.T.);
#13653=ADVANCED_FACE('',(#2175),#28,.T.);
#13654=ADVANCED_FACE('',(#2176),#12993,.T.);
#13655=ADVANCED_FACE('',(#2177),#29,.T.);
#13656=ADVANCED_FACE('',(#2178),#1487,.T.);
#13657=ADVANCED_FACE('',(#2179),#30,.T.);
#13658=ADVANCED_FACE('',(#2180),#12994,.T.);
#13659=ADVANCED_FACE('',(#2181),#31,.T.);
#13660=ADVANCED_FACE('',(#2182),#1488,.T.);
#13661=ADVANCED_FACE('',(#2183),#32,.T.);
#13662=ADVANCED_FACE('',(#2184),#12995,.T.);
#13663=ADVANCED_FACE('',(#2185),#33,.T.);
#13664=ADVANCED_FACE('',(#2186),#1489,.T.);
#13665=ADVANCED_FACE('',(#2187),#34,.T.);
#13666=ADVANCED_FACE('',(#2188),#12996,.T.);
#13667=ADVANCED_FACE('',(#2189),#35,.T.);
#13668=ADVANCED_FACE('',(#2190),#1490,.T.);
#13669=ADVANCED_FACE('',(#2191),#36,.T.);
#13670=ADVANCED_FACE('',(#2192),#12997,.T.);
#13671=ADVANCED_FACE('',(#2193),#37,.T.);
#13672=ADVANCED_FACE('',(#2194),#1491,.T.);
#13673=ADVANCED_FACE('',(#2195),#38,.T.);
#13674=ADVANCED_FACE('',(#2196),#12998,.T.);
#13675=ADVANCED_FACE('',(#2197),#39,.T.);
#13676=ADVANCED_FACE('',(#2198),#1492,.T.);
#13677=ADVANCED_FACE('',(#2199),#40,.T.);
#13678=ADVANCED_FACE('',(#2200),#12999,.T.);
#13679=ADVANCED_FACE('',(#2201),#41,.T.);
#13680=ADVANCED_FACE('',(#2202),#1493,.T.);
#13681=ADVANCED_FACE('',(#2203),#42,.T.);
#13682=ADVANCED_FACE('',(#2204),#13000,.T.);
#13683=ADVANCED_FACE('',(#2205),#43,.T.);
#13684=ADVANCED_FACE('',(#2206),#1494,.T.);
#13685=ADVANCED_FACE('',(#2207),#44,.T.);
#13686=ADVANCED_FACE('',(#2208),#13001,.T.);
#13687=ADVANCED_FACE('',(#2209),#45,.T.);
#13688=ADVANCED_FACE('',(#2210),#1495,.T.);
#13689=ADVANCED_FACE('',(#2211),#46,.T.);
#13690=ADVANCED_FACE('',(#2212),#13002,.T.);
#13691=ADVANCED_FACE('',(#2213),#47,.T.);
#13692=ADVANCED_FACE('',(#2214),#1496,.T.);
#13693=ADVANCED_FACE('',(#2215),#48,.T.);
#13694=ADVANCED_FACE('',(#2216),#13003,.T.);
#13695=ADVANCED_FACE('',(#2217),#49,.T.);
#13696=ADVANCED_FACE('',(#2218),#1497,.T.);
#13697=ADVANCED_FACE('',(#2219),#50,.T.);
#13698=ADVANCED_FACE('',(#2220,#1037),#1498,.T.);
#13699=ADVANCED_FACE('',(#2221),#13004,.T.);
#13802=CLOSED_SHELL('',(#13612,#13613,#13614,#13615,#13616,#13617,#13618,
#13619,#13620,#13621,#13622,#13623,#13624,#13625,#13626,#13627,#13628,#13629,
#13630,#13631,#13632,#13633,#13634,#13635,#13636,#13637,#13638,#13639,#13640,
#13641,#13642,#13643,#13644,#13645,#13646,#13647,#13648,#13649,#13650,#13651,
#13652,#13653,#13654,#13655,#13656,#13657,#13658,#13659,#13660,#13661,#13662,
#13663,#13664,#13665,#13666,#13667,#13668,#13669,#13670,#13671,#13672,#13673,
#13674,#13675,#13676,#13677,#13678,#13679,#13680,#13681,#13682,#13683,#13684,
#13685,#13686,#13687,#13688,#13689,#13690,#13691,#13692,#13693,#13694,#13695,
#13696,#13697,#13698,#13699));
#15322=AXIS2_PLACEMENT_3D('',#22825,#18694,#18695);
#15323=AXIS2_PLACEMENT_3D('',#22826,#18696,#18697);
#15324=AXIS2_PLACEMENT_3D('',#22835,#18702,#18703);
#15325=AXIS2_PLACEMENT_3D('',#22841,#18707,#18708);
#15326=AXIS2_PLACEMENT_3D('',#22847,#18712,#18713);
#15327=AXIS2_PLACEMENT_3D('',#22850,#18714,#18715);
#15328=AXIS2_PLACEMENT_3D('',#22996,#18717,#18718);
#15329=AXIS2_PLACEMENT_3D('',#23142,#18720,#18721);
#15330=AXIS2_PLACEMENT_3D('',#23288,#18723,#18724);
#15331=AXIS2_PLACEMENT_3D('',#23434,#18726,#18727);
#15332=AXIS2_PLACEMENT_3D('',#23580,#18729,#18730);
#15333=AXIS2_PLACEMENT_3D('',#23726,#18732,#18733);
#15334=AXIS2_PLACEMENT_3D('',#23872,#18735,#18736);
#15335=AXIS2_PLACEMENT_3D('',#24018,#18738,#18739);
#15336=AXIS2_PLACEMENT_3D('',#24164,#18741,#18742);
#15337=AXIS2_PLACEMENT_3D('',#24310,#18744,#18745);
#15338=AXIS2_PLACEMENT_3D('',#24456,#18747,#18748);
#15339=AXIS2_PLACEMENT_3D('',#24602,#18750,#18751);
#15340=AXIS2_PLACEMENT_3D('',#24748,#18753,#18754);
#15341=AXIS2_PLACEMENT_3D('',#24894,#18756,#18757);
#15342=AXIS2_PLACEMENT_3D('',#25040,#18759,#18760);
#15343=AXIS2_PLACEMENT_3D('',#25186,#18762,#18763);
#15344=AXIS2_PLACEMENT_3D('',#25332,#18765,#18766);
#15345=AXIS2_PLACEMENT_3D('',#25478,#18768,#18769);
#15346=AXIS2_PLACEMENT_3D('',#25624,#18771,#18772);
#15347=AXIS2_PLACEMENT_3D('',#25768,#18774,#18775);
#15348=AXIS2_PLACEMENT_3D('',#25769,#18776,#18777);
#15349=AXIS2_PLACEMENT_3D('',#25770,#18778,#18779);
#15350=AXIS2_PLACEMENT_3D('',#25771,#18780,#18781);
#15351=AXIS2_PLACEMENT_3D('',#25773,#18782,#18783);
#15352=AXIS2_PLACEMENT_3D('',#25776,#18785,#18786);
#15353=AXIS2_PLACEMENT_3D('',#25777,#18787,#18788);
#15354=AXIS2_PLACEMENT_3D('',#25992,#18791,#18792);
#15355=AXIS2_PLACEMENT_3D('',#26208,#18796,#18797);
#15356=AXIS2_PLACEMENT_3D('',#26210,#18798,#18799);
#15357=AXIS2_PLACEMENT_3D('',#26424,#18802,#18803);
#15358=AXIS2_PLACEMENT_3D('',#26640,#18807,#18808);
#15359=AXIS2_PLACEMENT_3D('',#26642,#18809,#18810);
#15360=AXIS2_PLACEMENT_3D('',#26856,#18813,#18814);
#15361=AXIS2_PLACEMENT_3D('',#27072,#18818,#18819);
#15362=AXIS2_PLACEMENT_3D('',#27074,#18820,#18821);
#15363=AXIS2_PLACEMENT_3D('',#27288,#18824,#18825);
#15364=AXIS2_PLACEMENT_3D('',#27504,#18829,#18830);
#15365=AXIS2_PLACEMENT_3D('',#27506,#18831,#18832);
#15366=AXIS2_PLACEMENT_3D('',#27720,#18835,#18836);
#15367=AXIS2_PLACEMENT_3D('',#27936,#18840,#18841);
#15368=AXIS2_PLACEMENT_3D('',#27938,#18842,#18843);
#15369=AXIS2_PLACEMENT_3D('',#28152,#18846,#18847);
#15370=AXIS2_PLACEMENT_3D('',#28368,#18851,#18852);
#15371=AXIS2_PLACEMENT_3D('',#28370,#18853,#18854);
#15372=AXIS2_PLACEMENT_3D('',#28584,#18857,#18858);
#15373=AXIS2_PLACEMENT_3D('',#28800,#18862,#18863);
#15374=AXIS2_PLACEMENT_3D('',#28802,#18864,#18865);
#15375=AXIS2_PLACEMENT_3D('',#29016,#18868,#18869);
#15376=AXIS2_PLACEMENT_3D('',#29232,#18873,#18874);
#15377=AXIS2_PLACEMENT_3D('',#29234,#18875,#18876);
#15378=AXIS2_PLACEMENT_3D('',#29448,#18879,#18880);
#15379=AXIS2_PLACEMENT_3D('',#29664,#18884,#18885);
#15380=AXIS2_PLACEMENT_3D('',#29666,#18886,#18887);
#15381=AXIS2_PLACEMENT_3D('',#29880,#18890,#18891);
#15382=AXIS2_PLACEMENT_3D('',#30096,#18895,#18896);
#15383=AXIS2_PLACEMENT_3D('',#30098,#18897,#18898);
#15384=AXIS2_PLACEMENT_3D('',#30312,#18901,#18902);
#15385=AXIS2_PLACEMENT_3D('',#30528,#18906,#18907);
#15386=AXIS2_PLACEMENT_3D('',#30530,#18908,#18909);
#15387=AXIS2_PLACEMENT_3D('',#30744,#18912,#18913);
#15388=AXIS2_PLACEMENT_3D('',#30960,#18917,#18918);
#15389=AXIS2_PLACEMENT_3D('',#30962,#18919,#18920);
#15390=AXIS2_PLACEMENT_3D('',#31176,#18923,#18924);
#15391=AXIS2_PLACEMENT_3D('',#31392,#18928,#18929);
#15392=AXIS2_PLACEMENT_3D('',#31394,#18930,#18931);
#15393=AXIS2_PLACEMENT_3D('',#31608,#18934,#18935);
#15394=AXIS2_PLACEMENT_3D('',#31824,#18939,#18940);
#15395=AXIS2_PLACEMENT_3D('',#31826,#18941,#18942);
#15396=AXIS2_PLACEMENT_3D('',#32040,#18945,#18946);
#15397=AXIS2_PLACEMENT_3D('',#32256,#18950,#18951);
#15398=AXIS2_PLACEMENT_3D('',#32258,#18952,#18953);
#15399=AXIS2_PLACEMENT_3D('',#32472,#18956,#18957);
#15400=AXIS2_PLACEMENT_3D('',#32688,#18961,#18962);
#15401=AXIS2_PLACEMENT_3D('',#32690,#18963,#18964);
#15402=AXIS2_PLACEMENT_3D('',#32904,#18967,#18968);
#15403=AXIS2_PLACEMENT_3D('',#33120,#18972,#18973);
#15404=AXIS2_PLACEMENT_3D('',#33122,#18974,#18975);
#15405=AXIS2_PLACEMENT_3D('',#33336,#18978,#18979);
#15406=AXIS2_PLACEMENT_3D('',#33552,#18983,#18984);
#15407=AXIS2_PLACEMENT_3D('',#33554,#18985,#18986);
#15408=AXIS2_PLACEMENT_3D('',#33768,#18989,#18990);
#15409=AXIS2_PLACEMENT_3D('',#33984,#18994,#18995);
#15410=AXIS2_PLACEMENT_3D('',#33986,#18996,#18997);
#15411=AXIS2_PLACEMENT_3D('',#34200,#19000,#19001);
#15412=AXIS2_PLACEMENT_3D('',#34416,#19005,#19006);
#15413=AXIS2_PLACEMENT_3D('',#34417,#19007,#19008);
#15414=AXIS2_PLACEMENT_3D('',#34418,#19009,#19010);
#18694=DIRECTION('axis',(0.,0.,1.));
#18695=DIRECTION('refdir',(1.,0.,0.));
#18696=DIRECTION('center_axis',(1.,0.,0.));
#18697=DIRECTION('ref_axis',(0.,0.,-1.));
#18698=DIRECTION('',(0.,0.,1.));
#18699=DIRECTION('',(0.,1.,0.));
#18700=DIRECTION('',(0.,0.,-1.));
#18701=DIRECTION('',(0.,-1.,0.));
#18702=DIRECTION('center_axis',(0.,0.,-1.));
#18703=DIRECTION('ref_axis',(-1.,0.,0.));
#18704=DIRECTION('',(1.,0.,0.));
#18705=DIRECTION('',(0.,-1.,0.));
#18706=DIRECTION('',(-1.,0.,0.));
#18707=DIRECTION('center_axis',(-1.,0.,0.));
#18708=DIRECTION('ref_axis',(0.,0.,1.));
#18709=DIRECTION('',(0.,0.,-1.));
#18710=DIRECTION('',(0.,1.,0.));
#18711=DIRECTION('',(0.,0.,1.));
#18712=DIRECTION('center_axis',(0.,1.,0.));
#18713=DIRECTION('ref_axis',(1.,0.,0.));
#18714=DIRECTION('center_axis',(0.,-1.,0.));
#18715=DIRECTION('ref_axis',(1.,0.,0.));
#18716=DIRECTION('',(-0.587785252292473,0.,0.809016994374947));
#18717=DIRECTION('center_axis',(0.,-1.,0.));
#18718=DIRECTION('ref_axis',(1.,0.,0.));
#18719=DIRECTION('',(-0.809016994374948,0.,0.587785252292473));
#18720=DIRECTION('center_axis',(0.,-1.,0.));
#18721=DIRECTION('ref_axis',(1.,0.,0.));
#18722=DIRECTION('',(-0.951056516295154,0.,0.309016994374947));
#18723=DIRECTION('center_axis',(0.,-1.,0.));
#18724=DIRECTION('ref_axis',(1.,0.,0.));
#18725=DIRECTION('',(-1.,0.,-1.83697019872103E-16));
#18726=DIRECTION('center_axis',(0.,-1.,0.));
#18727=DIRECTION('ref_axis',(1.,0.,0.));
#18728=DIRECTION('',(-0.951056516295154,0.,-0.309016994374948));
#18729=DIRECTION('center_axis',(0.,-1.,0.));
#18730=DIRECTION('ref_axis',(1.,0.,0.));
#18731=DIRECTION('',(-0.809016994374947,0.,-0.587785252292473));
#18732=DIRECTION('center_axis',(0.,-1.,0.));
#18733=DIRECTION('ref_axis',(1.,0.,0.));
#18734=DIRECTION('',(-0.587785252292473,0.,-0.809016994374948));
#18735=DIRECTION('center_axis',(0.,-1.,0.));
#18736=DIRECTION('ref_axis',(1.,0.,0.));
#18737=DIRECTION('',(-0.309016994374947,0.,-0.951056516295154));
#18738=DIRECTION('center_axis',(0.,-1.,0.));
#18739=DIRECTION('ref_axis',(1.,0.,0.));
#18740=DIRECTION('',(1.22464679914735E-16,0.,-1.));
#18741=DIRECTION('center_axis',(0.,-1.,0.));
#18742=DIRECTION('ref_axis',(1.,0.,0.));
#18743=DIRECTION('',(0.309016994374948,0.,-0.951056516295154));
#18744=DIRECTION('center_axis',(0.,-1.,0.));
#18745=DIRECTION('ref_axis',(1.,0.,0.));
#18746=DIRECTION('',(0.587785252292473,0.,-0.809016994374947));
#18747=DIRECTION('center_axis',(0.,-1.,0.));
#18748=DIRECTION('ref_axis',(1.,0.,0.));
#18749=DIRECTION('',(0.809016994374948,0.,-0.587785252292473));
#18750=DIRECTION('center_axis',(0.,-1.,0.));
#18751=DIRECTION('ref_axis',(1.,0.,0.));
#18752=DIRECTION('',(0.951056516295154,0.,-0.309016994374947));
#18753=DIRECTION('center_axis',(0.,-1.,0.));
#18754=DIRECTION('ref_axis',(1.,0.,0.));
#18755=DIRECTION('',(1.,0.,6.12323399573677E-17));
#18756=DIRECTION('center_axis',(0.,-1.,0.));
#18757=DIRECTION('ref_axis',(1.,0.,0.));
#18758=DIRECTION('',(0.951056516295154,0.,0.309016994374948));
#18759=DIRECTION('center_axis',(0.,-1.,0.));
#18760=DIRECTION('ref_axis',(1.,0.,0.));
#18761=DIRECTION('',(0.809016994374947,0.,0.587785252292473));
#18762=DIRECTION('center_axis',(0.,-1.,0.));
#18763=DIRECTION('ref_axis',(1.,0.,0.));
#18764=DIRECTION('',(0.587785252292473,0.,0.809016994374947));
#18765=DIRECTION('center_axis',(0.,-1.,0.));
#18766=DIRECTION('ref_axis',(1.,0.,0.));
#18767=DIRECTION('',(0.309016994374947,0.,0.951056516295154));
#18768=DIRECTION('center_axis',(0.,-1.,0.));
#18769=DIRECTION('ref_axis',(1.,0.,0.));
#18770=DIRECTION('',(0.,0.,1.));
#18771=DIRECTION('center_axis',(0.,-1.,0.));
#18772=DIRECTION('ref_axis',(1.,0.,0.));
#18773=DIRECTION('',(-0.309016994374948,0.,0.951056516295154));
#18774=DIRECTION('center_axis',(0.,1.,0.));
#18775=DIRECTION('ref_axis',(1.,0.,0.));
#18776=DIRECTION('center_axis',(0.,1.,0.));
#18777=DIRECTION('ref_axis',(6.12323399573677E-17,0.,1.));
#18778=DIRECTION('center_axis',(0.,-1.,0.));
#18779=DIRECTION('ref_axis',(1.,0.,0.));
#18780=DIRECTION('center_axis',(0.,1.,0.));
#18781=DIRECTION('ref_axis',(1.,0.,0.));
#18782=DIRECTION('center_axis',(0.,1.,0.));
#18783=DIRECTION('ref_axis',(1.,0.,0.));
#18784=DIRECTION('',(0.,-1.,0.));
#18785=DIRECTION('center_axis',(0.,-1.,0.));
#18786=DIRECTION('ref_axis',(1.,0.,0.));
#18787=DIRECTION('center_axis',(0.,1.,0.));
#18788=DIRECTION('ref_axis',(1.,0.,0.));
#18789=DIRECTION('',(0.,-1.,0.));
#18790=DIRECTION('',(0.,1.,0.));
#18791=DIRECTION('center_axis',(0.951056516295154,0.,0.309016994374948));
#18792=DIRECTION('ref_axis',(0.309016994374948,0.,-0.951056516295154));
#18793=DIRECTION('',(0.309016994374948,0.,-0.951056516295154));
#18794=DIRECTION('',(0.,1.,0.));
#18795=DIRECTION('',(0.,1.,0.));
#18796=DIRECTION('center_axis',(0.,1.,0.));
#18797=DIRECTION('ref_axis',(1.,0.,0.));
#18798=DIRECTION('center_axis',(0.,1.,0.));
#18799=DIRECTION('ref_axis',(1.,0.,0.));
#18800=DIRECTION('',(0.,-1.,0.));
#18801=DIRECTION('',(0.,1.,0.));
#18802=DIRECTION('center_axis',(0.809016994374947,0.,0.587785252292473));
#18803=DIRECTION('ref_axis',(0.587785252292473,0.,-0.809016994374947));
#18804=DIRECTION('',(0.587785252292473,0.,-0.809016994374947));
#18805=DIRECTION('',(0.,1.,0.));
#18806=DIRECTION('',(0.,1.,0.));
#18807=DIRECTION('center_axis',(0.,1.,0.));
#18808=DIRECTION('ref_axis',(1.,0.,0.));
#18809=DIRECTION('center_axis',(0.,1.,0.));
#18810=DIRECTION('ref_axis',(1.,0.,0.));
#18811=DIRECTION('',(0.,-1.,0.));
#18812=DIRECTION('',(0.,1.,0.));
#18813=DIRECTION('center_axis',(0.587785252292473,0.,0.809016994374948));
#18814=DIRECTION('ref_axis',(0.809016994374948,0.,-0.587785252292473));
#18815=DIRECTION('',(0.809016994374948,0.,-0.587785252292473));
#18816=DIRECTION('',(0.,1.,0.));
#18817=DIRECTION('',(0.,1.,0.));
#18818=DIRECTION('center_axis',(0.,1.,0.));
#18819=DIRECTION('ref_axis',(1.,0.,0.));
#18820=DIRECTION('center_axis',(0.,1.,0.));
#18821=DIRECTION('ref_axis',(1.,0.,0.));
#18822=DIRECTION('',(0.,-1.,0.));
#18823=DIRECTION('',(0.,1.,0.));
#18824=DIRECTION('center_axis',(0.309016994374947,0.,0.951056516295154));
#18825=DIRECTION('ref_axis',(0.951056516295154,0.,-0.309016994374947));
#18826=DIRECTION('',(0.951056516295154,0.,-0.309016994374947));
#18827=DIRECTION('',(0.,1.,0.));
#18828=DIRECTION('',(0.,1.,0.));
#18829=DIRECTION('center_axis',(0.,1.,0.));
#18830=DIRECTION('ref_axis',(1.,0.,0.));
#18831=DIRECTION('center_axis',(0.,1.,0.));
#18832=DIRECTION('ref_axis',(1.,0.,0.));
#18833=DIRECTION('',(0.,-1.,0.));
#18834=DIRECTION('',(0.,1.,0.));
#18835=DIRECTION('center_axis',(-1.83697019872103E-16,0.,1.));
#18836=DIRECTION('ref_axis',(1.,0.,1.83697019872103E-16));
#18837=DIRECTION('',(1.,0.,1.83697019872103E-16));
#18838=DIRECTION('',(0.,1.,0.));
#18839=DIRECTION('',(0.,1.,0.));
#18840=DIRECTION('center_axis',(0.,1.,0.));
#18841=DIRECTION('ref_axis',(1.,0.,0.));
#18842=DIRECTION('center_axis',(0.,1.,0.));
#18843=DIRECTION('ref_axis',(1.,0.,0.));
#18844=DIRECTION('',(0.,-1.,0.));
#18845=DIRECTION('',(0.,1.,0.));
#18846=DIRECTION('center_axis',(-0.309016994374948,0.,0.951056516295154));
#18847=DIRECTION('ref_axis',(0.951056516295154,0.,0.309016994374948));
#18848=DIRECTION('',(0.951056516295154,0.,0.309016994374948));
#18849=DIRECTION('',(0.,1.,0.));
#18850=DIRECTION('',(0.,1.,0.));
#18851=DIRECTION('center_axis',(0.,1.,0.));
#18852=DIRECTION('ref_axis',(1.,0.,0.));
#18853=DIRECTION('center_axis',(0.,1.,0.));
#18854=DIRECTION('ref_axis',(1.,0.,0.));
#18855=DIRECTION('',(0.,-1.,0.));
#18856=DIRECTION('',(0.,1.,0.));
#18857=DIRECTION('center_axis',(-0.587785252292473,0.,0.809016994374947));
#18858=DIRECTION('ref_axis',(0.809016994374947,0.,0.587785252292473));
#18859=DIRECTION('',(0.809016994374947,0.,0.587785252292473));
#18860=DIRECTION('',(0.,1.,0.));
#18861=DIRECTION('',(0.,1.,0.));
#18862=DIRECTION('center_axis',(0.,1.,0.));
#18863=DIRECTION('ref_axis',(1.,0.,0.));
#18864=DIRECTION('center_axis',(0.,1.,0.));
#18865=DIRECTION('ref_axis',(1.,0.,0.));
#18866=DIRECTION('',(0.,-1.,0.));
#18867=DIRECTION('',(0.,1.,0.));
#18868=DIRECTION('center_axis',(-0.809016994374948,0.,0.587785252292473));
#18869=DIRECTION('ref_axis',(0.587785252292473,0.,0.809016994374948));
#18870=DIRECTION('',(0.587785252292473,0.,0.809016994374948));
#18871=DIRECTION('',(0.,1.,0.));
#18872=DIRECTION('',(0.,1.,0.));
#18873=DIRECTION('center_axis',(0.,1.,0.));
#18874=DIRECTION('ref_axis',(1.,0.,0.));
#18875=DIRECTION('center_axis',(0.,1.,0.));
#18876=DIRECTION('ref_axis',(1.,0.,0.));
#18877=DIRECTION('',(0.,-1.,0.));
#18878=DIRECTION('',(0.,1.,0.));
#18879=DIRECTION('center_axis',(-0.951056516295154,0.,0.309016994374947));
#18880=DIRECTION('ref_axis',(0.309016994374947,0.,0.951056516295154));
#18881=DIRECTION('',(0.309016994374947,0.,0.951056516295154));
#18882=DIRECTION('',(0.,1.,0.));
#18883=DIRECTION('',(0.,1.,0.));
#18884=DIRECTION('center_axis',(0.,1.,0.));
#18885=DIRECTION('ref_axis',(1.,0.,0.));
#18886=DIRECTION('center_axis',(0.,1.,0.));
#18887=DIRECTION('ref_axis',(1.,0.,0.));
#18888=DIRECTION('',(0.,-1.,0.));
#18889=DIRECTION('',(0.,1.,0.));
#18890=DIRECTION('center_axis',(-1.,0.,-1.22464679914735E-16));
#18891=DIRECTION('ref_axis',(-1.22464679914735E-16,0.,1.));
#18892=DIRECTION('',(-1.22464679914735E-16,0.,1.));
#18893=DIRECTION('',(0.,1.,0.));
#18894=DIRECTION('',(0.,1.,0.));
#18895=DIRECTION('center_axis',(0.,1.,0.));
#18896=DIRECTION('ref_axis',(1.,0.,0.));
#18897=DIRECTION('center_axis',(0.,1.,0.));
#18898=DIRECTION('ref_axis',(1.,0.,0.));
#18899=DIRECTION('',(0.,-1.,0.));
#18900=DIRECTION('',(0.,1.,0.));
#18901=DIRECTION('center_axis',(-0.951056516295154,0.,-0.309016994374948));
#18902=DIRECTION('ref_axis',(-0.309016994374948,0.,0.951056516295154));
#18903=DIRECTION('',(-0.309016994374948,0.,0.951056516295154));
#18904=DIRECTION('',(0.,1.,0.));
#18905=DIRECTION('',(0.,1.,0.));
#18906=DIRECTION('center_axis',(0.,1.,0.));
#18907=DIRECTION('ref_axis',(1.,0.,0.));
#18908=DIRECTION('center_axis',(0.,1.,0.));
#18909=DIRECTION('ref_axis',(1.,0.,0.));
#18910=DIRECTION('',(0.,-1.,0.));
#18911=DIRECTION('',(0.,1.,0.));
#18912=DIRECTION('center_axis',(-0.809016994374947,0.,-0.587785252292473));
#18913=DIRECTION('ref_axis',(-0.587785252292473,0.,0.809016994374947));
#18914=DIRECTION('',(-0.587785252292473,0.,0.809016994374947));
#18915=DIRECTION('',(0.,1.,0.));
#18916=DIRECTION('',(0.,1.,0.));
#18917=DIRECTION('center_axis',(0.,1.,0.));
#18918=DIRECTION('ref_axis',(1.,0.,0.));
#18919=DIRECTION('center_axis',(0.,1.,0.));
#18920=DIRECTION('ref_axis',(1.,0.,0.));
#18921=DIRECTION('',(0.,-1.,0.));
#18922=DIRECTION('',(0.,1.,0.));
#18923=DIRECTION('center_axis',(-0.587785252292473,0.,-0.809016994374948));
#18924=DIRECTION('ref_axis',(-0.809016994374948,0.,0.587785252292473));
#18925=DIRECTION('',(-0.809016994374948,0.,0.587785252292473));
#18926=DIRECTION('',(0.,1.,0.));
#18927=DIRECTION('',(0.,1.,0.));
#18928=DIRECTION('center_axis',(0.,1.,0.));
#18929=DIRECTION('ref_axis',(1.,0.,0.));
#18930=DIRECTION('center_axis',(0.,1.,0.));
#18931=DIRECTION('ref_axis',(1.,0.,0.));
#18932=DIRECTION('',(0.,-1.,0.));
#18933=DIRECTION('',(0.,1.,0.));
#18934=DIRECTION('center_axis',(-0.309016994374947,0.,-0.951056516295154));
#18935=DIRECTION('ref_axis',(-0.951056516295154,0.,0.309016994374947));
#18936=DIRECTION('',(-0.951056516295154,0.,0.309016994374947));
#18937=DIRECTION('',(0.,1.,0.));
#18938=DIRECTION('',(0.,1.,0.));
#18939=DIRECTION('center_axis',(0.,1.,0.));
#18940=DIRECTION('ref_axis',(1.,0.,0.));
#18941=DIRECTION('center_axis',(0.,1.,0.));
#18942=DIRECTION('ref_axis',(1.,0.,0.));
#18943=DIRECTION('',(0.,-1.,0.));
#18944=DIRECTION('',(0.,1.,0.));
#18945=DIRECTION('center_axis',(6.12323399573677E-17,0.,-1.));
#18946=DIRECTION('ref_axis',(-1.,0.,-6.12323399573677E-17));
#18947=DIRECTION('',(-1.,0.,-6.12323399573677E-17));
#18948=DIRECTION('',(0.,1.,0.));
#18949=DIRECTION('',(0.,1.,0.));
#18950=DIRECTION('center_axis',(0.,1.,0.));
#18951=DIRECTION('ref_axis',(1.,0.,0.));
#18952=DIRECTION('center_axis',(0.,1.,0.));
#18953=DIRECTION('ref_axis',(1.,0.,0.));
#18954=DIRECTION('',(0.,-1.,0.));
#18955=DIRECTION('',(0.,1.,0.));
#18956=DIRECTION('center_axis',(0.309016994374948,0.,-0.951056516295154));
#18957=DIRECTION('ref_axis',(-0.951056516295154,0.,-0.309016994374948));
#18958=DIRECTION('',(-0.951056516295154,0.,-0.309016994374948));
#18959=DIRECTION('',(0.,1.,0.));
#18960=DIRECTION('',(0.,1.,0.));
#18961=DIRECTION('center_axis',(0.,1.,0.));
#18962=DIRECTION('ref_axis',(1.,0.,0.));
#18963=DIRECTION('center_axis',(0.,1.,0.));
#18964=DIRECTION('ref_axis',(1.,0.,0.));
#18965=DIRECTION('',(0.,-1.,0.));
#18966=DIRECTION('',(0.,1.,0.));
#18967=DIRECTION('center_axis',(0.587785252292473,0.,-0.809016994374947));
#18968=DIRECTION('ref_axis',(-0.809016994374947,0.,-0.587785252292473));
#18969=DIRECTION('',(-0.809016994374947,0.,-0.587785252292473));
#18970=DIRECTION('',(0.,1.,0.));
#18971=DIRECTION('',(0.,1.,0.));
#18972=DIRECTION('center_axis',(0.,1.,0.));
#18973=DIRECTION('ref_axis',(1.,0.,0.));
#18974=DIRECTION('center_axis',(0.,1.,0.));
#18975=DIRECTION('ref_axis',(1.,0.,0.));
#18976=DIRECTION('',(0.,-1.,0.));
#18977=DIRECTION('',(0.,1.,0.));
#18978=DIRECTION('center_axis',(0.809016994374947,0.,-0.587785252292473));
#18979=DIRECTION('ref_axis',(-0.587785252292473,0.,-0.809016994374947));
#18980=DIRECTION('',(-0.587785252292473,0.,-0.809016994374947));
#18981=DIRECTION('',(0.,1.,0.));
#18982=DIRECTION('',(0.,1.,0.));
#18983=DIRECTION('center_axis',(0.,1.,0.));
#18984=DIRECTION('ref_axis',(1.,0.,0.));
#18985=DIRECTION('center_axis',(0.,1.,0.));
#18986=DIRECTION('ref_axis',(1.,0.,0.));
#18987=DIRECTION('',(0.,-1.,0.));
#18988=DIRECTION('',(0.,1.,0.));
#18989=DIRECTION('center_axis',(0.951056516295154,0.,-0.309016994374947));
#18990=DIRECTION('ref_axis',(-0.309016994374947,0.,-0.951056516295154));
#18991=DIRECTION('',(-0.309016994374947,0.,-0.951056516295154));
#18992=DIRECTION('',(0.,1.,0.));
#18993=DIRECTION('',(0.,1.,0.));
#18994=DIRECTION('center_axis',(0.,1.,0.));
#18995=DIRECTION('ref_axis',(1.,0.,0.));
#18996=DIRECTION('center_axis',(0.,1.,0.));
#18997=DIRECTION('ref_axis',(1.,0.,0.));
#18998=DIRECTION('',(0.,-1.,0.));
#18999=DIRECTION('',(0.,1.,0.));
#19000=DIRECTION('center_axis',(1.,0.,0.));
#19001=DIRECTION('ref_axis',(0.,0.,-1.));
#19002=DIRECTION('',(0.,0.,-1.));
#19003=DIRECTION('',(0.,1.,0.));
#19004=DIRECTION('',(0.,1.,0.));
#19005=DIRECTION('center_axis',(0.,1.,0.));
#19006=DIRECTION('ref_axis',(1.,0.,0.));
#19007=DIRECTION('center_axis',(0.,1.,0.));
#19008=DIRECTION('ref_axis',(1.,0.,0.));
#19009=DIRECTION('center_axis',(0.,1.,0.));
#19010=DIRECTION('ref_axis',(1.,0.,0.));
#22825=CARTESIAN_POINT('',(0.,0.,0.));
#22826=CARTESIAN_POINT('Origin',(0.2,0.,0.));
#22827=CARTESIAN_POINT('',(0.2,2.2,-0.78));
#22828=CARTESIAN_POINT('',(0.2,2.2,-0.565685424949238));
#22829=CARTESIAN_POINT('',(0.2,2.2,0.));
#22830=CARTESIAN_POINT('',(0.2,-1.,-0.78));
#22831=CARTESIAN_POINT('',(0.2,0.,-0.78));
#22832=CARTESIAN_POINT('',(0.2,-1.,-0.565685424949238));
#22833=CARTESIAN_POINT('',(0.2,-1.,0.));
#22834=CARTESIAN_POINT('',(0.2,0.,-0.565685424949238));
#22835=CARTESIAN_POINT('Origin',(0.2,0.,-0.78));
#22836=CARTESIAN_POINT('',(-0.2,2.2,-0.78));
#22837=CARTESIAN_POINT('',(0.1,2.2,-0.78));
#22838=CARTESIAN_POINT('',(-0.2,-1.,-0.78));
#22839=CARTESIAN_POINT('',(-0.2,0.,-0.78));
#22840=CARTESIAN_POINT('',(0.1,-1.,-0.78));
#22841=CARTESIAN_POINT('Origin',(-0.2,0.,-0.78));
#22842=CARTESIAN_POINT('',(-0.2,2.2,-0.565685424949238));
#22843=CARTESIAN_POINT('',(-0.2,2.2,-0.39));
#22844=CARTESIAN_POINT('',(-0.2,-1.,-0.565685424949238));
#22845=CARTESIAN_POINT('',(-0.2,0.,-0.565685424949238));
#22846=CARTESIAN_POINT('',(-0.2,-1.,-0.39));
#22847=CARTESIAN_POINT('Origin',(0.,-1.,0.));
#22848=CARTESIAN_POINT('',(1.60662857109684,-1.,0.693717979106306));
#22849=CARTESIAN_POINT('',(1.5055822144029,-1.,0.892032620296856));
#22850=CARTESIAN_POINT('Origin',(0.,-1.,0.));
#22851=CARTESIAN_POINT('',(1.81978687191668,-1.,1.23627494547115));
#22852=CARTESIAN_POINT('Ctrl Pts',(1.5055822144029,-1.,0.892032620296856));
#22853=CARTESIAN_POINT('Ctrl Pts',(1.50980486806688,-1.,0.894452006964544));
#22854=CARTESIAN_POINT('Ctrl Pts',(1.51805569590094,-1.,0.899185047483511));
#22855=CARTESIAN_POINT('Ctrl Pts',(1.52984849887993,-1.,0.905967409625651));
#22856=CARTESIAN_POINT('Ctrl Pts',(1.54440491149498,-1.,0.914375919026456));
#22857=CARTESIAN_POINT('Ctrl Pts',(1.56065988578893,-1.,0.923832188944341));
#22858=CARTESIAN_POINT('Ctrl Pts',(1.57499388382243,-1.,0.932246680108685));
#22859=CARTESIAN_POINT('Ctrl Pts',(1.58744937487176,-1.,0.939646377893399));
#22860=CARTESIAN_POINT('Ctrl Pts',(1.59810042043673,-1.,0.946078063315257));
#22861=CARTESIAN_POINT('Ctrl Pts',(1.60706069896936,-1.,0.951613284356035));
#22862=CARTESIAN_POINT('Ctrl Pts',(1.61449324337085,-1.,0.956354422920671));
#22863=CARTESIAN_POINT('Ctrl Pts',(1.62061638140221,-1.,0.960438326101729));
#22864=CARTESIAN_POINT('Ctrl Pts',(1.62571930670187,-1.,0.964046107040536));
#22865=CARTESIAN_POINT('Ctrl Pts',(1.63013849959461,-1.,0.967387853230345));
#22866=CARTESIAN_POINT('Ctrl Pts',(1.63420665729798,-1.,0.970669715997509));
#22867=CARTESIAN_POINT('Ctrl Pts',(1.63820952658144,-1.,0.974066058287419));
#22868=CARTESIAN_POINT('Ctrl Pts',(1.64233990826687,-1.,0.977689794119417));
#22869=CARTESIAN_POINT('Ctrl Pts',(1.64665139190656,-1.,0.981562530939489));
#22870=CARTESIAN_POINT('Ctrl Pts',(1.65110016612638,-1.,0.985642622920821));
#22871=CARTESIAN_POINT('Ctrl Pts',(1.65559044289699,-1.,0.989855627854165));
#22872=CARTESIAN_POINT('Ctrl Pts',(1.66001553809947,-1.,0.994121836661306));
#22873=CARTESIAN_POINT('Ctrl Pts',(1.66430758030376,-1.,0.998389654952758));
#22874=CARTESIAN_POINT('Ctrl Pts',(1.66846059277303,-1.,1.00265091003727));
#22875=CARTESIAN_POINT('Ctrl Pts',(1.67250335383293,-1.,1.00692206696414));
#22876=CARTESIAN_POINT('Ctrl Pts',(1.67648246776464,-1.,1.01123236493511));
#22877=CARTESIAN_POINT('Ctrl Pts',(1.68044289894798,-1.,1.01561026162773));
#22878=CARTESIAN_POINT('Ctrl Pts',(1.68440578021706,-1.,1.02006795074201));
#22879=CARTESIAN_POINT('Ctrl Pts',(1.68836910178447,-1.,1.02460180535255));
#22880=CARTESIAN_POINT('Ctrl Pts',(1.69231840863458,-1.,1.02919977579147));
#22881=CARTESIAN_POINT('Ctrl Pts',(1.69623414782771,-1.,1.03384646003588));
#22882=CARTESIAN_POINT('Ctrl Pts',(1.70010052930962,-1.,1.03852922490789));
#22883=CARTESIAN_POINT('Ctrl Pts',(1.70391338707982,-1.,1.04324363334554));
#22884=CARTESIAN_POINT('Ctrl Pts',(1.70767646263649,-1.,1.04799085404995));
#22885=CARTESIAN_POINT('Ctrl Pts',(1.71139783543989,-1.,1.05277517202855));
#22886=CARTESIAN_POINT('Ctrl Pts',(1.7150865442702,-1.,1.05760163192479));
#22887=CARTESIAN_POINT('Ctrl Pts',(1.71874858456904,-1.,1.06247324680647));
#22888=CARTESIAN_POINT('Ctrl Pts',(1.72238500928453,-1.,1.06738966975462));
#22889=CARTESIAN_POINT('Ctrl Pts',(1.72599406198488,-1.,1.07234866990252));
#22890=CARTESIAN_POINT('Ctrl Pts',(1.72957248977424,-1.,1.0773470373727));
#22891=CARTESIAN_POINT('Ctrl Pts',(1.73311705663407,-1.,1.08238162784749));
#22892=CARTESIAN_POINT('Ctrl Pts',(1.73662628326091,-1.,1.08745056285427));
#22893=CARTESIAN_POINT('Ctrl Pts',(1.74010053962247,-1.,1.09255329056493));
#22894=CARTESIAN_POINT('Ctrl Pts',(1.74354119236208,-1.,1.09768999241226));
#22895=CARTESIAN_POINT('Ctrl Pts',(1.74695004214923,-1.,1.10286118991143));
#22896=CARTESIAN_POINT('Ctrl Pts',(1.7503286607592,-1.,1.10806728183007));
#22897=CARTESIAN_POINT('Ctrl Pts',(1.7536777209463,-1.,1.11330807582551));
#22898=CARTESIAN_POINT('Ctrl Pts',(1.75699720772105,-1.,1.11858293216763));
#22899=CARTESIAN_POINT('Ctrl Pts',(1.76028671825096,-1.,1.12389096855086));
#22900=CARTESIAN_POINT('Ctrl Pts',(1.7635457196617,-1.,1.12923123555075));
#22901=CARTESIAN_POINT('Ctrl Pts',(1.76677384551862,-1.,1.1346029180462));
#22902=CARTESIAN_POINT('Ctrl Pts',(1.76997111386769,-1.,1.14000548336975));
#22903=CARTESIAN_POINT('Ctrl Pts',(1.77313777896194,-1.,1.1454385822692));
#22904=CARTESIAN_POINT('Ctrl Pts',(1.7762742255701,-1.,1.15090197841515));
#22905=CARTESIAN_POINT('Ctrl Pts',(1.77938085564275,-1.,1.15639547194698));
#22906=CARTESIAN_POINT('Ctrl Pts',(1.78245795881009,-1.,1.16191881298499));
#22907=CARTESIAN_POINT('Ctrl Pts',(1.78550566040443,-1.,1.16747166312303));
#22908=CARTESIAN_POINT('Ctrl Pts',(1.78852398877616,-1.,1.17305363177328));
#22909=CARTESIAN_POINT('Ctrl Pts',(1.79151291552689,-1.,1.17866429440809));
#22910=CARTESIAN_POINT('Ctrl Pts',(1.79447240321515,-1.,1.18430321697432));
#22911=CARTESIAN_POINT('Ctrl Pts',(1.79740245923478,-1.,1.18996997934445));
#22912=CARTESIAN_POINT('Ctrl Pts',(1.80030314369879,-1.,1.19566418930242));
#22913=CARTESIAN_POINT('Ctrl Pts',(1.80317454838603,-1.,1.20138548938974));
#22914=CARTESIAN_POINT('Ctrl Pts',(1.80601678480707,-1.,1.20713356605475));
#22915=CARTESIAN_POINT('Ctrl Pts',(1.80882996917129,-1.,1.21290815708314));
#22916=CARTESIAN_POINT('Ctrl Pts',(1.81161420806656,-1.,1.21870906103557));
#22917=CARTESIAN_POINT('Ctrl Pts',(1.81436959210434,-1.,1.2245361330495));
#22918=CARTESIAN_POINT('Ctrl Pts',(1.8165508718364,-1.,1.2292186489137));
#22919=CARTESIAN_POINT('Ctrl Pts',(1.81817389921279,-1.,1.2327422452705));
#22920=CARTESIAN_POINT('Ctrl Pts',(1.81925017193666,-1.,1.23509651170476));
#22921=CARTESIAN_POINT('Ctrl Pts',(1.81978687191668,-1.,1.23627494547115));
#22922=CARTESIAN_POINT('',(1.73811241238545,-1.,1.34869019493419));
#22923=CARTESIAN_POINT('',(1.81978687191668,-1.,1.23627494547115));
#22924=CARTESIAN_POINT('',(1.31362392696032,-1.,1.15624053661742));
#22925=CARTESIAN_POINT('Ctrl Pts',(1.73811241238545,-1.,1.34869019493419));
#22926=CARTESIAN_POINT('Ctrl Pts',(1.73682580585691,-1.,1.34854391898045));
#22927=CARTESIAN_POINT('Ctrl Pts',(1.73425417885907,-1.,1.34824783112887));
#22928=CARTESIAN_POINT('Ctrl Pts',(1.7304014965394,-1.,1.34779309152035));
#22929=CARTESIAN_POINT('Ctrl Pts',(1.72527410680674,-1.,1.34716554819527));
#22930=CARTESIAN_POINT('Ctrl Pts',(1.7188807715049,-1.,1.34634568653227));
#22931=CARTESIAN_POINT('Ctrl Pts',(1.71250340686822,-1.,1.34549029589416));
#22932=CARTESIAN_POINT('Ctrl Pts',(1.70614212266738,-1.,1.34459924533831));
#22933=CARTESIAN_POINT('Ctrl Pts',(1.69979707754427,-1.,1.34367237124483));
#22934=CARTESIAN_POINT('Ctrl Pts',(1.6934684849687,-1.,1.34270948206319));
#22935=CARTESIAN_POINT('Ctrl Pts',(1.68715660868764,-1.,1.341710374848));
#22936=CARTESIAN_POINT('Ctrl Pts',(1.68086176030362,-1.,1.34067485185203));
#22937=CARTESIAN_POINT('Ctrl Pts',(1.67458429426086,-1.,1.3396027347034));
#22938=CARTESIAN_POINT('Ctrl Pts',(1.66832460783989,-1.,1.33849388654388));
#22939=CARTESIAN_POINT('Ctrl Pts',(1.66208312541983,-1.,1.33734820885262));
#22940=CARTESIAN_POINT('Ctrl Pts',(1.65586025952593,-1.,1.33616559745172));
#22941=CARTESIAN_POINT('Ctrl Pts',(1.6496563728683,-1.,1.33494590467993));
#22942=CARTESIAN_POINT('Ctrl Pts',(1.6434717485603,-1.,1.33368890676572));
#22943=CARTESIAN_POINT('Ctrl Pts',(1.63730653475089,-1.,1.33239425103724));
#22944=CARTESIAN_POINT('Ctrl Pts',(1.63116079730923,-1.,1.33106149345645));
#22945=CARTESIAN_POINT('Ctrl Pts',(1.62503464209797,-1.,1.3296901950568));
#22946=CARTESIAN_POINT('Ctrl Pts',(1.61892832270724,-1.,1.32828000610449));
#22947=CARTESIAN_POINT('Ctrl Pts',(1.6128423401575,-1.,1.32683074483356));
#22948=CARTESIAN_POINT('Ctrl Pts',(1.60677758290954,-1.,1.32534250785782));
#22949=CARTESIAN_POINT('Ctrl Pts',(1.60073511858687,-1.,1.32381550858256));
#22950=CARTESIAN_POINT('Ctrl Pts',(1.59471591079403,-1.,1.32224985747682));
#22951=CARTESIAN_POINT('Ctrl Pts',(1.58872057258245,-1.,1.32064537110892));
#22952=CARTESIAN_POINT('Ctrl Pts',(1.58274907898834,-1.,1.31900135021432));
#22953=CARTESIAN_POINT('Ctrl Pts',(1.5768005650559,-1.,1.31731642317187));
#22954=CARTESIAN_POINT('Ctrl Pts',(1.57087397835723,-1.,1.31558903860016));
#22955=CARTESIAN_POINT('Ctrl Pts',(1.56496872402353,-1.,1.31381795281002));
#22956=CARTESIAN_POINT('Ctrl Pts',(1.55908521254821,-1.,1.31200264341696));
#22957=CARTESIAN_POINT('Ctrl Pts',(1.55322568759481,-1.,1.31014393684222));
#22958=CARTESIAN_POINT('Ctrl Pts',(1.54739413957185,-1.,1.30824393907473));
#22959=CARTESIAN_POINT('Ctrl Pts',(1.54159462645432,-1.,1.30630475189556));
#22960=CARTESIAN_POINT('Ctrl Pts',(1.53582981268977,-1.,1.30432735639489));
#22961=CARTESIAN_POINT('Ctrl Pts',(1.53009970283891,-1.,1.30231064395568));
#22962=CARTESIAN_POINT('Ctrl Pts',(1.52439957861062,-1.,1.30024984366328));
#22963=CARTESIAN_POINT('Ctrl Pts',(1.51872184912724,-1.,1.29813791800747));
#22964=CARTESIAN_POINT('Ctrl Pts',(1.51305994241402,-1.,1.29596850710509));
#22965=CARTESIAN_POINT('Ctrl Pts',(1.50741159078365,-1.,1.29373841372842));
#22966=CARTESIAN_POINT('Ctrl Pts',(1.50178230149776,-1.,1.29145022885181));
#22967=CARTESIAN_POINT('Ctrl Pts',(1.49618896881754,-1.,1.28911506584254));
#22968=CARTESIAN_POINT('Ctrl Pts',(1.4906522831278,-1.,1.2867467611644));
#22969=CARTESIAN_POINT('Ctrl Pts',(1.4851881711891,-1.,1.28435533880201));
#22970=CARTESIAN_POINT('Ctrl Pts',(1.47980070347095,-1.,1.28194158939517));
#22971=CARTESIAN_POINT('Ctrl Pts',(1.4744717526707,-1.,1.2794891824849));
#22972=CARTESIAN_POINT('Ctrl Pts',(1.46916035917133,-1.,1.2769641483109));
#22973=CARTESIAN_POINT('Ctrl Pts',(1.46382431332476,-1.,1.27433119897822));
#22974=CARTESIAN_POINT('Ctrl Pts',(1.45843906294697,-1.,1.27156805265289));
#22975=CARTESIAN_POINT('Ctrl Pts',(1.45301422764247,-1.,1.2686778680489));
#22976=CARTESIAN_POINT('Ctrl Pts',(1.44761985001662,-1.,1.26570925118868));
#22977=CARTESIAN_POINT('Ctrl Pts',(1.44236470511303,-1.,1.26273903323859));
#22978=CARTESIAN_POINT('Ctrl Pts',(1.43734919180847,-1.,1.25983531012005));
#22979=CARTESIAN_POINT('Ctrl Pts',(1.43262645609691,-1.,1.25702687965755));
#22980=CARTESIAN_POINT('Ctrl Pts',(1.42815938799387,-1.,1.25426945222639));
#22981=CARTESIAN_POINT('Ctrl Pts',(1.42378102115575,-1.,1.2514145557001));
#22982=CARTESIAN_POINT('Ctrl Pts',(1.41923722596025,-1.,1.24824430986571));
#22983=CARTESIAN_POINT('Ctrl Pts',(1.41422913175179,-1.,1.24450600513056));
#22984=CARTESIAN_POINT('Ctrl Pts',(1.40845295531283,-1.,1.23994455029534));
#22985=CARTESIAN_POINT('Ctrl Pts',(1.40164708206106,-1.,1.23434087290423));
#22986=CARTESIAN_POINT('Ctrl Pts',(1.39361389568796,-1.,1.22752961899387));
#22987=CARTESIAN_POINT('Ctrl Pts',(1.38420564527715,-1.,1.21938737280852));
#22988=CARTESIAN_POINT('Ctrl Pts',(1.37331915607905,-1.,1.20982812925645));
#22989=CARTESIAN_POINT('Ctrl Pts',(1.36088705043885,-1.,1.1987959077932));
#22990=CARTESIAN_POINT('Ctrl Pts',(1.34687054001093,-1.,1.18625865667441));
#22991=CARTESIAN_POINT('Ctrl Pts',(1.33437539347008,-1.,1.17501305789857));
#22992=CARTESIAN_POINT('Ctrl Pts',(1.32428080721772,-1.,1.16589330093588));
#22993=CARTESIAN_POINT('Ctrl Pts',(1.31722977216397,-1.,1.15950888730809));
#22994=CARTESIAN_POINT('Ctrl Pts',(1.31362392696032,-1.,1.15624053661742));
#22995=CARTESIAN_POINT('',(1.15624053661742,-1.,1.31362392696033));
#22996=CARTESIAN_POINT('Origin',(0.,-1.,0.));
#22997=CARTESIAN_POINT('',(1.34869019493419,-1.,1.73811241238545));
#22998=CARTESIAN_POINT('Ctrl Pts',(1.15624053661742,-1.,1.31362392696033));
#22999=CARTESIAN_POINT('Ctrl Pts',(1.15950888730433,-1.,1.3172297721596));
#23000=CARTESIAN_POINT('Ctrl Pts',(1.16589330092532,-1.,1.32428080720544));
#23001=CARTESIAN_POINT('Ctrl Pts',(1.17501305787994,-1.,1.33437539344842));
#23002=CARTESIAN_POINT('Ctrl Pts',(1.18625865664915,-1.,1.34687053998157));
#23003=CARTESIAN_POINT('Ctrl Pts',(1.1987959077656,-1.,1.36088705040677));
#23004=CARTESIAN_POINT('Ctrl Pts',(1.20982812923113,-1.,1.37331915604962));
#23005=CARTESIAN_POINT('Ctrl Pts',(1.21938737278853,-1.,1.38420564525391));
#23006=CARTESIAN_POINT('Ctrl Pts',(1.22752961898063,-1.,1.39361389567257));
#23007=CARTESIAN_POINT('Ctrl Pts',(1.23434087289768,-1.,1.40164708205345));
#23008=CARTESIAN_POINT('Ctrl Pts',(1.23994455029421,-1.,1.40845295531151));
#23009=CARTESIAN_POINT('Ctrl Pts',(1.24450600513278,-1.,1.41422913175437));
#23010=CARTESIAN_POINT('Ctrl Pts',(1.24824430986911,-1.,1.41923722596421));
#23011=CARTESIAN_POINT('Ctrl Pts',(1.25141455570299,-1.,1.42378102115911));
#23012=CARTESIAN_POINT('Ctrl Pts',(1.25426945222783,-1.,1.42815938799555));
#23013=CARTESIAN_POINT('Ctrl Pts',(1.25702687965744,-1.,1.43262645609679));
#23014=CARTESIAN_POINT('Ctrl Pts',(1.25983531011894,-1.,1.43734919180719));
#23015=CARTESIAN_POINT('Ctrl Pts',(1.26273903323723,-1.,1.44236470511145));
#23016=CARTESIAN_POINT('Ctrl Pts',(1.26570925118767,-1.,1.44761985001544));
#23017=CARTESIAN_POINT('Ctrl Pts',(1.26867786804854,-1.,1.45301422764205));
#23018=CARTESIAN_POINT('Ctrl Pts',(1.27156805265312,-1.,1.45843906294725));
#23019=CARTESIAN_POINT('Ctrl Pts',(1.27433119897877,-1.,1.4638243133254));
#23020=CARTESIAN_POINT('Ctrl Pts',(1.27696414831144,-1.,1.46916035917197));
#23021=CARTESIAN_POINT('Ctrl Pts',(1.27948918248524,-1.,1.4744717526711));
#23022=CARTESIAN_POINT('Ctrl Pts',(1.28194158939522,-1.,1.47980070347102));
#23023=CARTESIAN_POINT('Ctrl Pts',(1.28435533880184,-1.,1.48518817118891));
#23024=CARTESIAN_POINT('Ctrl Pts',(1.28674676116415,-1.,1.4906522831275));
#23025=CARTESIAN_POINT('Ctrl Pts',(1.28911506584232,-1.,1.49618896881729));
#23026=CARTESIAN_POINT('Ctrl Pts',(1.29145022885171,-1.,1.50178230149764));
#23027=CARTESIAN_POINT('Ctrl Pts',(1.29373841372843,-1.,1.50741159078367));
#23028=CARTESIAN_POINT('Ctrl Pts',(1.29596850710518,-1.,1.51305994241412));
#23029=CARTESIAN_POINT('Ctrl Pts',(1.29813791800757,-1.,1.51872184912735));
#23030=CARTESIAN_POINT('Ctrl Pts',(1.30024984366334,-1.,1.5243995786107));
#23031=CARTESIAN_POINT('Ctrl Pts',(1.3023106439557,-1.,1.53009970283893));
#23032=CARTESIAN_POINT('Ctrl Pts',(1.30432735639487,-1.,1.53582981268976));
#23033=CARTESIAN_POINT('Ctrl Pts',(1.30630475189553,-1.,1.54159462645428));
#23034=CARTESIAN_POINT('Ctrl Pts',(1.30824393907471,-1.,1.54739413957183));
#23035=CARTESIAN_POINT('Ctrl Pts',(1.31014393684221,-1.,1.55322568759481));
#23036=CARTESIAN_POINT('Ctrl Pts',(1.31200264341696,-1.,1.55908521254822));
#23037=CARTESIAN_POINT('Ctrl Pts',(1.31381795281002,-1.,1.56496872402352));
#23038=CARTESIAN_POINT('Ctrl Pts',(1.31558903860015,-1.,1.57087397835721));
#23039=CARTESIAN_POINT('Ctrl Pts',(1.31731642317183,-1.,1.57680056505585));
#23040=CARTESIAN_POINT('Ctrl Pts',(1.31900135021428,-1.,1.58274907898829));
#23041=CARTESIAN_POINT('Ctrl Pts',(1.32064537110891,-1.,1.58872057258244));
#23042=CARTESIAN_POINT('Ctrl Pts',(1.32224985747686,-1.,1.59471591079408));
#23043=CARTESIAN_POINT('Ctrl Pts',(1.32381550858266,-1.,1.600735118587));
#23044=CARTESIAN_POINT('Ctrl Pts',(1.32534250785794,-1.,1.6067775829097));
#23045=CARTESIAN_POINT('Ctrl Pts',(1.32683074483365,-1.,1.61284234015762));
#23046=CARTESIAN_POINT('Ctrl Pts',(1.32828000610448,-1.,1.61892832270723));
#23047=CARTESIAN_POINT('Ctrl Pts',(1.32969019505665,-1.,1.62503464209777));
#23048=CARTESIAN_POINT('Ctrl Pts',(1.33106149345618,-1.,1.63116079730887));
#23049=CARTESIAN_POINT('Ctrl Pts',(1.33239425103694,-1.,1.6373065347505));
#23050=CARTESIAN_POINT('Ctrl Pts',(1.33368890676554,-1.,1.64347174856007));
#23051=CARTESIAN_POINT('Ctrl Pts',(1.33494590468003,-1.,1.64965637286843));
#23052=CARTESIAN_POINT('Ctrl Pts',(1.33616559745217,-1.,1.65586025952651));
#23053=CARTESIAN_POINT('Ctrl Pts',(1.33734820885331,-1.,1.66208312542073));
#23054=CARTESIAN_POINT('Ctrl Pts',(1.33849388654458,-1.,1.66832460784078));
#23055=CARTESIAN_POINT('Ctrl Pts',(1.33960273470372,-1.,1.67458429426126));
#23056=CARTESIAN_POINT('Ctrl Pts',(1.3406748518516,-1.,1.68086176030308));
#23057=CARTESIAN_POINT('Ctrl Pts',(1.34171037484673,-1.,1.68715660868602));
#23058=CARTESIAN_POINT('Ctrl Pts',(1.34270948206139,-1.,1.6934684849664));
#23059=CARTESIAN_POINT('Ctrl Pts',(1.34367237124322,-1.,1.69979707754221));
#23060=CARTESIAN_POINT('Ctrl Pts',(1.34459924533783,-1.,1.70614212266676));
#23061=CARTESIAN_POINT('Ctrl Pts',(1.34549029589563,-1.,1.71250340687011));
#23062=CARTESIAN_POINT('Ctrl Pts',(1.34634568653586,-1.,1.7188807715095));
#23063=CARTESIAN_POINT('Ctrl Pts',(1.34716554820013,-1.,1.72527410681298));
#23064=CARTESIAN_POINT('Ctrl Pts',(1.3477930915247,-1.,1.73040149654497));
#23065=CARTESIAN_POINT('Ctrl Pts',(1.34824783113158,-1.,1.73425417886255));
#23066=CARTESIAN_POINT('Ctrl Pts',(1.34854391898145,-1.,1.73682580585819));
#23067=CARTESIAN_POINT('Ctrl Pts',(1.34869019493419,-1.,1.73811241238545));
#23068=CARTESIAN_POINT('',(1.23627494547115,-1.,1.81978687191668));
#23069=CARTESIAN_POINT('',(1.34869019493419,-1.,1.73811241238545));
#23070=CARTESIAN_POINT('',(0.892032620296855,-1.,1.5055822144029));
#23071=CARTESIAN_POINT('Ctrl Pts',(1.23627494547115,-1.,1.81978687191668));
#23072=CARTESIAN_POINT('Ctrl Pts',(1.23509651170384,-1.,1.81925017193531));
#23073=CARTESIAN_POINT('Ctrl Pts',(1.23274224526804,-1.,1.81817389920914));
#23074=CARTESIAN_POINT('Ctrl Pts',(1.22921864890975,-1.,1.81655087183054));
#23075=CARTESIAN_POINT('Ctrl Pts',(1.22453613304507,-1.,1.81436959209778));
#23076=CARTESIAN_POINT('Ctrl Pts',(1.2187090610323,-1.,1.81161420806172));
#23077=CARTESIAN_POINT('Ctrl Pts',(1.2129081570818,-1.,1.80882996916931));
#23078=CARTESIAN_POINT('Ctrl Pts',(1.20713356605519,-1.,1.80601678480772));
#23079=CARTESIAN_POINT('Ctrl Pts',(1.2013854893912,-1.,1.8031745483882));
#23080=CARTESIAN_POINT('Ctrl Pts',(1.19566418930405,-1.,1.80030314370121));
#23081=CARTESIAN_POINT('Ctrl Pts',(1.1899699793456,-1.,1.79740245923649));
#23082=CARTESIAN_POINT('Ctrl Pts',(1.18430321697471,-1.,1.79447240321572));
#23083=CARTESIAN_POINT('Ctrl Pts',(1.17866429440781,-1.,1.79151291552646));
#23084=CARTESIAN_POINT('Ctrl Pts',(1.17305363177265,-1.,1.78852398877523));
#23085=CARTESIAN_POINT('Ctrl Pts',(1.16747166312239,-1.,1.78550566040349));
#23086=CARTESIAN_POINT('Ctrl Pts',(1.16191881298458,-1.,1.78245795880949));
#23087=CARTESIAN_POINT('Ctrl Pts',(1.15639547194689,-1.,1.77938085564261));
#23088=CARTESIAN_POINT('Ctrl Pts',(1.15090197841531,-1.,1.77627422557034));
#23089=CARTESIAN_POINT('Ctrl Pts',(1.14543858226948,-1.,1.77313777896234));
#23090=CARTESIAN_POINT('Ctrl Pts',(1.14000548337,-1.,1.76997111386806));
#23091=CARTESIAN_POINT('Ctrl Pts',(1.13460291804634,-1.,1.76677384551883));
#23092=CARTESIAN_POINT('Ctrl Pts',(1.12923123555076,-1.,1.76354571966171));
#23093=CARTESIAN_POINT('Ctrl Pts',(1.12389096855078,-1.,1.76028671825084));
#23094=CARTESIAN_POINT('Ctrl Pts',(1.11858293216752,-1.,1.75699720772089));
#23095=CARTESIAN_POINT('Ctrl Pts',(1.11330807582542,-1.,1.75367772094617));
#23096=CARTESIAN_POINT('Ctrl Pts',(1.10806728183003,-1.,1.75032866075914));
#23097=CARTESIAN_POINT('Ctrl Pts',(1.10286118991144,-1.,1.74695004214924));
#23098=CARTESIAN_POINT('Ctrl Pts',(1.09768999241229,-1.,1.74354119236212));
#23099=CARTESIAN_POINT('Ctrl Pts',(1.09255329056496,-1.,1.74010053962252));
#23100=CARTESIAN_POINT('Ctrl Pts',(1.08745056285429,-1.,1.73662628326093));
#23101=CARTESIAN_POINT('Ctrl Pts',(1.08238162784749,-1.,1.73311705663407));
#23102=CARTESIAN_POINT('Ctrl Pts',(1.0773470373727,-1.,1.72957248977424));
#23103=CARTESIAN_POINT('Ctrl Pts',(1.07234866990252,-1.,1.72599406198489));
#23104=CARTESIAN_POINT('Ctrl Pts',(1.06738966975463,-1.,1.72238500928456));
#23105=CARTESIAN_POINT('Ctrl Pts',(1.06247324680649,-1.,1.71874858456908));
#23106=CARTESIAN_POINT('Ctrl Pts',(1.05760163192481,-1.,1.71508654427022));
#23107=CARTESIAN_POINT('Ctrl Pts',(1.05277517202853,-1.,1.71139783543986));
#23108=CARTESIAN_POINT('Ctrl Pts',(1.0479908540499,-1.,1.70767646263641));
#23109=CARTESIAN_POINT('Ctrl Pts',(1.04324363334546,-1.,1.70391338707969));
#23110=CARTESIAN_POINT('Ctrl Pts',(1.03852922490782,-1.,1.70010052930951));
#23111=CARTESIAN_POINT('Ctrl Pts',(1.03384646003587,-1.,1.69623414782769));
#23112=CARTESIAN_POINT('Ctrl Pts',(1.02919977579155,-1.,1.69231840863471));
#23113=CARTESIAN_POINT('Ctrl Pts',(1.02460180535272,-1.,1.68836910178475));
#23114=CARTESIAN_POINT('Ctrl Pts',(1.02006795074222,-1.,1.68440578021739));
#23115=CARTESIAN_POINT('Ctrl Pts',(1.01561026162786,-1.,1.6804428989482));
#23116=CARTESIAN_POINT('Ctrl Pts',(1.01123236493507,-1.,1.67648246776457));
#23117=CARTESIAN_POINT('Ctrl Pts',(1.00692206696387,-1.,1.67250335383248));
#23118=CARTESIAN_POINT('Ctrl Pts',(1.00265091003682,-1.,1.66846059277231));
#23119=CARTESIAN_POINT('Ctrl Pts',(0.998389654952317,-1.,1.66430758030304));
#23120=CARTESIAN_POINT('Ctrl Pts',(0.994121836661115,-1.,1.66001553809916));
#23121=CARTESIAN_POINT('Ctrl Pts',(0.98985562785445,-1.,1.65559044289746));
#23122=CARTESIAN_POINT('Ctrl Pts',(0.985642622921626,-1.,1.6511001661277));
#23123=CARTESIAN_POINT('Ctrl Pts',(0.981562530940574,-1.,1.64665139190834));
#23124=CARTESIAN_POINT('Ctrl Pts',(0.977689794120296,-1.,1.64233990826831));
#23125=CARTESIAN_POINT('Ctrl Pts',(0.974066058287501,-1.,1.63820952658157));
#23126=CARTESIAN_POINT('Ctrl Pts',(0.970669715996356,-1.,1.63420665729609));
#23127=CARTESIAN_POINT('Ctrl Pts',(0.967387853228041,-1.,1.63013849959083));
#23128=CARTESIAN_POINT('Ctrl Pts',(0.964046107037821,-1.,1.6257193066974));
#23129=CARTESIAN_POINT('Ctrl Pts',(0.960438326099958,-1.,1.62061638139929));
#23130=CARTESIAN_POINT('Ctrl Pts',(0.956354422921572,-1.,1.61449324337233));
#23131=CARTESIAN_POINT('Ctrl Pts',(0.951613284361247,-1.,1.60706069897794));
#23132=CARTESIAN_POINT('Ctrl Pts',(0.946078063325795,-1.,1.59810042045408));
#23133=CARTESIAN_POINT('Ctrl Pts',(0.939646377909319,-1.,1.58744937489796));
#23134=CARTESIAN_POINT('Ctrl Pts',(0.932246680128848,-1.,1.57499388385561));
#23135=CARTESIAN_POINT('Ctrl Pts',(0.923832188966322,-1.,1.56065988582509));
#23136=CARTESIAN_POINT('Ctrl Pts',(0.914375919046579,-1.,1.54440491152808));
#23137=CARTESIAN_POINT('Ctrl Pts',(0.905967409640498,-1.,1.52984849890434));
#23138=CARTESIAN_POINT('Ctrl Pts',(0.89918504749193,-1.,1.51805569591479));
#23139=CARTESIAN_POINT('Ctrl Pts',(0.894452006967538,-1.,1.50980486807181));
#23140=CARTESIAN_POINT('Ctrl Pts',(0.892032620296855,-1.,1.5055822144029));
#23141=CARTESIAN_POINT('',(0.693717979106305,-1.,1.60662857109684));
#23142=CARTESIAN_POINT('Origin',(0.,-1.,0.));
#23143=CARTESIAN_POINT('',(0.7455743247944,-1.,2.0698113262342));
#23144=CARTESIAN_POINT('Ctrl Pts',(0.693717979106305,-1.,1.60662857109684));
#23145=CARTESIAN_POINT('Ctrl Pts',(0.69571209787897,-1.,1.61106790957619));
#23146=CARTESIAN_POINT('Ctrl Pts',(0.699605146398836,-1.,1.61974673471117));
#23147=CARTESIAN_POINT('Ctrl Pts',(0.705159151977294,-1.,1.6321654166204));
#23148=CARTESIAN_POINT('Ctrl Pts',(0.711993139340447,-1.,1.64752408828442));
#23149=CARTESIAN_POINT('Ctrl Pts',(0.719585433787949,-1.,1.66472880551777));
#23150=CARTESIAN_POINT('Ctrl Pts',(0.726235967982445,-1.,1.67996158451922));
#23151=CARTESIAN_POINT('Ctrl Pts',(0.731963238685357,-1.,1.69326921972915));
#23152=CARTESIAN_POINT('Ctrl Pts',(0.736799665716932,-1.,1.70473309004249));
#23153=CARTESIAN_POINT('Ctrl Pts',(0.74079516202821,-1.,1.71447789751001));
#23154=CARTESIAN_POINT('Ctrl Pts',(0.744021445433093,-1.,1.72268229916769));
#23155=CARTESIAN_POINT('Ctrl Pts',(0.746574710097752,-1.,1.72958533647714));
#23156=CARTESIAN_POINT('Ctrl Pts',(0.74858246295687,-1.,1.7355035168033));
#23157=CARTESIAN_POINT('Ctrl Pts',(0.750193435981249,-1.,1.74080458267114));
#23158=CARTESIAN_POINT('Ctrl Pts',(0.751555614164482,-1.,1.74585086852502));
#23159=CARTESIAN_POINT('Ctrl Pts',(0.752797683531314,-1.,1.75095139468794));
#23160=CARTESIAN_POINT('Ctrl Pts',(0.754009254027828,-1.,1.75631083600019));
#23161=CARTESIAN_POINT('Ctrl Pts',(0.755220979974461,-1.,1.76197817240128));
#23162=CARTESIAN_POINT('Ctrl Pts',(0.75642189602781,-1.,1.76789396002998));
#23163=CARTESIAN_POINT('Ctrl Pts',(0.757578264077028,-1.,1.77394167108292));
#23164=CARTESIAN_POINT('Ctrl Pts',(0.758650626677518,-1.,1.77999411220945));
#23165=CARTESIAN_POINT('Ctrl Pts',(0.759614401110189,-1.,1.78596964884604));
#23166=CARTESIAN_POINT('Ctrl Pts',(0.760469555880749,-1.,1.7918581561088));
#23167=CARTESIAN_POINT('Ctrl Pts',(0.761229695230558,-1.,1.79768986997783));
#23168=CARTESIAN_POINT('Ctrl Pts',(0.761915336443547,-1.,1.80351583877342));
#23169=CARTESIAN_POINT('Ctrl Pts',(0.762546129463938,-1.,1.80938551463965));
#23170=CARTESIAN_POINT('Ctrl Pts',(0.763132003836634,-1.,1.8153211840553));
#23171=CARTESIAN_POINT('Ctrl Pts',(0.763673465462726,-1.,1.82131873145266));
#23172=CARTESIAN_POINT('Ctrl Pts',(0.764165902605995,-1.,1.82735991200065));
#23173=CARTESIAN_POINT('Ctrl Pts',(0.764602549687853,-1.,1.83342077227142));
#23174=CARTESIAN_POINT('Ctrl Pts',(0.764978057881737,-1.,1.83948181064835));
#23175=CARTESIAN_POINT('Ctrl Pts',(0.765291664862029,-1.,1.84553698875924));
#23176=CARTESIAN_POINT('Ctrl Pts',(0.765545710619062,-1.,1.85158945130063));
#23177=CARTESIAN_POINT('Ctrl Pts',(0.765744212909318,-1.,1.85764741390394));
#23178=CARTESIAN_POINT('Ctrl Pts',(0.765891519092547,-1.,1.86372027063312));
#23179=CARTESIAN_POINT('Ctrl Pts',(0.765990708546091,-1.,1.86981398314341));
#23180=CARTESIAN_POINT('Ctrl Pts',(0.766042837036744,-1.,1.87592888967883));
#23181=CARTESIAN_POINT('Ctrl Pts',(0.766047794851864,-1.,1.88206215302561));
#23182=CARTESIAN_POINT('Ctrl Pts',(0.766004837062091,-1.,1.88820926433409));
#23183=CARTESIAN_POINT('Ctrl Pts',(0.765913193856978,-1.,1.89436577771388));
#23184=CARTESIAN_POINT('Ctrl Pts',(0.765772772593386,-1.,1.90052930393596));
#23185=CARTESIAN_POINT('Ctrl Pts',(0.765584196937919,-1.,1.90669961402356));
#23186=CARTESIAN_POINT('Ctrl Pts',(0.765348465884722,-1.,1.91287765805169));
#23187=CARTESIAN_POINT('Ctrl Pts',(0.765066729667088,-1.,1.91906491634196));
#23188=CARTESIAN_POINT('Ctrl Pts',(0.764740025488211,-1.,1.92526263537048));
#23189=CARTESIAN_POINT('Ctrl Pts',(0.76436901067394,-1.,1.93147105496382));
#23190=CARTESIAN_POINT('Ctrl Pts',(0.763954049121458,-1.,1.93768964875886));
#23191=CARTESIAN_POINT('Ctrl Pts',(0.763495333538629,-1.,1.9439174661764));
#23192=CARTESIAN_POINT('Ctrl Pts',(0.762992990878769,-1.,1.95015342590024));
#23193=CARTESIAN_POINT('Ctrl Pts',(0.762447203806178,-1.,1.95639665309869));
#23194=CARTESIAN_POINT('Ctrl Pts',(0.761858300014423,-1.,1.96264672744186));
#23195=CARTESIAN_POINT('Ctrl Pts',(0.76122669048382,-1.,1.96890351582499));
#23196=CARTESIAN_POINT('Ctrl Pts',(0.760552825409757,-1.,1.97516705321494));
#23197=CARTESIAN_POINT('Ctrl Pts',(0.75983714745219,-1.,1.98143741418172));
#23198=CARTESIAN_POINT('Ctrl Pts',(0.759080037802488,-1.,1.98771456680874));
#23199=CARTESIAN_POINT('Ctrl Pts',(0.758281796766761,-1.,1.99399831098817));
#23200=CARTESIAN_POINT('Ctrl Pts',(0.757442676862724,-1.,2.00028834739178));
#23201=CARTESIAN_POINT('Ctrl Pts',(0.75656290464667,-1.,2.0065843158773));
#23202=CARTESIAN_POINT('Ctrl Pts',(0.755642704957865,-1.,2.01288584328084));
#23203=CARTESIAN_POINT('Ctrl Pts',(0.754682330722816,-1.,2.01919259405809));
#23204=CARTESIAN_POINT('Ctrl Pts',(0.753682061112768,-1.,2.02550428623313));
#23205=CARTESIAN_POINT('Ctrl Pts',(0.75264218048721,-1.,2.03182068456221));
#23206=CARTESIAN_POINT('Ctrl Pts',(0.751562963361115,-1.,2.03814160092099));
#23207=CARTESIAN_POINT('Ctrl Pts',(0.750444657875575,-1.,2.04446689147979));
#23208=CARTESIAN_POINT('Ctrl Pts',(0.749287468665046,-1.,2.05079645592154));
#23209=CARTESIAN_POINT('Ctrl Pts',(0.748091554183802,-1.,2.05713023031007));
#23210=CARTESIAN_POINT('Ctrl Pts',(0.747103932787919,-1.,2.06220058927826));
#23211=CARTESIAN_POINT('Ctrl Pts',(0.7463458715442,-1.,2.06600523016815));
#23212=CARTESIAN_POINT('Ctrl Pts',(0.745832791378367,-1.,2.06854248895728));
#23213=CARTESIAN_POINT('Ctrl Pts',(0.7455743247944,-1.,2.0698113262342));
#23214=CARTESIAN_POINT('',(0.61342227326009,-1.,2.11275013067528));
#23215=CARTESIAN_POINT('',(0.7455743247944,-1.,2.0698113262342));
#23216=CARTESIAN_POINT('',(0.383122945602004,-1.,1.7075470150345));
#23217=CARTESIAN_POINT('Ctrl Pts',(0.61342227326009,-1.,2.11275013067528));
#23218=CARTESIAN_POINT('Ctrl Pts',(0.6124673655618,-1.,2.11187554259986));
#23219=CARTESIAN_POINT('Ctrl Pts',(0.610560911689898,-1.,2.11012443807238));
#23220=CARTESIAN_POINT('Ctrl Pts',(0.607711315454876,-1.,2.1074919961518));
#23221=CARTESIAN_POINT('Ctrl Pts',(0.60393203073603,-1.,2.10397049886949));
#23222=CARTESIAN_POINT('Ctrl Pts',(0.599241616420533,-1.,2.0995493086477));
#23223=CARTESIAN_POINT('Ctrl Pts',(0.594585006052162,-1.,2.0951087622027));
#23224=CARTESIAN_POINT('Ctrl Pts',(0.589962365403406,-1.,2.09064881812129));
#23225=CARTESIAN_POINT('Ctrl Pts',(0.585373918991617,-1.,2.08616943727951));
#23226=CARTESIAN_POINT('Ctrl Pts',(0.580819952108063,-1.,2.08167059018418));
#23227=CARTESIAN_POINT('Ctrl Pts',(0.576300797416844,-1.,2.07715226767559));
#23228=CARTESIAN_POINT('Ctrl Pts',(0.571816823242602,-1.,2.07261449292824));
#23229=CARTESIAN_POINT('Ctrl Pts',(0.567368421181087,-1.,2.06805732997334));
#23230=CARTESIAN_POINT('Ctrl Pts',(0.562955993082261,-1.,2.06348090160589));
#23231=CARTESIAN_POINT('Ctrl Pts',(0.558579940185151,-1.,2.05888537756462));
#23232=CARTESIAN_POINT('Ctrl Pts',(0.554240657463906,-1.,2.05427091604413));
#23233=CARTESIAN_POINT('Ctrl Pts',(0.549938525150295,-1.,2.04963761077958));
#23234=CARTESIAN_POINT('Ctrl Pts',(0.54567390381743,-1.,2.04498544714588));
#23235=CARTESIAN_POINT('Ctrl Pts',(0.541447120615659,-1.,2.04031422690527));
#23236=CARTESIAN_POINT('Ctrl Pts',(0.537258489833262,-1.,2.03562362954037));
#23237=CARTESIAN_POINT('Ctrl Pts',(0.533108355132976,-1.,2.03091336214426));
#23238=CARTESIAN_POINT('Ctrl Pts',(0.528997127241914,-1.,2.0261832908329));
#23239=CARTESIAN_POINT('Ctrl Pts',(0.524925318333476,-1.,2.02143356304698));
#23240=CARTESIAN_POINT('Ctrl Pts',(0.52089359039937,-1.,2.01666477917286));
#23241=CARTESIAN_POINT('Ctrl Pts',(0.516902681728687,-1.,2.01187773939242));
#23242=CARTESIAN_POINT('Ctrl Pts',(0.512953306961792,-1.,2.00707309946949));
#23243=CARTESIAN_POINT('Ctrl Pts',(0.509046069886157,-1.,2.00225107134734));
#23244=CARTESIAN_POINT('Ctrl Pts',(0.505181361323026,-1.,1.99741107463572));
#23245=CARTESIAN_POINT('Ctrl Pts',(0.501359287727146,-1.,1.99255149126155));
#23246=CARTESIAN_POINT('Ctrl Pts',(0.497579909545574,-1.,1.98767044752932));
#23247=CARTESIAN_POINT('Ctrl Pts',(0.493843476541494,-1.,1.98276658761821));
#23248=CARTESIAN_POINT('Ctrl Pts',(0.490150627860952,-1.,1.97783973019229));
#23249=CARTESIAN_POINT('Ctrl Pts',(0.486502692907658,-1.,1.97289186263272));
#23250=CARTESIAN_POINT('Ctrl Pts',(0.48290166212069,-1.,1.96792703422362));
#23251=CARTESIAN_POINT('Ctrl Pts',(0.479349583074855,-1.,1.96294933055943));
#23252=CARTESIAN_POINT('Ctrl Pts',(0.475848034683176,-1.,1.95796111148177));
#23253=CARTESIAN_POINT('Ctrl Pts',(0.472397672264072,-1.,1.95296148278133));
#23254=CARTESIAN_POINT('Ctrl Pts',(0.468997482913135,-1.,1.94794381136514));
#23255=CARTESIAN_POINT('Ctrl Pts',(0.46564546202603,-1.,1.9428979419619));
#23256=CARTESIAN_POINT('Ctrl Pts',(0.462340031009056,-1.,1.93781486640821));
#23257=CARTESIAN_POINT('Ctrl Pts',(0.459081234547926,-1.,1.93269066517934));
#23258=CARTESIAN_POINT('Ctrl Pts',(0.45587200517437,-1.,1.92753067150476));
#23259=CARTESIAN_POINT('Ctrl Pts',(0.452719478359432,-1.,1.92235380648502));
#23260=CARTESIAN_POINT('Ctrl Pts',(0.449632260106662,-1.,1.91718342555755));
#23261=CARTESIAN_POINT('Ctrl Pts',(0.446617343485711,-1.,1.9120369998112));
#23262=CARTESIAN_POINT('Ctrl Pts',(0.44367755684915,-1.,1.90691756144898));
#23263=CARTESIAN_POINT('Ctrl Pts',(0.440807833704038,-1.,1.90180124389086));
#23264=CARTESIAN_POINT('Ctrl Pts',(0.437995003948244,-1.,1.89663648956466));
#23265=CARTESIAN_POINT('Ctrl Pts',(0.435225660963383,-1.,1.89136993975504));
#23266=CARTESIAN_POINT('Ctrl Pts',(0.432493038548748,-1.,1.88596913666793));
#23267=CARTESIAN_POINT('Ctrl Pts',(0.429803062482344,-1.,1.88044229001832));
#23268=CARTESIAN_POINT('Ctrl Pts',(0.427183828519102,-1.,1.87486989291484));
#23269=CARTESIAN_POINT('Ctrl Pts',(0.424678177291358,-1.,1.86937803944323));
#23270=CARTESIAN_POINT('Ctrl Pts',(0.422327307418275,-1.,1.86408083334028));
#23271=CARTESIAN_POINT('Ctrl Pts',(0.420157287975619,-1.,1.85903281096686));
#23272=CARTESIAN_POINT('Ctrl Pts',(0.418164129143534,-1.,1.85417632856234));
#23273=CARTESIAN_POINT('Ctrl Pts',(0.416300022038864,-1.,1.84929312929882));
#23274=CARTESIAN_POINT('Ctrl Pts',(0.41448743825434,-1.,1.8440575707371));
#23275=CARTESIAN_POINT('Ctrl Pts',(0.412633125322161,-1.,1.83808953475839));
#23276=CARTESIAN_POINT('Ctrl Pts',(0.410641256301674,-1.,1.83100408895216));
#23277=CARTESIAN_POINT('Ctrl Pts',(0.408428948108533,-1.,1.8224702267854));
#23278=CARTESIAN_POINT('Ctrl Pts',(0.405933518411838,-1.,1.81223801813988));
#23279=CARTESIAN_POINT('Ctrl Pts',(0.403107976170441,-1.,1.80012077176221));
#23280=CARTESIAN_POINT('Ctrl Pts',(0.39991940378308,-1.,1.78598826347533));
#23281=CARTESIAN_POINT('Ctrl Pts',(0.39634619612042,-1.,1.7697556004756));
#23282=CARTESIAN_POINT('Ctrl Pts',(0.392375812294307,-1.,1.75137405313962));
#23283=CARTESIAN_POINT('Ctrl Pts',(0.388877023509191,-1.,1.7349317097561));
#23284=CARTESIAN_POINT('Ctrl Pts',(0.38607079032701,-1.,1.72162022246158));
#23285=CARTESIAN_POINT('Ctrl Pts',(0.384119047315541,-1.,1.71231062891958));
#23286=CARTESIAN_POINT('Ctrl Pts',(0.383122945602004,-1.,1.7075470150345));
#23287=CARTESIAN_POINT('',(0.163289472382896,-1.,1.74236521665491));
#23288=CARTESIAN_POINT('Origin',(0.,-1.,0.));
#23289=CARTESIAN_POINT('',(0.0694764450219578,-1.,2.19890268624765));
#23290=CARTESIAN_POINT('Ctrl Pts',(0.163289472382896,-1.,1.74236521665491));
#23291=CARTESIAN_POINT('Ctrl Pts',(0.163814161002002,-1.,1.7472034950333));
#23292=CARTESIAN_POINT('Ctrl Pts',(0.164834765707158,-1.,1.75666056638427));
#23293=CARTESIAN_POINT('Ctrl Pts',(0.1662793551464,-1.,1.77018771684844));
#23294=CARTESIAN_POINT('Ctrl Pts',(0.168032772805197,-1.,1.7869064998507));
#23295=CARTESIAN_POINT('Ctrl Pts',(0.169936923904608,-1.,1.80561530629706));
#23296=CARTESIAN_POINT('Ctrl Pts',(0.171554770204119,-1.,1.82215766811545));
#23297=CARTESIAN_POINT('Ctrl Pts',(0.1728894428919,-1.,1.83658380527692));
#23298=CARTESIAN_POINT('Ctrl Pts',(0.173946627587731,-1.,1.8489811319852));
#23299=CARTESIAN_POINT('Ctrl Pts',(0.17473525927603,-1.,1.85948367088837));
#23300=CARTESIAN_POINT('Ctrl Pts',(0.175268337590757,-1.,1.86828349694799));
#23301=CARTESIAN_POINT('Ctrl Pts',(0.175563480746485,-1.,1.87563767773588));
#23302=CARTESIAN_POINT('Ctrl Pts',(0.175644148889698,-1.,1.88188663145367));
#23303=CARTESIAN_POINT('Ctrl Pts',(0.175538155840648,-1.,1.88742606273259));
#23304=CARTESIAN_POINT('Ctrl Pts',(0.175274276190844,-1.,1.892646301985));
#23305=CARTESIAN_POINT('Ctrl Pts',(0.174879405091263,-1.,1.89788101117132));
#23306=CARTESIAN_POINT('Ctrl Pts',(0.174375518661085,-1.,1.90335253862834));
#23307=CARTESIAN_POINT('Ctrl Pts',(0.173776635257816,-1.,1.90911693975267));
#23308=CARTESIAN_POINT('Ctrl Pts',(0.173090695383496,-1.,1.91511429159527));
#23309=CARTESIAN_POINT('Ctrl Pts',(0.172321621259513,-1.,1.9212233439798));
#23310=CARTESIAN_POINT('Ctrl Pts',(0.171471191532988,-1.,1.92731093582036));
#23311=CARTESIAN_POINT('Ctrl Pts',(0.170541253116201,-1.,1.93329183155539));
#23312=CARTESIAN_POINT('Ctrl Pts',(0.16953490481749,-1.,1.93915639211581));
#23313=CARTESIAN_POINT('Ctrl Pts',(0.168455741607556,-1.,1.94493757756931));
#23314=CARTESIAN_POINT('Ctrl Pts',(0.167307501784475,-1.,1.95069027794294));
#23315=CARTESIAN_POINT('Ctrl Pts',(0.166093592002812,-1.,1.9564675971873));
#23316=CARTESIAN_POINT('Ctrl Pts',(0.164816568920269,-1.,1.96229379940136));
#23317=CARTESIAN_POINT('Ctrl Pts',(0.163478185457734,-1.,1.96816512677967));
#23318=CARTESIAN_POINT('Ctrl Pts',(0.162079693556288,-1.,1.97406280235188));
#23319=CARTESIAN_POINT('Ctrl Pts',(0.160622060784611,-1.,1.97996195437559));
#23320=CARTESIAN_POINT('Ctrl Pts',(0.159106226437299,-1.,1.98584238283292));
#23321=CARTESIAN_POINT('Ctrl Pts',(0.157533331459227,-1.,1.99169810931908));
#23322=CARTESIAN_POINT('Ctrl Pts',(0.155904629548783,-1.,1.99753284771497));
#23323=CARTESIAN_POINT('Ctrl Pts',(0.154221403049722,-1.,2.00335565310543));
#23324=CARTESIAN_POINT('Ctrl Pts',(0.152484883621449,-1.,2.00917680318424));
#23325=CARTESIAN_POINT('Ctrl Pts',(0.150696157673078,-1.,2.01500291940238));
#23326=CARTESIAN_POINT('Ctrl Pts',(0.148856124775337,-1.,2.02083464969894));
#23327=CARTESIAN_POINT('Ctrl Pts',(0.146965557332583,-1.,2.02666926182017));
#23328=CARTESIAN_POINT('Ctrl Pts',(0.145025140186057,-1.,2.03250223739942));
#23329=CARTESIAN_POINT('Ctrl Pts',(0.143035515058208,-1.,2.03832911025912));
#23330=CARTESIAN_POINT('Ctrl Pts',(0.140997332152546,-1.,2.04414757947916));
#23331=CARTESIAN_POINT('Ctrl Pts',(0.138911255368966,-1.,2.04995762001328));
#23332=CARTESIAN_POINT('Ctrl Pts',(0.136777941218043,-1.,2.05576044414264));
#23333=CARTESIAN_POINT('Ctrl Pts',(0.134598026192106,-1.,2.06155781517842));
#23334=CARTESIAN_POINT('Ctrl Pts',(0.13237211154771,-1.,2.06735123910326));
#23335=CARTESIAN_POINT('Ctrl Pts',(0.130100748328403,-1.,2.07314114713063));
#23336=CARTESIAN_POINT('Ctrl Pts',(0.12778444527612,-1.,2.07892715110987));
#23337=CARTESIAN_POINT('Ctrl Pts',(0.125423679412061,-1.,2.08470840653643));
#23338=CARTESIAN_POINT('Ctrl Pts',(0.123018905621083,-1.,2.09048392424825));
#23339=CARTESIAN_POINT('Ctrl Pts',(0.120570567965122,-1.,2.0962529286773));
#23340=CARTESIAN_POINT('Ctrl Pts',(0.118079107988355,-1.,2.102015121329));
#23341=CARTESIAN_POINT('Ctrl Pts',(0.115544957687926,-1.,2.10777050261309));
#23342=CARTESIAN_POINT('Ctrl Pts',(0.112968534419737,-1.,2.11351924490306));
#23343=CARTESIAN_POINT('Ctrl Pts',(0.110350236135025,-1.,2.11926155590865));
#23344=CARTESIAN_POINT('Ctrl Pts',(0.10769043523109,-1.,2.12499752307));
#23345=CARTESIAN_POINT('Ctrl Pts',(0.104989479152739,-1.,2.13072704887293));
#23346=CARTESIAN_POINT('Ctrl Pts',(0.1022477005561,-1.,2.13644992667165));
#23347=CARTESIAN_POINT('Ctrl Pts',(0.0994654261990913,-1.,2.14216588396025));
#23348=CARTESIAN_POINT('Ctrl Pts',(0.0966429852305456,-1.,2.14787463531795));
#23349=CARTESIAN_POINT('Ctrl Pts',(0.0937807218867641,-1.,2.1535759397817));
#23350=CARTESIAN_POINT('Ctrl Pts',(0.0908789888107263,-1.,2.15926961544516));
#23351=CARTESIAN_POINT('Ctrl Pts',(0.087938129138692,-1.,2.16495552645014));
#23352=CARTESIAN_POINT('Ctrl Pts',(0.084958462083537,-1.,2.17063357870952));
#23353=CARTESIAN_POINT('Ctrl Pts',(0.0819402680872763,-1.,2.176303712113));
#23354=CARTESIAN_POINT('Ctrl Pts',(0.078883772768524,-1.,2.18196589448887));
#23355=CARTESIAN_POINT('Ctrl Pts',(0.0757891465836145,-1.,2.1876201139953));
#23356=CARTESIAN_POINT('Ctrl Pts',(0.0732830357306722,-1.,2.19213712013662));
#23357=CARTESIAN_POINT('Ctrl Pts',(0.0713863779526151,-1.,2.19552129484002));
#23358=CARTESIAN_POINT('Ctrl Pts',(0.0701143536325487,-1.,2.19777582085423));
#23359=CARTESIAN_POINT('Ctrl Pts',(0.0694764450219578,-1.,2.19890268624765));
#23360=CARTESIAN_POINT('',(-0.0694764450219586,-1.,2.19890268624765));
#23361=CARTESIAN_POINT('',(0.0694764450219578,-1.,2.19890268624765));
#23362=CARTESIAN_POINT('',(-0.163289472382896,-1.,1.74236521665491));
#23363=CARTESIAN_POINT('Ctrl Pts',(-0.0694764450219586,-1.,2.19890268624765));
#23364=CARTESIAN_POINT('Ctrl Pts',(-0.0701143536324929,-1.,2.19777582085261));
#23365=CARTESIAN_POINT('Ctrl Pts',(-0.071386377952463,-1.,2.19552129483562));
#23366=CARTESIAN_POINT('Ctrl Pts',(-0.0732830357304279,-1.,2.19213712012956));
#23367=CARTESIAN_POINT('Ctrl Pts',(-0.0757891465833414,-1.,2.1876201139874));
#23368=CARTESIAN_POINT('Ctrl Pts',(-0.078883772768323,-1.,2.18196589448304));
#23369=CARTESIAN_POINT('Ctrl Pts',(-0.0819402680871942,-1.,2.1763037121106));
#23370=CARTESIAN_POINT('Ctrl Pts',(-0.0849584620835646,-1.,2.17063357871031));
#23371=CARTESIAN_POINT('Ctrl Pts',(-0.0879381291387825,-1.,2.16495552645275));
#23372=CARTESIAN_POINT('Ctrl Pts',(-0.0908789888108269,-1.,2.15926961544808));
#23373=CARTESIAN_POINT('Ctrl Pts',(-0.0937807218868348,-1.,2.15357593978377));
#23374=CARTESIAN_POINT('Ctrl Pts',(-0.0966429852305691,-1.,2.14787463531864));
#23375=CARTESIAN_POINT('Ctrl Pts',(-0.0994654261990745,-1.,2.14216588395974));
#23376=CARTESIAN_POINT('Ctrl Pts',(-0.102247700556064,-1.,2.13644992667052));
#23377=CARTESIAN_POINT('Ctrl Pts',(-0.104989479152703,-1.,2.1307270488718));
#23378=CARTESIAN_POINT('Ctrl Pts',(-0.107690435231068,-1.,2.12499752306927));
#23379=CARTESIAN_POINT('Ctrl Pts',(-0.11035023613502,-1.,2.11926155590849));
#23380=CARTESIAN_POINT('Ctrl Pts',(-0.112968534419746,-1.,2.11351924490335));
#23381=CARTESIAN_POINT('Ctrl Pts',(-0.115544957687941,-1.,2.10777050261359));
#23382=CARTESIAN_POINT('Ctrl Pts',(-0.118079107988368,-1.,2.10201512132945));
#23383=CARTESIAN_POINT('Ctrl Pts',(-0.120570567965129,-1.,2.09625292867756));
#23384=CARTESIAN_POINT('Ctrl Pts',(-0.123018905621083,-1.,2.09048392424826));
#23385=CARTESIAN_POINT('Ctrl Pts',(-0.125423679412058,-1.,2.08470840653628));
#23386=CARTESIAN_POINT('Ctrl Pts',(-0.127784445276116,-1.,2.07892715110967));
#23387=CARTESIAN_POINT('Ctrl Pts',(-0.130100748328401,-1.,2.07314114713047));
#23388=CARTESIAN_POINT('Ctrl Pts',(-0.13237211154771,-1.,2.06735123910319));
#23389=CARTESIAN_POINT('Ctrl Pts',(-0.134598026192107,-1.,2.06155781517844));
#23390=CARTESIAN_POINT('Ctrl Pts',(-0.136777941218044,-1.,2.0557604441427));
#23391=CARTESIAN_POINT('Ctrl Pts',(-0.138911255368966,-1.,2.04995762001333));
#23392=CARTESIAN_POINT('Ctrl Pts',(-0.140997332152546,-1.,2.04414757947919));
#23393=CARTESIAN_POINT('Ctrl Pts',(-0.143035515058208,-1.,2.03832911025913));
#23394=CARTESIAN_POINT('Ctrl Pts',(-0.145025140186058,-1.,2.03250223739941));
#23395=CARTESIAN_POINT('Ctrl Pts',(-0.146965557332586,-1.,2.02666926182017));
#23396=CARTESIAN_POINT('Ctrl Pts',(-0.148856124775343,-1.,2.02083464969897));
#23397=CARTESIAN_POINT('Ctrl Pts',(-0.150696157673084,-1.,2.01500291940243));
#23398=CARTESIAN_POINT('Ctrl Pts',(-0.152484883621452,-1.,2.00917680318426));
#23399=CARTESIAN_POINT('Ctrl Pts',(-0.154221403049719,-1.,2.00335565310539));
#23400=CARTESIAN_POINT('Ctrl Pts',(-0.155904629548775,-1.,1.99753284771487));
#23401=CARTESIAN_POINT('Ctrl Pts',(-0.157533331459215,-1.,1.99169810931893));
#23402=CARTESIAN_POINT('Ctrl Pts',(-0.159106226437289,-1.,1.98584238283279));
#23403=CARTESIAN_POINT('Ctrl Pts',(-0.16062206078461,-1.,1.97996195437557));
#23404=CARTESIAN_POINT('Ctrl Pts',(-0.162079693556302,-1.,1.97406280235204));
#23405=CARTESIAN_POINT('Ctrl Pts',(-0.16347818545776,-1.,1.96816512678));
#23406=CARTESIAN_POINT('Ctrl Pts',(-0.1648165689203,-1.,1.96229379940174));
#23407=CARTESIAN_POINT('Ctrl Pts',(-0.166093592002833,-1.,1.95646759718755));
#23408=CARTESIAN_POINT('Ctrl Pts',(-0.167307501784469,-1.,1.95069027794286));
#23409=CARTESIAN_POINT('Ctrl Pts',(-0.168455741607516,-1.,1.94493757756879));
#23410=CARTESIAN_POINT('Ctrl Pts',(-0.169534904817425,-1.,1.93915639211497));
#23411=CARTESIAN_POINT('Ctrl Pts',(-0.170541253116136,-1.,1.93329183155455));
#23412=CARTESIAN_POINT('Ctrl Pts',(-0.17147119153296,-1.,1.92731093582));
#23413=CARTESIAN_POINT('Ctrl Pts',(-0.172321621259557,-1.,1.92122334398034));
#23414=CARTESIAN_POINT('Ctrl Pts',(-0.173090695383619,-1.,1.91511429159681));
#23415=CARTESIAN_POINT('Ctrl Pts',(-0.173776635257984,-1.,1.90911693975475));
#23416=CARTESIAN_POINT('Ctrl Pts',(-0.174375518661222,-1.,1.90335253863003));
#23417=CARTESIAN_POINT('Ctrl Pts',(-0.174879405091277,-1.,1.89788101117148));
#23418=CARTESIAN_POINT('Ctrl Pts',(-0.175274276190664,-1.,1.89264630198279));
#23419=CARTESIAN_POINT('Ctrl Pts',(-0.175538155840286,-1.,1.88742606272818));
#23420=CARTESIAN_POINT('Ctrl Pts',(-0.175644148889271,-1.,1.88188663144846));
#23421=CARTESIAN_POINT('Ctrl Pts',(-0.175563480746206,-1.,1.87563767773249));
#23422=CARTESIAN_POINT('Ctrl Pts',(-0.175268337590901,-1.,1.86828349694972));
#23423=CARTESIAN_POINT('Ctrl Pts',(-0.174735259276856,-1.,1.85948367089838));
#23424=CARTESIAN_POINT('Ctrl Pts',(-0.173946627589401,-1.,1.84898113200543));
#23425=CARTESIAN_POINT('Ctrl Pts',(-0.17288944289442,-1.,1.83658380530747));
#23426=CARTESIAN_POINT('Ctrl Pts',(-0.171554770207306,-1.,1.82215766815414));
#23427=CARTESIAN_POINT('Ctrl Pts',(-0.169936923908078,-1.,1.80561530633924));
#23428=CARTESIAN_POINT('Ctrl Pts',(-0.16803277280837,-1.,1.78690649988931));
#23429=CARTESIAN_POINT('Ctrl Pts',(-0.166279355148738,-1.,1.77018771687692));
#23430=CARTESIAN_POINT('Ctrl Pts',(-0.164834765708484,-1.,1.75666056640041));
#23431=CARTESIAN_POINT('Ctrl Pts',(-0.163814161002474,-1.,1.74720349503904));
#23432=CARTESIAN_POINT('Ctrl Pts',(-0.163289472382896,-1.,1.74236521665491));
#23433=CARTESIAN_POINT('',(-0.383122945602004,-1.,1.7075470150345));
#23434=CARTESIAN_POINT('Origin',(0.,-1.,0.));
#23435=CARTESIAN_POINT('',(-0.61342227326009,-1.,2.11275013067528));
#23436=CARTESIAN_POINT('Ctrl Pts',(-0.383122945602004,-1.,1.7075470150345));
#23437=CARTESIAN_POINT('Ctrl Pts',(-0.384119047314215,-1.,1.71231062891398));
#23438=CARTESIAN_POINT('Ctrl Pts',(-0.386070790323281,-1.,1.72162022244582));
#23439=CARTESIAN_POINT('Ctrl Pts',(-0.388877023502615,-1.,1.73493170972829));
#23440=CARTESIAN_POINT('Ctrl Pts',(-0.392375812285395,-1.,1.75137405310193));
#23441=CARTESIAN_POINT('Ctrl Pts',(-0.396346196110688,-1.,1.76975560043442));
#23442=CARTESIAN_POINT('Ctrl Pts',(-0.399919403774155,-1.,1.78598826343754));
#23443=CARTESIAN_POINT('Ctrl Pts',(-0.403107976163396,-1.,1.80012077173238));
#23444=CARTESIAN_POINT('Ctrl Pts',(-0.405933518407175,-1.,1.81223801812013));
#23445=CARTESIAN_POINT('Ctrl Pts',(-0.408428948106227,-1.,1.82247022677562));
#23446=CARTESIAN_POINT('Ctrl Pts',(-0.410641256301276,-1.,1.83100408895047));
#23447=CARTESIAN_POINT('Ctrl Pts',(-0.412633125322945,-1.,1.8380895347617));
#23448=CARTESIAN_POINT('Ctrl Pts',(-0.414487438255542,-1.,1.84405757074218));
#23449=CARTESIAN_POINT('Ctrl Pts',(-0.416300022039885,-1.,1.84929312930314));
#23450=CARTESIAN_POINT('Ctrl Pts',(-0.418164129144045,-1.,1.8541763285645));
#23451=CARTESIAN_POINT('Ctrl Pts',(-0.420157287975583,-1.,1.8590328109667));
#23452=CARTESIAN_POINT('Ctrl Pts',(-0.422327307417885,-1.,1.86408083333863));
#23453=CARTESIAN_POINT('Ctrl Pts',(-0.424678177290876,-1.,1.8693780394412));
#23454=CARTESIAN_POINT('Ctrl Pts',(-0.427183828518743,-1.,1.87486989291333));
#23455=CARTESIAN_POINT('Ctrl Pts',(-0.429803062482217,-1.,1.88044229001778));
#23456=CARTESIAN_POINT('Ctrl Pts',(-0.432493038548833,-1.,1.88596913666828));
#23457=CARTESIAN_POINT('Ctrl Pts',(-0.43522566096358,-1.,1.89136993975585));
#23458=CARTESIAN_POINT('Ctrl Pts',(-0.437995003948443,-1.,1.89663648956549));
#23459=CARTESIAN_POINT('Ctrl Pts',(-0.440807833704161,-1.,1.90180124389137));
#23460=CARTESIAN_POINT('Ctrl Pts',(-0.44367755684917,-1.,1.90691756144906));
#23461=CARTESIAN_POINT('Ctrl Pts',(-0.446617343485651,-1.,1.91203699981095));
#23462=CARTESIAN_POINT('Ctrl Pts',(-0.449632260106572,-1.,1.91718342555717));
#23463=CARTESIAN_POINT('Ctrl Pts',(-0.452719478359356,-1.,1.9223538064847));
#23464=CARTESIAN_POINT('Ctrl Pts',(-0.455872005174335,-1.,1.92753067150461));
#23465=CARTESIAN_POINT('Ctrl Pts',(-0.459081234547931,-1.,1.93269066517936));
#23466=CARTESIAN_POINT('Ctrl Pts',(-0.462340031009087,-1.,1.93781486640834));
#23467=CARTESIAN_POINT('Ctrl Pts',(-0.465645462026065,-1.,1.94289794196205));
#23468=CARTESIAN_POINT('Ctrl Pts',(-0.468997482913158,-1.,1.94794381136524));
#23469=CARTESIAN_POINT('Ctrl Pts',(-0.47239767226408,-1.,1.95296148278136));
#23470=CARTESIAN_POINT('Ctrl Pts',(-0.475848034683172,-1.,1.95796111148175));
#23471=CARTESIAN_POINT('Ctrl Pts',(-0.479349583074846,-1.,1.96294933055938));
#23472=CARTESIAN_POINT('Ctrl Pts',(-0.482901662120687,-1.,1.96792703422358));
#23473=CARTESIAN_POINT('Ctrl Pts',(-0.486502692907661,-1.,1.97289186263272));
#23474=CARTESIAN_POINT('Ctrl Pts',(-0.490150627860955,-1.,1.97783973019229));
#23475=CARTESIAN_POINT('Ctrl Pts',(-0.493843476541492,-1.,1.9827665876182));
#23476=CARTESIAN_POINT('Ctrl Pts',(-0.497579909545564,-1.,1.98767044752929));
#23477=CARTESIAN_POINT('Ctrl Pts',(-0.501359287727129,-1.,1.9925514912615));
#23478=CARTESIAN_POINT('Ctrl Pts',(-0.505181361323011,-1.,1.99741107463567));
#23479=CARTESIAN_POINT('Ctrl Pts',(-0.509046069886152,-1.,2.00225107134733));
#23480=CARTESIAN_POINT('Ctrl Pts',(-0.512953306961814,-1.,2.00707309946955));
#23481=CARTESIAN_POINT('Ctrl Pts',(-0.516902681728733,-1.,2.01187773939257));
#23482=CARTESIAN_POINT('Ctrl Pts',(-0.520893590399428,-1.,2.01666477917305));
#23483=CARTESIAN_POINT('Ctrl Pts',(-0.524925318333518,-1.,2.02143356304712));
#23484=CARTESIAN_POINT('Ctrl Pts',(-0.528997127241911,-1.,2.02618329083289));
#23485=CARTESIAN_POINT('Ctrl Pts',(-0.533108355132905,-1.,2.03091336214401));
#23486=CARTESIAN_POINT('Ctrl Pts',(-0.537258489833134,-1.,2.03562362953993));
#23487=CARTESIAN_POINT('Ctrl Pts',(-0.54144712061552,-1.,2.0403142269048));
#23488=CARTESIAN_POINT('Ctrl Pts',(-0.545673903817348,-1.,2.0449854471456));
#23489=CARTESIAN_POINT('Ctrl Pts',(-0.549938525150342,-1.,2.04963761077974));
#23490=CARTESIAN_POINT('Ctrl Pts',(-0.55424065746411,-1.,2.05427091604482));
#23491=CARTESIAN_POINT('Ctrl Pts',(-0.558579940185467,-1.,2.05888537756571));
#23492=CARTESIAN_POINT('Ctrl Pts',(-0.562955993082574,-1.,2.06348090160697));
#23493=CARTESIAN_POINT('Ctrl Pts',(-0.567368421181229,-1.,2.06805732997383));
#23494=CARTESIAN_POINT('Ctrl Pts',(-0.571816823242411,-1.,2.07261449292757));
#23495=CARTESIAN_POINT('Ctrl Pts',(-0.576300797416275,-1.,2.07715226767361));
#23496=CARTESIAN_POINT('Ctrl Pts',(-0.580819952107257,-1.,2.08167059018138));
#23497=CARTESIAN_POINT('Ctrl Pts',(-0.585373918990895,-1.,2.086169437277));
#23498=CARTESIAN_POINT('Ctrl Pts',(-0.589962365403189,-1.,2.09064881812053));
#23499=CARTESIAN_POINT('Ctrl Pts',(-0.594585006052824,-1.,2.09510876220501));
#23500=CARTESIAN_POINT('Ctrl Pts',(-0.599241616422144,-1.,2.09954930865331));
#23501=CARTESIAN_POINT('Ctrl Pts',(-0.603932030738212,-1.,2.10397049887709));
#23502=CARTESIAN_POINT('Ctrl Pts',(-0.607711315456826,-1.,2.10749199615859));
#23503=CARTESIAN_POINT('Ctrl Pts',(-0.610560911691113,-1.,2.11012443807661));
#23504=CARTESIAN_POINT('Ctrl Pts',(-0.61246736556225,-1.,2.11187554260142));
#23505=CARTESIAN_POINT('Ctrl Pts',(-0.61342227326009,-1.,2.11275013067528));
#23506=CARTESIAN_POINT('',(-0.745574324794401,-1.,2.0698113262342));
#23507=CARTESIAN_POINT('',(-0.61342227326009,-1.,2.11275013067528));
#23508=CARTESIAN_POINT('',(-0.693717979106306,-1.,1.60662857109684));
#23509=CARTESIAN_POINT('Ctrl Pts',(-0.745574324794401,-1.,2.0698113262342));
#23510=CARTESIAN_POINT('Ctrl Pts',(-0.74583279137781,-1.,2.06854248895575));
#23511=CARTESIAN_POINT('Ctrl Pts',(-0.746345871542696,-1.,2.06600523016401));
#23512=CARTESIAN_POINT('Ctrl Pts',(-0.747103932785504,-1.,2.06220058927162));
#23513=CARTESIAN_POINT('Ctrl Pts',(-0.748091554181101,-1.,2.05713023030263));
#23514=CARTESIAN_POINT('Ctrl Pts',(-0.749287468663053,-1.,2.05079645591606));
#23515=CARTESIAN_POINT('Ctrl Pts',(-0.750444657874758,-1.,2.04446689147754));
#23516=CARTESIAN_POINT('Ctrl Pts',(-0.751562963361384,-1.,2.03814160092173));
#23517=CARTESIAN_POINT('Ctrl Pts',(-0.752642180488104,-1.,2.03182068456467));
#23518=CARTESIAN_POINT('Ctrl Pts',(-0.753682061113766,-1.,2.02550428623587));
#23519=CARTESIAN_POINT('Ctrl Pts',(-0.75468233072352,-1.,2.01919259406003));
#23520=CARTESIAN_POINT('Ctrl Pts',(-0.7556427049581,-1.,2.01288584328149));
#23521=CARTESIAN_POINT('Ctrl Pts',(-0.756562904646496,-1.,2.00658431587682));
#23522=CARTESIAN_POINT('Ctrl Pts',(-0.757442676862341,-1.,2.00028834739072));
#23523=CARTESIAN_POINT('Ctrl Pts',(-0.758281796766377,-1.,1.9939983109871));
#23524=CARTESIAN_POINT('Ctrl Pts',(-0.759080037802243,-1.,1.98771456680806));
#23525=CARTESIAN_POINT('Ctrl Pts',(-0.759837147452135,-1.,1.98143741418156));
#23526=CARTESIAN_POINT('Ctrl Pts',(-0.760552825409855,-1.,1.97516705321521));
#23527=CARTESIAN_POINT('Ctrl Pts',(-0.761226690483986,-1.,1.96890351582545));
#23528=CARTESIAN_POINT('Ctrl Pts',(-0.761858300014575,-1.,1.96264672744229));
#23529=CARTESIAN_POINT('Ctrl Pts',(-0.762447203806263,-1.,1.95639665309893));
#23530=CARTESIAN_POINT('Ctrl Pts',(-0.762992990878774,-1.,1.95015342590025));
#23531=CARTESIAN_POINT('Ctrl Pts',(-0.76349533353858,-1.,1.94391746617626));
#23532=CARTESIAN_POINT('Ctrl Pts',(-0.763954049121393,-1.,1.93768964875867));
#23533=CARTESIAN_POINT('Ctrl Pts',(-0.764369010673889,-1.,1.93147105496367));
#23534=CARTESIAN_POINT('Ctrl Pts',(-0.764740025488189,-1.,1.92526263537041));
#23535=CARTESIAN_POINT('Ctrl Pts',(-0.765066729667095,-1.,1.91906491634197));
#23536=CARTESIAN_POINT('Ctrl Pts',(-0.765348465884739,-1.,1.91287765805174));
#23537=CARTESIAN_POINT('Ctrl Pts',(-0.765584196937936,-1.,1.90669961402362));
#23538=CARTESIAN_POINT('Ctrl Pts',(-0.765772772593395,-1.,1.90052930393599));
#23539=CARTESIAN_POINT('Ctrl Pts',(-0.765913193856979,-1.,1.89436577771389));
#23540=CARTESIAN_POINT('Ctrl Pts',(-0.76600483706209,-1.,1.88820926433409));
#23541=CARTESIAN_POINT('Ctrl Pts',(-0.766047794851869,-1.,1.88206215302561));
#23542=CARTESIAN_POINT('Ctrl Pts',(-0.766042837036759,-1.,1.87592888967886));
#23543=CARTESIAN_POINT('Ctrl Pts',(-0.765990708546111,-1.,1.86981398314345));
#23544=CARTESIAN_POINT('Ctrl Pts',(-0.765891519092557,-1.,1.86372027063314));
#23545=CARTESIAN_POINT('Ctrl Pts',(-0.765744212909305,-1.,1.85764741390391));
#23546=CARTESIAN_POINT('Ctrl Pts',(-0.765545710619023,-1.,1.85158945130054));
#23547=CARTESIAN_POINT('Ctrl Pts',(-0.765291664861971,-1.,1.8455369887591));
#23548=CARTESIAN_POINT('Ctrl Pts',(-0.764978057881687,-1.,1.83948181064823));
#23549=CARTESIAN_POINT('Ctrl Pts',(-0.764602549687845,-1.,1.8334207722714));
#23550=CARTESIAN_POINT('Ctrl Pts',(-0.764165902606055,-1.,1.8273599120008));
#23551=CARTESIAN_POINT('Ctrl Pts',(-0.763673465462854,-1.,1.82131873145297));
#23552=CARTESIAN_POINT('Ctrl Pts',(-0.763132003836783,-1.,1.81532118405566));
#23553=CARTESIAN_POINT('Ctrl Pts',(-0.762546129464036,-1.,1.80938551463989));
#23554=CARTESIAN_POINT('Ctrl Pts',(-0.761915336443516,-1.,1.80351583877334));
#23555=CARTESIAN_POINT('Ctrl Pts',(-0.761229695230359,-1.,1.79768986997735));
#23556=CARTESIAN_POINT('Ctrl Pts',(-0.760469555880425,-1.,1.79185815610802));
#23557=CARTESIAN_POINT('Ctrl Pts',(-0.759614401109868,-1.,1.78596964884526));
#23558=CARTESIAN_POINT('Ctrl Pts',(-0.75865062667738,-1.,1.77999411220912));
#23559=CARTESIAN_POINT('Ctrl Pts',(-0.757578264077238,-1.,1.77394167108342));
#23560=CARTESIAN_POINT('Ctrl Pts',(-0.756421896028403,-1.,1.76789396003141));
#23561=CARTESIAN_POINT('Ctrl Pts',(-0.755220979975262,-1.,1.7619781724032));
#23562=CARTESIAN_POINT('Ctrl Pts',(-0.75400925402848,-1.,1.75631083600175));
#23563=CARTESIAN_POINT('Ctrl Pts',(-0.752797683531377,-1.,1.75095139468809));
#23564=CARTESIAN_POINT('Ctrl Pts',(-0.751555614163629,-1.,1.74585086852298));
#23565=CARTESIAN_POINT('Ctrl Pts',(-0.75019343597954,-1.,1.74080458266705));
#23566=CARTESIAN_POINT('Ctrl Pts',(-0.748582462954855,-1.,1.73550351679848));
#23567=CARTESIAN_POINT('Ctrl Pts',(-0.746574710096436,-1.,1.72958533647399));
#23568=CARTESIAN_POINT('Ctrl Pts',(-0.744021445433764,-1.,1.7226822991693));
#23569=CARTESIAN_POINT('Ctrl Pts',(-0.740795162032088,-1.,1.71447789751927));
#23570=CARTESIAN_POINT('Ctrl Pts',(-0.736799665724771,-1.,1.70473309006121));
#23571=CARTESIAN_POINT('Ctrl Pts',(-0.731963238697195,-1.,1.69326921975743));
#23572=CARTESIAN_POINT('Ctrl Pts',(-0.726235967997433,-1.,1.67996158455503));
#23573=CARTESIAN_POINT('Ctrl Pts',(-0.719585433804282,-1.,1.6647288055568));
#23574=CARTESIAN_POINT('Ctrl Pts',(-0.711993139355394,-1.,1.64752408832016));
#23575=CARTESIAN_POINT('Ctrl Pts',(-0.705159151988319,-1.,1.63216541664676));
#23576=CARTESIAN_POINT('Ctrl Pts',(-0.699605146405088,-1.,1.61974673472612));
#23577=CARTESIAN_POINT('Ctrl Pts',(-0.695712097881194,-1.,1.61106790958151));
#23578=CARTESIAN_POINT('Ctrl Pts',(-0.693717979106306,-1.,1.60662857109684));
#23579=CARTESIAN_POINT('',(-0.892032620296855,-1.,1.5055822144029));
#23580=CARTESIAN_POINT('Origin',(0.,-1.,0.));
#23581=CARTESIAN_POINT('',(-1.23627494547115,-1.,1.81978687191668));
#23582=CARTESIAN_POINT('Ctrl Pts',(-0.892032620296855,-1.,1.5055822144029));
#23583=CARTESIAN_POINT('Ctrl Pts',(-0.894452006964543,-1.,1.50980486806688));
#23584=CARTESIAN_POINT('Ctrl Pts',(-0.899185047483511,-1.,1.51805569590094));
#23585=CARTESIAN_POINT('Ctrl Pts',(-0.905967409625651,-1.,1.52984849887993));
#23586=CARTESIAN_POINT('Ctrl Pts',(-0.914375919026456,-1.,1.54440491149498));
#23587=CARTESIAN_POINT('Ctrl Pts',(-0.923832188944341,-1.,1.56065988578893));
#23588=CARTESIAN_POINT('Ctrl Pts',(-0.932246680108685,-1.,1.57499388382243));
#23589=CARTESIAN_POINT('Ctrl Pts',(-0.939646377893399,-1.,1.58744937487176));
#23590=CARTESIAN_POINT('Ctrl Pts',(-0.946078063315257,-1.,1.59810042043673));
#23591=CARTESIAN_POINT('Ctrl Pts',(-0.951613284356035,-1.,1.60706069896936));
#23592=CARTESIAN_POINT('Ctrl Pts',(-0.956354422920671,-1.,1.61449324337085));
#23593=CARTESIAN_POINT('Ctrl Pts',(-0.960438326101729,-1.,1.62061638140221));
#23594=CARTESIAN_POINT('Ctrl Pts',(-0.964046107040536,-1.,1.62571930670187));
#23595=CARTESIAN_POINT('Ctrl Pts',(-0.967387853230345,-1.,1.63013849959461));
#23596=CARTESIAN_POINT('Ctrl Pts',(-0.970669715997509,-1.,1.63420665729798));
#23597=CARTESIAN_POINT('Ctrl Pts',(-0.974066058287418,-1.,1.63820952658144));
#23598=CARTESIAN_POINT('Ctrl Pts',(-0.977689794119416,-1.,1.64233990826687));
#23599=CARTESIAN_POINT('Ctrl Pts',(-0.981562530939489,-1.,1.64665139190656));
#23600=CARTESIAN_POINT('Ctrl Pts',(-0.985642622920821,-1.,1.65110016612638));
#23601=CARTESIAN_POINT('Ctrl Pts',(-0.989855627854165,-1.,1.65559044289699));
#23602=CARTESIAN_POINT('Ctrl Pts',(-0.994121836661306,-1.,1.66001553809947));
#23603=CARTESIAN_POINT('Ctrl Pts',(-0.998389654952758,-1.,1.66430758030376));
#23604=CARTESIAN_POINT('Ctrl Pts',(-1.00265091003727,-1.,1.66846059277303));
#23605=CARTESIAN_POINT('Ctrl Pts',(-1.00692206696414,-1.,1.67250335383293));
#23606=CARTESIAN_POINT('Ctrl Pts',(-1.01123236493511,-1.,1.67648246776464));
#23607=CARTESIAN_POINT('Ctrl Pts',(-1.01561026162773,-1.,1.68044289894798));
#23608=CARTESIAN_POINT('Ctrl Pts',(-1.02006795074201,-1.,1.68440578021706));
#23609=CARTESIAN_POINT('Ctrl Pts',(-1.02460180535255,-1.,1.68836910178447));
#23610=CARTESIAN_POINT('Ctrl Pts',(-1.02919977579147,-1.,1.69231840863458));
#23611=CARTESIAN_POINT('Ctrl Pts',(-1.03384646003588,-1.,1.69623414782771));
#23612=CARTESIAN_POINT('Ctrl Pts',(-1.03852922490789,-1.,1.70010052930962));
#23613=CARTESIAN_POINT('Ctrl Pts',(-1.04324363334554,-1.,1.70391338707982));
#23614=CARTESIAN_POINT('Ctrl Pts',(-1.04799085404995,-1.,1.70767646263649));
#23615=CARTESIAN_POINT('Ctrl Pts',(-1.05277517202855,-1.,1.71139783543989));
#23616=CARTESIAN_POINT('Ctrl Pts',(-1.05760163192479,-1.,1.7150865442702));
#23617=CARTESIAN_POINT('Ctrl Pts',(-1.06247324680647,-1.,1.71874858456904));
#23618=CARTESIAN_POINT('Ctrl Pts',(-1.06738966975462,-1.,1.72238500928453));
#23619=CARTESIAN_POINT('Ctrl Pts',(-1.07234866990252,-1.,1.72599406198488));
#23620=CARTESIAN_POINT('Ctrl Pts',(-1.0773470373727,-1.,1.72957248977424));
#23621=CARTESIAN_POINT('Ctrl Pts',(-1.08238162784749,-1.,1.73311705663407));
#23622=CARTESIAN_POINT('Ctrl Pts',(-1.08745056285427,-1.,1.73662628326091));
#23623=CARTESIAN_POINT('Ctrl Pts',(-1.09255329056493,-1.,1.74010053962247));
#23624=CARTESIAN_POINT('Ctrl Pts',(-1.09768999241225,-1.,1.74354119236208));
#23625=CARTESIAN_POINT('Ctrl Pts',(-1.10286118991143,-1.,1.74695004214923));
#23626=CARTESIAN_POINT('Ctrl Pts',(-1.10806728183007,-1.,1.7503286607592));
#23627=CARTESIAN_POINT('Ctrl Pts',(-1.11330807582551,-1.,1.7536777209463));
#23628=CARTESIAN_POINT('Ctrl Pts',(-1.11858293216763,-1.,1.75699720772105));
#23629=CARTESIAN_POINT('Ctrl Pts',(-1.12389096855086,-1.,1.76028671825096));
#23630=CARTESIAN_POINT('Ctrl Pts',(-1.12923123555075,-1.,1.7635457196617));
#23631=CARTESIAN_POINT('Ctrl Pts',(-1.1346029180462,-1.,1.76677384551862));
#23632=CARTESIAN_POINT('Ctrl Pts',(-1.14000548336975,-1.,1.76997111386769));
#23633=CARTESIAN_POINT('Ctrl Pts',(-1.1454385822692,-1.,1.77313777896194));
#23634=CARTESIAN_POINT('Ctrl Pts',(-1.15090197841515,-1.,1.7762742255701));
#23635=CARTESIAN_POINT('Ctrl Pts',(-1.15639547194698,-1.,1.77938085564275));
#23636=CARTESIAN_POINT('Ctrl Pts',(-1.16191881298499,-1.,1.78245795881009));
#23637=CARTESIAN_POINT('Ctrl Pts',(-1.16747166312303,-1.,1.78550566040443));
#23638=CARTESIAN_POINT('Ctrl Pts',(-1.17305363177328,-1.,1.78852398877616));
#23639=CARTESIAN_POINT('Ctrl Pts',(-1.17866429440809,-1.,1.79151291552689));
#23640=CARTESIAN_POINT('Ctrl Pts',(-1.18430321697432,-1.,1.79447240321515));
#23641=CARTESIAN_POINT('Ctrl Pts',(-1.18996997934445,-1.,1.79740245923478));
#23642=CARTESIAN_POINT('Ctrl Pts',(-1.19566418930242,-1.,1.80030314369879));
#23643=CARTESIAN_POINT('Ctrl Pts',(-1.20138548938974,-1.,1.80317454838603));
#23644=CARTESIAN_POINT('Ctrl Pts',(-1.20713356605475,-1.,1.80601678480707));
#23645=CARTESIAN_POINT('Ctrl Pts',(-1.21290815708314,-1.,1.80882996917129));
#23646=CARTESIAN_POINT('Ctrl Pts',(-1.21870906103557,-1.,1.81161420806656));
#23647=CARTESIAN_POINT('Ctrl Pts',(-1.2245361330495,-1.,1.81436959210434));
#23648=CARTESIAN_POINT('Ctrl Pts',(-1.2292186489137,-1.,1.8165508718364));
#23649=CARTESIAN_POINT('Ctrl Pts',(-1.2327422452705,-1.,1.81817389921279));
#23650=CARTESIAN_POINT('Ctrl Pts',(-1.23509651170476,-1.,1.81925017193666));
#23651=CARTESIAN_POINT('Ctrl Pts',(-1.23627494547115,-1.,1.81978687191668));
#23652=CARTESIAN_POINT('',(-1.34869019493419,-1.,1.73811241238545));
#23653=CARTESIAN_POINT('',(-1.23627494547115,-1.,1.81978687191668));
#23654=CARTESIAN_POINT('',(-1.15624053661742,-1.,1.31362392696032));
#23655=CARTESIAN_POINT('Ctrl Pts',(-1.34869019493419,-1.,1.73811241238545));
#23656=CARTESIAN_POINT('Ctrl Pts',(-1.34854391898045,-1.,1.73682580585691));
#23657=CARTESIAN_POINT('Ctrl Pts',(-1.34824783112887,-1.,1.73425417885907));
#23658=CARTESIAN_POINT('Ctrl Pts',(-1.34779309152035,-1.,1.7304014965394));
#23659=CARTESIAN_POINT('Ctrl Pts',(-1.34716554819527,-1.,1.72527410680674));
#23660=CARTESIAN_POINT('Ctrl Pts',(-1.34634568653227,-1.,1.7188807715049));
#23661=CARTESIAN_POINT('Ctrl Pts',(-1.34549029589416,-1.,1.71250340686822));
#23662=CARTESIAN_POINT('Ctrl Pts',(-1.34459924533831,-1.,1.70614212266738));
#23663=CARTESIAN_POINT('Ctrl Pts',(-1.34367237124483,-1.,1.69979707754427));
#23664=CARTESIAN_POINT('Ctrl Pts',(-1.34270948206319,-1.,1.6934684849687));
#23665=CARTESIAN_POINT('Ctrl Pts',(-1.341710374848,-1.,1.68715660868764));
#23666=CARTESIAN_POINT('Ctrl Pts',(-1.34067485185203,-1.,1.68086176030362));
#23667=CARTESIAN_POINT('Ctrl Pts',(-1.3396027347034,-1.,1.67458429426086));
#23668=CARTESIAN_POINT('Ctrl Pts',(-1.33849388654388,-1.,1.66832460783989));
#23669=CARTESIAN_POINT('Ctrl Pts',(-1.33734820885262,-1.,1.66208312541983));
#23670=CARTESIAN_POINT('Ctrl Pts',(-1.33616559745172,-1.,1.65586025952593));
#23671=CARTESIAN_POINT('Ctrl Pts',(-1.33494590467993,-1.,1.6496563728683));
#23672=CARTESIAN_POINT('Ctrl Pts',(-1.33368890676572,-1.,1.6434717485603));
#23673=CARTESIAN_POINT('Ctrl Pts',(-1.33239425103724,-1.,1.63730653475089));
#23674=CARTESIAN_POINT('Ctrl Pts',(-1.33106149345645,-1.,1.63116079730923));
#23675=CARTESIAN_POINT('Ctrl Pts',(-1.3296901950568,-1.,1.62503464209797));
#23676=CARTESIAN_POINT('Ctrl Pts',(-1.32828000610449,-1.,1.61892832270724));
#23677=CARTESIAN_POINT('Ctrl Pts',(-1.32683074483356,-1.,1.6128423401575));
#23678=CARTESIAN_POINT('Ctrl Pts',(-1.32534250785782,-1.,1.60677758290954));
#23679=CARTESIAN_POINT('Ctrl Pts',(-1.32381550858256,-1.,1.60073511858687));
#23680=CARTESIAN_POINT('Ctrl Pts',(-1.32224985747682,-1.,1.59471591079403));
#23681=CARTESIAN_POINT('Ctrl Pts',(-1.32064537110892,-1.,1.58872057258245));
#23682=CARTESIAN_POINT('Ctrl Pts',(-1.31900135021432,-1.,1.58274907898834));
#23683=CARTESIAN_POINT('Ctrl Pts',(-1.31731642317187,-1.,1.5768005650559));
#23684=CARTESIAN_POINT('Ctrl Pts',(-1.31558903860016,-1.,1.57087397835723));
#23685=CARTESIAN_POINT('Ctrl Pts',(-1.31381795281002,-1.,1.56496872402353));
#23686=CARTESIAN_POINT('Ctrl Pts',(-1.31200264341696,-1.,1.55908521254821));
#23687=CARTESIAN_POINT('Ctrl Pts',(-1.31014393684222,-1.,1.55322568759481));
#23688=CARTESIAN_POINT('Ctrl Pts',(-1.30824393907473,-1.,1.54739413957185));
#23689=CARTESIAN_POINT('Ctrl Pts',(-1.30630475189556,-1.,1.54159462645432));
#23690=CARTESIAN_POINT('Ctrl Pts',(-1.30432735639489,-1.,1.53582981268977));
#23691=CARTESIAN_POINT('Ctrl Pts',(-1.30231064395568,-1.,1.53009970283891));
#23692=CARTESIAN_POINT('Ctrl Pts',(-1.30024984366328,-1.,1.52439957861062));
#23693=CARTESIAN_POINT('Ctrl Pts',(-1.29813791800747,-1.,1.51872184912724));
#23694=CARTESIAN_POINT('Ctrl Pts',(-1.29596850710509,-1.,1.51305994241402));
#23695=CARTESIAN_POINT('Ctrl Pts',(-1.29373841372842,-1.,1.50741159078365));
#23696=CARTESIAN_POINT('Ctrl Pts',(-1.29145022885181,-1.,1.50178230149776));
#23697=CARTESIAN_POINT('Ctrl Pts',(-1.28911506584254,-1.,1.49618896881754));
#23698=CARTESIAN_POINT('Ctrl Pts',(-1.2867467611644,-1.,1.4906522831278));
#23699=CARTESIAN_POINT('Ctrl Pts',(-1.28435533880201,-1.,1.4851881711891));
#23700=CARTESIAN_POINT('Ctrl Pts',(-1.28194158939517,-1.,1.47980070347095));
#23701=CARTESIAN_POINT('Ctrl Pts',(-1.2794891824849,-1.,1.4744717526707));
#23702=CARTESIAN_POINT('Ctrl Pts',(-1.27696414831089,-1.,1.46916035917133));
#23703=CARTESIAN_POINT('Ctrl Pts',(-1.27433119897822,-1.,1.46382431332476));
#23704=CARTESIAN_POINT('Ctrl Pts',(-1.27156805265289,-1.,1.45843906294697));
#23705=CARTESIAN_POINT('Ctrl Pts',(-1.2686778680489,-1.,1.45301422764247));
#23706=CARTESIAN_POINT('Ctrl Pts',(-1.26570925118868,-1.,1.44761985001662));
#23707=CARTESIAN_POINT('Ctrl Pts',(-1.26273903323859,-1.,1.44236470511303));
#23708=CARTESIAN_POINT('Ctrl Pts',(-1.25983531012005,-1.,1.43734919180848));
#23709=CARTESIAN_POINT('Ctrl Pts',(-1.25702687965755,-1.,1.43262645609691));
#23710=CARTESIAN_POINT('Ctrl Pts',(-1.25426945222639,-1.,1.42815938799387));
#23711=CARTESIAN_POINT('Ctrl Pts',(-1.2514145557001,-1.,1.42378102115575));
#23712=CARTESIAN_POINT('Ctrl Pts',(-1.24824430986571,-1.,1.41923722596025));
#23713=CARTESIAN_POINT('Ctrl Pts',(-1.24450600513056,-1.,1.41422913175179));
#23714=CARTESIAN_POINT('Ctrl Pts',(-1.23994455029534,-1.,1.40845295531283));
#23715=CARTESIAN_POINT('Ctrl Pts',(-1.23434087290423,-1.,1.40164708206106));
#23716=CARTESIAN_POINT('Ctrl Pts',(-1.22752961899387,-1.,1.39361389568796));
#23717=CARTESIAN_POINT('Ctrl Pts',(-1.21938737280852,-1.,1.38420564527715));
#23718=CARTESIAN_POINT('Ctrl Pts',(-1.20982812925645,-1.,1.37331915607905));
#23719=CARTESIAN_POINT('Ctrl Pts',(-1.1987959077932,-1.,1.36088705043885));
#23720=CARTESIAN_POINT('Ctrl Pts',(-1.18625865667441,-1.,1.34687054001093));
#23721=CARTESIAN_POINT('Ctrl Pts',(-1.17501305789857,-1.,1.33437539347008));
#23722=CARTESIAN_POINT('Ctrl Pts',(-1.16589330093588,-1.,1.32428080721772));
#23723=CARTESIAN_POINT('Ctrl Pts',(-1.15950888730809,-1.,1.31722977216397));
#23724=CARTESIAN_POINT('Ctrl Pts',(-1.15624053661742,-1.,1.31362392696032));
#23725=CARTESIAN_POINT('',(-1.31362392696033,-1.,1.15624053661742));
#23726=CARTESIAN_POINT('Origin',(0.,-1.,0.));
#23727=CARTESIAN_POINT('',(-1.73811241238545,-1.,1.34869019493419));
#23728=CARTESIAN_POINT('Ctrl Pts',(-1.31362392696033,-1.,1.15624053661742));
#23729=CARTESIAN_POINT('Ctrl Pts',(-1.3172297721596,-1.,1.15950888730433));
#23730=CARTESIAN_POINT('Ctrl Pts',(-1.32428080720544,-1.,1.16589330092532));
#23731=CARTESIAN_POINT('Ctrl Pts',(-1.33437539344842,-1.,1.17501305787994));
#23732=CARTESIAN_POINT('Ctrl Pts',(-1.34687053998157,-1.,1.18625865664915));
#23733=CARTESIAN_POINT('Ctrl Pts',(-1.36088705040677,-1.,1.1987959077656));
#23734=CARTESIAN_POINT('Ctrl Pts',(-1.37331915604962,-1.,1.20982812923113));
#23735=CARTESIAN_POINT('Ctrl Pts',(-1.38420564525391,-1.,1.21938737278853));
#23736=CARTESIAN_POINT('Ctrl Pts',(-1.39361389567257,-1.,1.22752961898063));
#23737=CARTESIAN_POINT('Ctrl Pts',(-1.40164708205345,-1.,1.23434087289768));
#23738=CARTESIAN_POINT('Ctrl Pts',(-1.40845295531151,-1.,1.23994455029421));
#23739=CARTESIAN_POINT('Ctrl Pts',(-1.41422913175437,-1.,1.24450600513278));
#23740=CARTESIAN_POINT('Ctrl Pts',(-1.41923722596421,-1.,1.24824430986911));
#23741=CARTESIAN_POINT('Ctrl Pts',(-1.42378102115911,-1.,1.25141455570299));
#23742=CARTESIAN_POINT('Ctrl Pts',(-1.42815938799555,-1.,1.25426945222783));
#23743=CARTESIAN_POINT('Ctrl Pts',(-1.43262645609679,-1.,1.25702687965744));
#23744=CARTESIAN_POINT('Ctrl Pts',(-1.43734919180719,-1.,1.25983531011894));
#23745=CARTESIAN_POINT('Ctrl Pts',(-1.44236470511145,-1.,1.26273903323723));
#23746=CARTESIAN_POINT('Ctrl Pts',(-1.44761985001544,-1.,1.26570925118767));
#23747=CARTESIAN_POINT('Ctrl Pts',(-1.45301422764205,-1.,1.26867786804854));
#23748=CARTESIAN_POINT('Ctrl Pts',(-1.45843906294725,-1.,1.27156805265312));
#23749=CARTESIAN_POINT('Ctrl Pts',(-1.4638243133254,-1.,1.27433119897877));
#23750=CARTESIAN_POINT('Ctrl Pts',(-1.46916035917197,-1.,1.27696414831144));
#23751=CARTESIAN_POINT('Ctrl Pts',(-1.4744717526711,-1.,1.27948918248524));
#23752=CARTESIAN_POINT('Ctrl Pts',(-1.47980070347102,-1.,1.28194158939522));
#23753=CARTESIAN_POINT('Ctrl Pts',(-1.48518817118891,-1.,1.28435533880184));
#23754=CARTESIAN_POINT('Ctrl Pts',(-1.4906522831275,-1.,1.28674676116415));
#23755=CARTESIAN_POINT('Ctrl Pts',(-1.49618896881729,-1.,1.28911506584232));
#23756=CARTESIAN_POINT('Ctrl Pts',(-1.50178230149764,-1.,1.29145022885171));
#23757=CARTESIAN_POINT('Ctrl Pts',(-1.50741159078367,-1.,1.29373841372843));
#23758=CARTESIAN_POINT('Ctrl Pts',(-1.51305994241412,-1.,1.29596850710518));
#23759=CARTESIAN_POINT('Ctrl Pts',(-1.51872184912735,-1.,1.29813791800757));
#23760=CARTESIAN_POINT('Ctrl Pts',(-1.5243995786107,-1.,1.30024984366334));
#23761=CARTESIAN_POINT('Ctrl Pts',(-1.53009970283893,-1.,1.3023106439557));
#23762=CARTESIAN_POINT('Ctrl Pts',(-1.53582981268976,-1.,1.30432735639487));
#23763=CARTESIAN_POINT('Ctrl Pts',(-1.54159462645428,-1.,1.30630475189553));
#23764=CARTESIAN_POINT('Ctrl Pts',(-1.54739413957183,-1.,1.30824393907471));
#23765=CARTESIAN_POINT('Ctrl Pts',(-1.55322568759481,-1.,1.31014393684221));
#23766=CARTESIAN_POINT('Ctrl Pts',(-1.55908521254822,-1.,1.31200264341696));
#23767=CARTESIAN_POINT('Ctrl Pts',(-1.56496872402352,-1.,1.31381795281002));
#23768=CARTESIAN_POINT('Ctrl Pts',(-1.57087397835721,-1.,1.31558903860015));
#23769=CARTESIAN_POINT('Ctrl Pts',(-1.57680056505585,-1.,1.31731642317183));
#23770=CARTESIAN_POINT('Ctrl Pts',(-1.58274907898829,-1.,1.31900135021428));
#23771=CARTESIAN_POINT('Ctrl Pts',(-1.58872057258244,-1.,1.32064537110891));
#23772=CARTESIAN_POINT('Ctrl Pts',(-1.59471591079408,-1.,1.32224985747686));
#23773=CARTESIAN_POINT('Ctrl Pts',(-1.600735118587,-1.,1.32381550858266));
#23774=CARTESIAN_POINT('Ctrl Pts',(-1.6067775829097,-1.,1.32534250785794));
#23775=CARTESIAN_POINT('Ctrl Pts',(-1.61284234015762,-1.,1.32683074483365));
#23776=CARTESIAN_POINT('Ctrl Pts',(-1.61892832270723,-1.,1.32828000610448));
#23777=CARTESIAN_POINT('Ctrl Pts',(-1.62503464209777,-1.,1.32969019505665));
#23778=CARTESIAN_POINT('Ctrl Pts',(-1.63116079730887,-1.,1.33106149345618));
#23779=CARTESIAN_POINT('Ctrl Pts',(-1.6373065347505,-1.,1.33239425103694));
#23780=CARTESIAN_POINT('Ctrl Pts',(-1.64347174856007,-1.,1.33368890676554));
#23781=CARTESIAN_POINT('Ctrl Pts',(-1.64965637286843,-1.,1.33494590468003));
#23782=CARTESIAN_POINT('Ctrl Pts',(-1.65586025952651,-1.,1.33616559745217));
#23783=CARTESIAN_POINT('Ctrl Pts',(-1.66208312542073,-1.,1.33734820885331));
#23784=CARTESIAN_POINT('Ctrl Pts',(-1.66832460784078,-1.,1.33849388654458));
#23785=CARTESIAN_POINT('Ctrl Pts',(-1.67458429426126,-1.,1.33960273470372));
#23786=CARTESIAN_POINT('Ctrl Pts',(-1.68086176030308,-1.,1.3406748518516));
#23787=CARTESIAN_POINT('Ctrl Pts',(-1.68715660868602,-1.,1.34171037484673));
#23788=CARTESIAN_POINT('Ctrl Pts',(-1.6934684849664,-1.,1.34270948206139));
#23789=CARTESIAN_POINT('Ctrl Pts',(-1.69979707754221,-1.,1.34367237124322));
#23790=CARTESIAN_POINT('Ctrl Pts',(-1.70614212266676,-1.,1.34459924533783));
#23791=CARTESIAN_POINT('Ctrl Pts',(-1.71250340687011,-1.,1.34549029589563));
#23792=CARTESIAN_POINT('Ctrl Pts',(-1.7188807715095,-1.,1.34634568653586));
#23793=CARTESIAN_POINT('Ctrl Pts',(-1.72527410681298,-1.,1.34716554820013));
#23794=CARTESIAN_POINT('Ctrl Pts',(-1.73040149654497,-1.,1.3477930915247));
#23795=CARTESIAN_POINT('Ctrl Pts',(-1.73425417886255,-1.,1.34824783113158));
#23796=CARTESIAN_POINT('Ctrl Pts',(-1.73682580585819,-1.,1.34854391898145));
#23797=CARTESIAN_POINT('Ctrl Pts',(-1.73811241238545,-1.,1.34869019493419));
#23798=CARTESIAN_POINT('',(-1.81978687191668,-1.,1.23627494547115));
#23799=CARTESIAN_POINT('',(-1.73811241238545,-1.,1.34869019493419));
#23800=CARTESIAN_POINT('',(-1.5055822144029,-1.,0.892032620296855));
#23801=CARTESIAN_POINT('Ctrl Pts',(-1.81978687191668,-1.,1.23627494547115));
#23802=CARTESIAN_POINT('Ctrl Pts',(-1.81925017193531,-1.,1.23509651170384));
#23803=CARTESIAN_POINT('Ctrl Pts',(-1.81817389920914,-1.,1.23274224526804));
#23804=CARTESIAN_POINT('Ctrl Pts',(-1.81655087183054,-1.,1.22921864890975));
#23805=CARTESIAN_POINT('Ctrl Pts',(-1.81436959209778,-1.,1.22453613304507));
#23806=CARTESIAN_POINT('Ctrl Pts',(-1.81161420806172,-1.,1.2187090610323));
#23807=CARTESIAN_POINT('Ctrl Pts',(-1.80882996916931,-1.,1.2129081570818));
#23808=CARTESIAN_POINT('Ctrl Pts',(-1.80601678480772,-1.,1.20713356605519));
#23809=CARTESIAN_POINT('Ctrl Pts',(-1.8031745483882,-1.,1.2013854893912));
#23810=CARTESIAN_POINT('Ctrl Pts',(-1.80030314370121,-1.,1.19566418930405));
#23811=CARTESIAN_POINT('Ctrl Pts',(-1.79740245923649,-1.,1.1899699793456));
#23812=CARTESIAN_POINT('Ctrl Pts',(-1.79447240321572,-1.,1.18430321697471));
#23813=CARTESIAN_POINT('Ctrl Pts',(-1.79151291552646,-1.,1.17866429440781));
#23814=CARTESIAN_POINT('Ctrl Pts',(-1.78852398877523,-1.,1.17305363177265));
#23815=CARTESIAN_POINT('Ctrl Pts',(-1.78550566040349,-1.,1.16747166312239));
#23816=CARTESIAN_POINT('Ctrl Pts',(-1.78245795880949,-1.,1.16191881298458));
#23817=CARTESIAN_POINT('Ctrl Pts',(-1.77938085564261,-1.,1.15639547194689));
#23818=CARTESIAN_POINT('Ctrl Pts',(-1.77627422557034,-1.,1.15090197841531));
#23819=CARTESIAN_POINT('Ctrl Pts',(-1.77313777896234,-1.,1.14543858226948));
#23820=CARTESIAN_POINT('Ctrl Pts',(-1.76997111386806,-1.,1.14000548337));
#23821=CARTESIAN_POINT('Ctrl Pts',(-1.76677384551883,-1.,1.13460291804635));
#23822=CARTESIAN_POINT('Ctrl Pts',(-1.76354571966171,-1.,1.12923123555076));
#23823=CARTESIAN_POINT('Ctrl Pts',(-1.76028671825084,-1.,1.12389096855078));
#23824=CARTESIAN_POINT('Ctrl Pts',(-1.75699720772089,-1.,1.11858293216752));
#23825=CARTESIAN_POINT('Ctrl Pts',(-1.75367772094617,-1.,1.11330807582542));
#23826=CARTESIAN_POINT('Ctrl Pts',(-1.75032866075914,-1.,1.10806728183003));
#23827=CARTESIAN_POINT('Ctrl Pts',(-1.74695004214924,-1.,1.10286118991144));
#23828=CARTESIAN_POINT('Ctrl Pts',(-1.74354119236212,-1.,1.09768999241229));
#23829=CARTESIAN_POINT('Ctrl Pts',(-1.74010053962252,-1.,1.09255329056496));
#23830=CARTESIAN_POINT('Ctrl Pts',(-1.73662628326093,-1.,1.08745056285429));
#23831=CARTESIAN_POINT('Ctrl Pts',(-1.73311705663407,-1.,1.08238162784749));
#23832=CARTESIAN_POINT('Ctrl Pts',(-1.72957248977424,-1.,1.0773470373727));
#23833=CARTESIAN_POINT('Ctrl Pts',(-1.72599406198489,-1.,1.07234866990252));
#23834=CARTESIAN_POINT('Ctrl Pts',(-1.72238500928456,-1.,1.06738966975463));
#23835=CARTESIAN_POINT('Ctrl Pts',(-1.71874858456908,-1.,1.0624732468065));
#23836=CARTESIAN_POINT('Ctrl Pts',(-1.71508654427022,-1.,1.05760163192481));
#23837=CARTESIAN_POINT('Ctrl Pts',(-1.71139783543986,-1.,1.05277517202854));
#23838=CARTESIAN_POINT('Ctrl Pts',(-1.70767646263641,-1.,1.0479908540499));
#23839=CARTESIAN_POINT('Ctrl Pts',(-1.70391338707969,-1.,1.04324363334546));
#23840=CARTESIAN_POINT('Ctrl Pts',(-1.70010052930951,-1.,1.03852922490782));
#23841=CARTESIAN_POINT('Ctrl Pts',(-1.69623414782769,-1.,1.03384646003587));
#23842=CARTESIAN_POINT('Ctrl Pts',(-1.69231840863471,-1.,1.02919977579155));
#23843=CARTESIAN_POINT('Ctrl Pts',(-1.68836910178475,-1.,1.02460180535272));
#23844=CARTESIAN_POINT('Ctrl Pts',(-1.68440578021739,-1.,1.02006795074222));
#23845=CARTESIAN_POINT('Ctrl Pts',(-1.6804428989482,-1.,1.01561026162787));
#23846=CARTESIAN_POINT('Ctrl Pts',(-1.67648246776457,-1.,1.01123236493507));
#23847=CARTESIAN_POINT('Ctrl Pts',(-1.67250335383248,-1.,1.00692206696387));
#23848=CARTESIAN_POINT('Ctrl Pts',(-1.66846059277231,-1.,1.00265091003682));
#23849=CARTESIAN_POINT('Ctrl Pts',(-1.66430758030304,-1.,0.998389654952317));
#23850=CARTESIAN_POINT('Ctrl Pts',(-1.66001553809916,-1.,0.994121836661116));
#23851=CARTESIAN_POINT('Ctrl Pts',(-1.65559044289746,-1.,0.98985562785445));
#23852=CARTESIAN_POINT('Ctrl Pts',(-1.6511001661277,-1.,0.985642622921626));
#23853=CARTESIAN_POINT('Ctrl Pts',(-1.64665139190834,-1.,0.981562530940574));
#23854=CARTESIAN_POINT('Ctrl Pts',(-1.64233990826831,-1.,0.977689794120297));
#23855=CARTESIAN_POINT('Ctrl Pts',(-1.63820952658157,-1.,0.974066058287501));
#23856=CARTESIAN_POINT('Ctrl Pts',(-1.63420665729609,-1.,0.970669715996356));
#23857=CARTESIAN_POINT('Ctrl Pts',(-1.63013849959083,-1.,0.967387853228041));
#23858=CARTESIAN_POINT('Ctrl Pts',(-1.6257193066974,-1.,0.964046107037821));
#23859=CARTESIAN_POINT('Ctrl Pts',(-1.62061638139929,-1.,0.960438326099958));
#23860=CARTESIAN_POINT('Ctrl Pts',(-1.61449324337233,-1.,0.956354422921573));
#23861=CARTESIAN_POINT('Ctrl Pts',(-1.60706069897794,-1.,0.951613284361248));
#23862=CARTESIAN_POINT('Ctrl Pts',(-1.59810042045408,-1.,0.946078063325796));
#23863=CARTESIAN_POINT('Ctrl Pts',(-1.58744937489796,-1.,0.939646377909319));
#23864=CARTESIAN_POINT('Ctrl Pts',(-1.57499388385561,-1.,0.932246680128849));
#23865=CARTESIAN_POINT('Ctrl Pts',(-1.56065988582509,-1.,0.923832188966322));
#23866=CARTESIAN_POINT('Ctrl Pts',(-1.54440491152808,-1.,0.91437591904658));
#23867=CARTESIAN_POINT('Ctrl Pts',(-1.52984849890434,-1.,0.905967409640499));
#23868=CARTESIAN_POINT('Ctrl Pts',(-1.51805569591479,-1.,0.89918504749193));
#23869=CARTESIAN_POINT('Ctrl Pts',(-1.50980486807181,-1.,0.894452006967538));
#23870=CARTESIAN_POINT('Ctrl Pts',(-1.5055822144029,-1.,0.892032620296855));
#23871=CARTESIAN_POINT('',(-1.60662857109684,-1.,0.693717979106305));
#23872=CARTESIAN_POINT('Origin',(0.,-1.,0.));
#23873=CARTESIAN_POINT('',(-2.0698113262342,-1.,0.7455743247944));
#23874=CARTESIAN_POINT('Ctrl Pts',(-1.60662857109684,-1.,0.693717979106305));
#23875=CARTESIAN_POINT('Ctrl Pts',(-1.61106790957619,-1.,0.69571209787897));
#23876=CARTESIAN_POINT('Ctrl Pts',(-1.61974673471117,-1.,0.699605146398837));
#23877=CARTESIAN_POINT('Ctrl Pts',(-1.6321654166204,-1.,0.705159151977294));
#23878=CARTESIAN_POINT('Ctrl Pts',(-1.64752408828442,-1.,0.711993139340447));
#23879=CARTESIAN_POINT('Ctrl Pts',(-1.66472880551777,-1.,0.71958543378795));
#23880=CARTESIAN_POINT('Ctrl Pts',(-1.67996158451922,-1.,0.726235967982445));
#23881=CARTESIAN_POINT('Ctrl Pts',(-1.69326921972915,-1.,0.731963238685357));
#23882=CARTESIAN_POINT('Ctrl Pts',(-1.70473309004249,-1.,0.736799665716932));
#23883=CARTESIAN_POINT('Ctrl Pts',(-1.71447789751001,-1.,0.74079516202821));
#23884=CARTESIAN_POINT('Ctrl Pts',(-1.72268229916769,-1.,0.744021445433093));
#23885=CARTESIAN_POINT('Ctrl Pts',(-1.72958533647714,-1.,0.746574710097752));
#23886=CARTESIAN_POINT('Ctrl Pts',(-1.7355035168033,-1.,0.74858246295687));
#23887=CARTESIAN_POINT('Ctrl Pts',(-1.74080458267114,-1.,0.750193435981249));
#23888=CARTESIAN_POINT('Ctrl Pts',(-1.74585086852502,-1.,0.751555614164482));
#23889=CARTESIAN_POINT('Ctrl Pts',(-1.75095139468794,-1.,0.752797683531314));
#23890=CARTESIAN_POINT('Ctrl Pts',(-1.75631083600019,-1.,0.754009254027829));
#23891=CARTESIAN_POINT('Ctrl Pts',(-1.76197817240128,-1.,0.755220979974461));
#23892=CARTESIAN_POINT('Ctrl Pts',(-1.76789396002998,-1.,0.75642189602781));
#23893=CARTESIAN_POINT('Ctrl Pts',(-1.77394167108292,-1.,0.757578264077029));
#23894=CARTESIAN_POINT('Ctrl Pts',(-1.77999411220945,-1.,0.758650626677518));
#23895=CARTESIAN_POINT('Ctrl Pts',(-1.78596964884604,-1.,0.759614401110189));
#23896=CARTESIAN_POINT('Ctrl Pts',(-1.7918581561088,-1.,0.760469555880749));
#23897=CARTESIAN_POINT('Ctrl Pts',(-1.79768986997783,-1.,0.761229695230558));
#23898=CARTESIAN_POINT('Ctrl Pts',(-1.80351583877342,-1.,0.761915336443547));
#23899=CARTESIAN_POINT('Ctrl Pts',(-1.80938551463965,-1.,0.762546129463938));
#23900=CARTESIAN_POINT('Ctrl Pts',(-1.8153211840553,-1.,0.763132003836634));
#23901=CARTESIAN_POINT('Ctrl Pts',(-1.82131873145266,-1.,0.763673465462726));
#23902=CARTESIAN_POINT('Ctrl Pts',(-1.82735991200065,-1.,0.764165902605995));
#23903=CARTESIAN_POINT('Ctrl Pts',(-1.83342077227142,-1.,0.764602549687853));
#23904=CARTESIAN_POINT('Ctrl Pts',(-1.83948181064835,-1.,0.764978057881737));
#23905=CARTESIAN_POINT('Ctrl Pts',(-1.84553698875924,-1.,0.765291664862029));
#23906=CARTESIAN_POINT('Ctrl Pts',(-1.85158945130063,-1.,0.765545710619062));
#23907=CARTESIAN_POINT('Ctrl Pts',(-1.85764741390394,-1.,0.765744212909318));
#23908=CARTESIAN_POINT('Ctrl Pts',(-1.86372027063312,-1.,0.765891519092547));
#23909=CARTESIAN_POINT('Ctrl Pts',(-1.86981398314341,-1.,0.765990708546091));
#23910=CARTESIAN_POINT('Ctrl Pts',(-1.87592888967883,-1.,0.766042837036744));
#23911=CARTESIAN_POINT('Ctrl Pts',(-1.88206215302561,-1.,0.766047794851864));
#23912=CARTESIAN_POINT('Ctrl Pts',(-1.88820926433409,-1.,0.766004837062091));
#23913=CARTESIAN_POINT('Ctrl Pts',(-1.89436577771388,-1.,0.765913193856978));
#23914=CARTESIAN_POINT('Ctrl Pts',(-1.90052930393596,-1.,0.765772772593386));
#23915=CARTESIAN_POINT('Ctrl Pts',(-1.90669961402356,-1.,0.765584196937919));
#23916=CARTESIAN_POINT('Ctrl Pts',(-1.91287765805169,-1.,0.765348465884722));
#23917=CARTESIAN_POINT('Ctrl Pts',(-1.91906491634196,-1.,0.765066729667088));
#23918=CARTESIAN_POINT('Ctrl Pts',(-1.92526263537048,-1.,0.764740025488211));
#23919=CARTESIAN_POINT('Ctrl Pts',(-1.93147105496382,-1.,0.76436901067394));
#23920=CARTESIAN_POINT('Ctrl Pts',(-1.93768964875886,-1.,0.763954049121458));
#23921=CARTESIAN_POINT('Ctrl Pts',(-1.9439174661764,-1.,0.763495333538629));
#23922=CARTESIAN_POINT('Ctrl Pts',(-1.95015342590024,-1.,0.762992990878769));
#23923=CARTESIAN_POINT('Ctrl Pts',(-1.95639665309869,-1.,0.762447203806179));
#23924=CARTESIAN_POINT('Ctrl Pts',(-1.96264672744186,-1.,0.761858300014423));
#23925=CARTESIAN_POINT('Ctrl Pts',(-1.96890351582499,-1.,0.76122669048382));
#23926=CARTESIAN_POINT('Ctrl Pts',(-1.97516705321494,-1.,0.760552825409757));
#23927=CARTESIAN_POINT('Ctrl Pts',(-1.98143741418172,-1.,0.75983714745219));
#23928=CARTESIAN_POINT('Ctrl Pts',(-1.98771456680874,-1.,0.759080037802488));
#23929=CARTESIAN_POINT('Ctrl Pts',(-1.99399831098817,-1.,0.758281796766761));
#23930=CARTESIAN_POINT('Ctrl Pts',(-2.00028834739178,-1.,0.757442676862724));
#23931=CARTESIAN_POINT('Ctrl Pts',(-2.0065843158773,-1.,0.75656290464667));
#23932=CARTESIAN_POINT('Ctrl Pts',(-2.01288584328084,-1.,0.755642704957865));
#23933=CARTESIAN_POINT('Ctrl Pts',(-2.01919259405809,-1.,0.754682330722816));
#23934=CARTESIAN_POINT('Ctrl Pts',(-2.02550428623313,-1.,0.753682061112768));
#23935=CARTESIAN_POINT('Ctrl Pts',(-2.03182068456221,-1.,0.752642180487211));
#23936=CARTESIAN_POINT('Ctrl Pts',(-2.03814160092099,-1.,0.751562963361115));
#23937=CARTESIAN_POINT('Ctrl Pts',(-2.04446689147979,-1.,0.750444657875576));
#23938=CARTESIAN_POINT('Ctrl Pts',(-2.05079645592154,-1.,0.749287468665046));
#23939=CARTESIAN_POINT('Ctrl Pts',(-2.05713023031006,-1.,0.748091554183802));
#23940=CARTESIAN_POINT('Ctrl Pts',(-2.06220058927826,-1.,0.747103932787919));
#23941=CARTESIAN_POINT('Ctrl Pts',(-2.06600523016815,-1.,0.7463458715442));
#23942=CARTESIAN_POINT('Ctrl Pts',(-2.06854248895728,-1.,0.745832791378367));
#23943=CARTESIAN_POINT('Ctrl Pts',(-2.0698113262342,-1.,0.7455743247944));
#23944=CARTESIAN_POINT('',(-2.11275013067528,-1.,0.61342227326009));
#23945=CARTESIAN_POINT('',(-2.0698113262342,-1.,0.7455743247944));
#23946=CARTESIAN_POINT('',(-1.7075470150345,-1.,0.383122945602004));
#23947=CARTESIAN_POINT('Ctrl Pts',(-2.11275013067528,-1.,0.61342227326009));
#23948=CARTESIAN_POINT('Ctrl Pts',(-2.11187554259986,-1.,0.6124673655618));
#23949=CARTESIAN_POINT('Ctrl Pts',(-2.11012443807238,-1.,0.610560911689899));
#23950=CARTESIAN_POINT('Ctrl Pts',(-2.1074919961518,-1.,0.607711315454876));
#23951=CARTESIAN_POINT('Ctrl Pts',(-2.10397049886949,-1.,0.60393203073603));
#23952=CARTESIAN_POINT('Ctrl Pts',(-2.0995493086477,-1.,0.599241616420533));
#23953=CARTESIAN_POINT('Ctrl Pts',(-2.0951087622027,-1.,0.594585006052162));
#23954=CARTESIAN_POINT('Ctrl Pts',(-2.09064881812129,-1.,0.589962365403406));
#23955=CARTESIAN_POINT('Ctrl Pts',(-2.08616943727951,-1.,0.585373918991617));
#23956=CARTESIAN_POINT('Ctrl Pts',(-2.08167059018418,-1.,0.580819952108063));
#23957=CARTESIAN_POINT('Ctrl Pts',(-2.07715226767559,-1.,0.576300797416844));
#23958=CARTESIAN_POINT('Ctrl Pts',(-2.07261449292824,-1.,0.571816823242603));
#23959=CARTESIAN_POINT('Ctrl Pts',(-2.06805732997334,-1.,0.567368421181087));
#23960=CARTESIAN_POINT('Ctrl Pts',(-2.06348090160589,-1.,0.562955993082261));
#23961=CARTESIAN_POINT('Ctrl Pts',(-2.05888537756462,-1.,0.558579940185151));
#23962=CARTESIAN_POINT('Ctrl Pts',(-2.05427091604413,-1.,0.554240657463906));
#23963=CARTESIAN_POINT('Ctrl Pts',(-2.04963761077958,-1.,0.549938525150295));
#23964=CARTESIAN_POINT('Ctrl Pts',(-2.04498544714588,-1.,0.54567390381743));
#23965=CARTESIAN_POINT('Ctrl Pts',(-2.04031422690527,-1.,0.541447120615659));
#23966=CARTESIAN_POINT('Ctrl Pts',(-2.03562362954037,-1.,0.537258489833262));
#23967=CARTESIAN_POINT('Ctrl Pts',(-2.03091336214426,-1.,0.533108355132976));
#23968=CARTESIAN_POINT('Ctrl Pts',(-2.0261832908329,-1.,0.528997127241914));
#23969=CARTESIAN_POINT('Ctrl Pts',(-2.02143356304698,-1.,0.524925318333476));
#23970=CARTESIAN_POINT('Ctrl Pts',(-2.01666477917286,-1.,0.52089359039937));
#23971=CARTESIAN_POINT('Ctrl Pts',(-2.01187773939242,-1.,0.516902681728687));
#23972=CARTESIAN_POINT('Ctrl Pts',(-2.00707309946949,-1.,0.512953306961792));
#23973=CARTESIAN_POINT('Ctrl Pts',(-2.00225107134734,-1.,0.509046069886157));
#23974=CARTESIAN_POINT('Ctrl Pts',(-1.99741107463572,-1.,0.505181361323026));
#23975=CARTESIAN_POINT('Ctrl Pts',(-1.99255149126155,-1.,0.501359287727146));
#23976=CARTESIAN_POINT('Ctrl Pts',(-1.98767044752932,-1.,0.497579909545574));
#23977=CARTESIAN_POINT('Ctrl Pts',(-1.98276658761821,-1.,0.493843476541494));
#23978=CARTESIAN_POINT('Ctrl Pts',(-1.97783973019229,-1.,0.490150627860952));
#23979=CARTESIAN_POINT('Ctrl Pts',(-1.97289186263272,-1.,0.486502692907659));
#23980=CARTESIAN_POINT('Ctrl Pts',(-1.96792703422362,-1.,0.48290166212069));
#23981=CARTESIAN_POINT('Ctrl Pts',(-1.96294933055943,-1.,0.479349583074855));
#23982=CARTESIAN_POINT('Ctrl Pts',(-1.95796111148177,-1.,0.475848034683176));
#23983=CARTESIAN_POINT('Ctrl Pts',(-1.95296148278133,-1.,0.472397672264072));
#23984=CARTESIAN_POINT('Ctrl Pts',(-1.94794381136514,-1.,0.468997482913135));
#23985=CARTESIAN_POINT('Ctrl Pts',(-1.9428979419619,-1.,0.46564546202603));
#23986=CARTESIAN_POINT('Ctrl Pts',(-1.93781486640821,-1.,0.462340031009056));
#23987=CARTESIAN_POINT('Ctrl Pts',(-1.93269066517934,-1.,0.459081234547926));
#23988=CARTESIAN_POINT('Ctrl Pts',(-1.92753067150476,-1.,0.455872005174371));
#23989=CARTESIAN_POINT('Ctrl Pts',(-1.92235380648502,-1.,0.452719478359432));
#23990=CARTESIAN_POINT('Ctrl Pts',(-1.91718342555755,-1.,0.449632260106662));
#23991=CARTESIAN_POINT('Ctrl Pts',(-1.9120369998112,-1.,0.446617343485711));
#23992=CARTESIAN_POINT('Ctrl Pts',(-1.90691756144898,-1.,0.44367755684915));
#23993=CARTESIAN_POINT('Ctrl Pts',(-1.90180124389086,-1.,0.440807833704038));
#23994=CARTESIAN_POINT('Ctrl Pts',(-1.89663648956466,-1.,0.437995003948244));
#23995=CARTESIAN_POINT('Ctrl Pts',(-1.89136993975504,-1.,0.435225660963383));
#23996=CARTESIAN_POINT('Ctrl Pts',(-1.88596913666793,-1.,0.432493038548748));
#23997=CARTESIAN_POINT('Ctrl Pts',(-1.88044229001832,-1.,0.429803062482344));
#23998=CARTESIAN_POINT('Ctrl Pts',(-1.87486989291484,-1.,0.427183828519102));
#23999=CARTESIAN_POINT('Ctrl Pts',(-1.86937803944323,-1.,0.424678177291359));
#24000=CARTESIAN_POINT('Ctrl Pts',(-1.86408083334028,-1.,0.422327307418275));
#24001=CARTESIAN_POINT('Ctrl Pts',(-1.85903281096686,-1.,0.420157287975619));
#24002=CARTESIAN_POINT('Ctrl Pts',(-1.85417632856234,-1.,0.418164129143534));
#24003=CARTESIAN_POINT('Ctrl Pts',(-1.84929312929882,-1.,0.416300022038864));
#24004=CARTESIAN_POINT('Ctrl Pts',(-1.8440575707371,-1.,0.41448743825434));
#24005=CARTESIAN_POINT('Ctrl Pts',(-1.83808953475839,-1.,0.412633125322161));
#24006=CARTESIAN_POINT('Ctrl Pts',(-1.83100408895216,-1.,0.410641256301675));
#24007=CARTESIAN_POINT('Ctrl Pts',(-1.8224702267854,-1.,0.408428948108533));
#24008=CARTESIAN_POINT('Ctrl Pts',(-1.81223801813988,-1.,0.405933518411838));
#24009=CARTESIAN_POINT('Ctrl Pts',(-1.80012077176221,-1.,0.403107976170441));
#24010=CARTESIAN_POINT('Ctrl Pts',(-1.78598826347533,-1.,0.39991940378308));
#24011=CARTESIAN_POINT('Ctrl Pts',(-1.7697556004756,-1.,0.39634619612042));
#24012=CARTESIAN_POINT('Ctrl Pts',(-1.75137405313962,-1.,0.392375812294307));
#24013=CARTESIAN_POINT('Ctrl Pts',(-1.7349317097561,-1.,0.388877023509191));
#24014=CARTESIAN_POINT('Ctrl Pts',(-1.72162022246158,-1.,0.38607079032701));
#24015=CARTESIAN_POINT('Ctrl Pts',(-1.71231062891958,-1.,0.384119047315542));
#24016=CARTESIAN_POINT('Ctrl Pts',(-1.7075470150345,-1.,0.383122945602004));
#24017=CARTESIAN_POINT('',(-1.74236521665491,-1.,0.163289472382896));
#24018=CARTESIAN_POINT('Origin',(0.,-1.,0.));
#24019=CARTESIAN_POINT('',(-2.19890268624765,-1.,0.069476445021958));
#24020=CARTESIAN_POINT('Ctrl Pts',(-1.74236521665491,-1.,0.163289472382896));
#24021=CARTESIAN_POINT('Ctrl Pts',(-1.7472034950333,-1.,0.163814161002002));
#24022=CARTESIAN_POINT('Ctrl Pts',(-1.75666056638427,-1.,0.164834765707158));
#24023=CARTESIAN_POINT('Ctrl Pts',(-1.77018771684844,-1.,0.1662793551464));
#24024=CARTESIAN_POINT('Ctrl Pts',(-1.7869064998507,-1.,0.168032772805197));
#24025=CARTESIAN_POINT('Ctrl Pts',(-1.80561530629706,-1.,0.169936923904608));
#24026=CARTESIAN_POINT('Ctrl Pts',(-1.82215766811545,-1.,0.171554770204119));
#24027=CARTESIAN_POINT('Ctrl Pts',(-1.83658380527692,-1.,0.1728894428919));
#24028=CARTESIAN_POINT('Ctrl Pts',(-1.8489811319852,-1.,0.173946627587731));
#24029=CARTESIAN_POINT('Ctrl Pts',(-1.85948367088837,-1.,0.17473525927603));
#24030=CARTESIAN_POINT('Ctrl Pts',(-1.86828349694799,-1.,0.175268337590758));
#24031=CARTESIAN_POINT('Ctrl Pts',(-1.87563767773588,-1.,0.175563480746485));
#24032=CARTESIAN_POINT('Ctrl Pts',(-1.88188663145367,-1.,0.175644148889698));
#24033=CARTESIAN_POINT('Ctrl Pts',(-1.88742606273259,-1.,0.175538155840648));
#24034=CARTESIAN_POINT('Ctrl Pts',(-1.892646301985,-1.,0.175274276190844));
#24035=CARTESIAN_POINT('Ctrl Pts',(-1.89788101117132,-1.,0.174879405091263));
#24036=CARTESIAN_POINT('Ctrl Pts',(-1.90335253862834,-1.,0.174375518661085));
#24037=CARTESIAN_POINT('Ctrl Pts',(-1.90911693975267,-1.,0.173776635257817));
#24038=CARTESIAN_POINT('Ctrl Pts',(-1.91511429159527,-1.,0.173090695383496));
#24039=CARTESIAN_POINT('Ctrl Pts',(-1.9212233439798,-1.,0.172321621259514));
#24040=CARTESIAN_POINT('Ctrl Pts',(-1.92731093582036,-1.,0.171471191532988));
#24041=CARTESIAN_POINT('Ctrl Pts',(-1.93329183155539,-1.,0.170541253116201));
#24042=CARTESIAN_POINT('Ctrl Pts',(-1.93915639211581,-1.,0.169534904817491));
#24043=CARTESIAN_POINT('Ctrl Pts',(-1.94493757756931,-1.,0.168455741607556));
#24044=CARTESIAN_POINT('Ctrl Pts',(-1.95069027794294,-1.,0.167307501784475));
#24045=CARTESIAN_POINT('Ctrl Pts',(-1.9564675971873,-1.,0.166093592002812));
#24046=CARTESIAN_POINT('Ctrl Pts',(-1.96229379940136,-1.,0.164816568920269));
#24047=CARTESIAN_POINT('Ctrl Pts',(-1.96816512677967,-1.,0.163478185457734));
#24048=CARTESIAN_POINT('Ctrl Pts',(-1.97406280235188,-1.,0.162079693556288));
#24049=CARTESIAN_POINT('Ctrl Pts',(-1.97996195437559,-1.,0.160622060784611));
#24050=CARTESIAN_POINT('Ctrl Pts',(-1.98584238283292,-1.,0.159106226437299));
#24051=CARTESIAN_POINT('Ctrl Pts',(-1.99169810931908,-1.,0.157533331459227));
#24052=CARTESIAN_POINT('Ctrl Pts',(-1.99753284771497,-1.,0.155904629548783));
#24053=CARTESIAN_POINT('Ctrl Pts',(-2.00335565310543,-1.,0.154221403049722));
#24054=CARTESIAN_POINT('Ctrl Pts',(-2.00917680318424,-1.,0.15248488362145));
#24055=CARTESIAN_POINT('Ctrl Pts',(-2.01500291940238,-1.,0.150696157673078));
#24056=CARTESIAN_POINT('Ctrl Pts',(-2.02083464969894,-1.,0.148856124775337));
#24057=CARTESIAN_POINT('Ctrl Pts',(-2.02666926182017,-1.,0.146965557332583));
#24058=CARTESIAN_POINT('Ctrl Pts',(-2.03250223739942,-1.,0.145025140186057));
#24059=CARTESIAN_POINT('Ctrl Pts',(-2.03832911025912,-1.,0.143035515058209));
#24060=CARTESIAN_POINT('Ctrl Pts',(-2.04414757947916,-1.,0.140997332152546));
#24061=CARTESIAN_POINT('Ctrl Pts',(-2.04995762001328,-1.,0.138911255368966));
#24062=CARTESIAN_POINT('Ctrl Pts',(-2.05576044414264,-1.,0.136777941218043));
#24063=CARTESIAN_POINT('Ctrl Pts',(-2.06155781517842,-1.,0.134598026192106));
#24064=CARTESIAN_POINT('Ctrl Pts',(-2.06735123910326,-1.,0.13237211154771));
#24065=CARTESIAN_POINT('Ctrl Pts',(-2.07314114713063,-1.,0.130100748328403));
#24066=CARTESIAN_POINT('Ctrl Pts',(-2.07892715110987,-1.,0.12778444527612));
#24067=CARTESIAN_POINT('Ctrl Pts',(-2.08470840653643,-1.,0.125423679412061));
#24068=CARTESIAN_POINT('Ctrl Pts',(-2.09048392424825,-1.,0.123018905621083));
#24069=CARTESIAN_POINT('Ctrl Pts',(-2.0962529286773,-1.,0.120570567965122));
#24070=CARTESIAN_POINT('Ctrl Pts',(-2.102015121329,-1.,0.118079107988355));
#24071=CARTESIAN_POINT('Ctrl Pts',(-2.10777050261309,-1.,0.115544957687926));
#24072=CARTESIAN_POINT('Ctrl Pts',(-2.11351924490306,-1.,0.112968534419737));
#24073=CARTESIAN_POINT('Ctrl Pts',(-2.11926155590865,-1.,0.110350236135025));
#24074=CARTESIAN_POINT('Ctrl Pts',(-2.12499752307,-1.,0.10769043523109));
#24075=CARTESIAN_POINT('Ctrl Pts',(-2.13072704887293,-1.,0.104989479152739));
#24076=CARTESIAN_POINT('Ctrl Pts',(-2.13644992667165,-1.,0.1022477005561));
#24077=CARTESIAN_POINT('Ctrl Pts',(-2.14216588396025,-1.,0.0994654261990914));
#24078=CARTESIAN_POINT('Ctrl Pts',(-2.14787463531795,-1.,0.0966429852305457));
#24079=CARTESIAN_POINT('Ctrl Pts',(-2.1535759397817,-1.,0.0937807218867642));
#24080=CARTESIAN_POINT('Ctrl Pts',(-2.15926961544516,-1.,0.0908789888107264));
#24081=CARTESIAN_POINT('Ctrl Pts',(-2.16495552645014,-1.,0.0879381291386921));
#24082=CARTESIAN_POINT('Ctrl Pts',(-2.17063357870952,-1.,0.0849584620835371));
#24083=CARTESIAN_POINT('Ctrl Pts',(-2.176303712113,-1.,0.0819402680872764));
#24084=CARTESIAN_POINT('Ctrl Pts',(-2.18196589448887,-1.,0.0788837727685241));
#24085=CARTESIAN_POINT('Ctrl Pts',(-2.1876201139953,-1.,0.0757891465836146));
#24086=CARTESIAN_POINT('Ctrl Pts',(-2.19213712013662,-1.,0.0732830357306724));
#24087=CARTESIAN_POINT('Ctrl Pts',(-2.19552129484002,-1.,0.0713863779526153));
#24088=CARTESIAN_POINT('Ctrl Pts',(-2.19777582085423,-1.,0.0701143536325489));
#24089=CARTESIAN_POINT('Ctrl Pts',(-2.19890268624765,-1.,0.069476445021958));
#24090=CARTESIAN_POINT('',(-2.19890268624765,-1.,-0.0694764450219585));
#24091=CARTESIAN_POINT('',(-2.19890268624765,-1.,0.069476445021958));
#24092=CARTESIAN_POINT('',(-1.74236521665491,-1.,-0.163289472382896));
#24093=CARTESIAN_POINT('Ctrl Pts',(-2.19890268624765,-1.,-0.0694764450219585));
#24094=CARTESIAN_POINT('Ctrl Pts',(-2.19777582085261,-1.,-0.0701143536324927));
#24095=CARTESIAN_POINT('Ctrl Pts',(-2.19552129483562,-1.,-0.0713863779524629));
#24096=CARTESIAN_POINT('Ctrl Pts',(-2.19213712012956,-1.,-0.0732830357304277));
#24097=CARTESIAN_POINT('Ctrl Pts',(-2.1876201139874,-1.,-0.0757891465833413));
#24098=CARTESIAN_POINT('Ctrl Pts',(-2.18196589448304,-1.,-0.0788837727683229));
#24099=CARTESIAN_POINT('Ctrl Pts',(-2.1763037121106,-1.,-0.0819402680871941));
#24100=CARTESIAN_POINT('Ctrl Pts',(-2.17063357871031,-1.,-0.0849584620835644));
#24101=CARTESIAN_POINT('Ctrl Pts',(-2.16495552645275,-1.,-0.0879381291387824));
#24102=CARTESIAN_POINT('Ctrl Pts',(-2.15926961544808,-1.,-0.0908789888108267));
#24103=CARTESIAN_POINT('Ctrl Pts',(-2.15357593978377,-1.,-0.0937807218868346));
#24104=CARTESIAN_POINT('Ctrl Pts',(-2.14787463531864,-1.,-0.096642985230569));
#24105=CARTESIAN_POINT('Ctrl Pts',(-2.14216588395974,-1.,-0.0994654261990744));
#24106=CARTESIAN_POINT('Ctrl Pts',(-2.13644992667052,-1.,-0.102247700556064));
#24107=CARTESIAN_POINT('Ctrl Pts',(-2.1307270488718,-1.,-0.104989479152703));
#24108=CARTESIAN_POINT('Ctrl Pts',(-2.12499752306927,-1.,-0.107690435231068));
#24109=CARTESIAN_POINT('Ctrl Pts',(-2.11926155590849,-1.,-0.11035023613502));
#24110=CARTESIAN_POINT('Ctrl Pts',(-2.11351924490335,-1.,-0.112968534419746));
#24111=CARTESIAN_POINT('Ctrl Pts',(-2.10777050261359,-1.,-0.11554495768794));
#24112=CARTESIAN_POINT('Ctrl Pts',(-2.10201512132945,-1.,-0.118079107988368));
#24113=CARTESIAN_POINT('Ctrl Pts',(-2.09625292867756,-1.,-0.120570567965129));
#24114=CARTESIAN_POINT('Ctrl Pts',(-2.09048392424826,-1.,-0.123018905621083));
#24115=CARTESIAN_POINT('Ctrl Pts',(-2.08470840653628,-1.,-0.125423679412058));
#24116=CARTESIAN_POINT('Ctrl Pts',(-2.07892715110967,-1.,-0.127784445276116));
#24117=CARTESIAN_POINT('Ctrl Pts',(-2.07314114713047,-1.,-0.130100748328401));
#24118=CARTESIAN_POINT('Ctrl Pts',(-2.06735123910319,-1.,-0.13237211154771));
#24119=CARTESIAN_POINT('Ctrl Pts',(-2.06155781517844,-1.,-0.134598026192107));
#24120=CARTESIAN_POINT('Ctrl Pts',(-2.0557604441427,-1.,-0.136777941218044));
#24121=CARTESIAN_POINT('Ctrl Pts',(-2.04995762001333,-1.,-0.138911255368966));
#24122=CARTESIAN_POINT('Ctrl Pts',(-2.04414757947919,-1.,-0.140997332152545));
#24123=CARTESIAN_POINT('Ctrl Pts',(-2.03832911025913,-1.,-0.143035515058208));
#24124=CARTESIAN_POINT('Ctrl Pts',(-2.03250223739941,-1.,-0.145025140186058));
#24125=CARTESIAN_POINT('Ctrl Pts',(-2.02666926182017,-1.,-0.146965557332586));
#24126=CARTESIAN_POINT('Ctrl Pts',(-2.02083464969897,-1.,-0.148856124775343));
#24127=CARTESIAN_POINT('Ctrl Pts',(-2.01500291940243,-1.,-0.150696157673084));
#24128=CARTESIAN_POINT('Ctrl Pts',(-2.00917680318426,-1.,-0.152484883621452));
#24129=CARTESIAN_POINT('Ctrl Pts',(-2.00335565310539,-1.,-0.154221403049719));
#24130=CARTESIAN_POINT('Ctrl Pts',(-1.99753284771487,-1.,-0.155904629548775));
#24131=CARTESIAN_POINT('Ctrl Pts',(-1.99169810931893,-1.,-0.157533331459215));
#24132=CARTESIAN_POINT('Ctrl Pts',(-1.98584238283279,-1.,-0.159106226437289));
#24133=CARTESIAN_POINT('Ctrl Pts',(-1.97996195437557,-1.,-0.16062206078461));
#24134=CARTESIAN_POINT('Ctrl Pts',(-1.97406280235204,-1.,-0.162079693556302));
#24135=CARTESIAN_POINT('Ctrl Pts',(-1.96816512678,-1.,-0.16347818545776));
#24136=CARTESIAN_POINT('Ctrl Pts',(-1.96229379940174,-1.,-0.1648165689203));
#24137=CARTESIAN_POINT('Ctrl Pts',(-1.95646759718755,-1.,-0.166093592002833));
#24138=CARTESIAN_POINT('Ctrl Pts',(-1.95069027794286,-1.,-0.167307501784469));
#24139=CARTESIAN_POINT('Ctrl Pts',(-1.94493757756879,-1.,-0.168455741607516));
#24140=CARTESIAN_POINT('Ctrl Pts',(-1.93915639211497,-1.,-0.169534904817425));
#24141=CARTESIAN_POINT('Ctrl Pts',(-1.93329183155455,-1.,-0.170541253116136));
#24142=CARTESIAN_POINT('Ctrl Pts',(-1.92731093582,-1.,-0.17147119153296));
#24143=CARTESIAN_POINT('Ctrl Pts',(-1.92122334398034,-1.,-0.172321621259557));
#24144=CARTESIAN_POINT('Ctrl Pts',(-1.91511429159681,-1.,-0.173090695383619));
#24145=CARTESIAN_POINT('Ctrl Pts',(-1.90911693975475,-1.,-0.173776635257984));
#24146=CARTESIAN_POINT('Ctrl Pts',(-1.90335253863003,-1.,-0.174375518661222));
#24147=CARTESIAN_POINT('Ctrl Pts',(-1.89788101117148,-1.,-0.174879405091277));
#24148=CARTESIAN_POINT('Ctrl Pts',(-1.89264630198279,-1.,-0.175274276190664));
#24149=CARTESIAN_POINT('Ctrl Pts',(-1.88742606272818,-1.,-0.175538155840286));
#24150=CARTESIAN_POINT('Ctrl Pts',(-1.88188663144846,-1.,-0.175644148889271));
#24151=CARTESIAN_POINT('Ctrl Pts',(-1.87563767773249,-1.,-0.175563480746205));
#24152=CARTESIAN_POINT('Ctrl Pts',(-1.86828349694972,-1.,-0.175268337590901));
#24153=CARTESIAN_POINT('Ctrl Pts',(-1.85948367089838,-1.,-0.174735259276856));
#24154=CARTESIAN_POINT('Ctrl Pts',(-1.84898113200543,-1.,-0.173946627589401));
#24155=CARTESIAN_POINT('Ctrl Pts',(-1.83658380530747,-1.,-0.17288944289442));
#24156=CARTESIAN_POINT('Ctrl Pts',(-1.82215766815414,-1.,-0.171554770207306));
#24157=CARTESIAN_POINT('Ctrl Pts',(-1.80561530633924,-1.,-0.169936923908078));
#24158=CARTESIAN_POINT('Ctrl Pts',(-1.78690649988931,-1.,-0.16803277280837));
#24159=CARTESIAN_POINT('Ctrl Pts',(-1.77018771687692,-1.,-0.166279355148738));
#24160=CARTESIAN_POINT('Ctrl Pts',(-1.75666056640041,-1.,-0.164834765708484));
#24161=CARTESIAN_POINT('Ctrl Pts',(-1.74720349503904,-1.,-0.163814161002474));
#24162=CARTESIAN_POINT('Ctrl Pts',(-1.74236521665491,-1.,-0.163289472382896));
#24163=CARTESIAN_POINT('',(-1.7075470150345,-1.,-0.383122945602004));
#24164=CARTESIAN_POINT('Origin',(0.,-1.,0.));
#24165=CARTESIAN_POINT('',(-2.11275013067528,-1.,-0.61342227326009));
#24166=CARTESIAN_POINT('Ctrl Pts',(-1.7075470150345,-1.,-0.383122945602004));
#24167=CARTESIAN_POINT('Ctrl Pts',(-1.71231062891398,-1.,-0.384119047314215));
#24168=CARTESIAN_POINT('Ctrl Pts',(-1.72162022244582,-1.,-0.386070790323281));
#24169=CARTESIAN_POINT('Ctrl Pts',(-1.73493170972829,-1.,-0.388877023502615));
#24170=CARTESIAN_POINT('Ctrl Pts',(-1.75137405310193,-1.,-0.392375812285395));
#24171=CARTESIAN_POINT('Ctrl Pts',(-1.76975560043442,-1.,-0.396346196110688));
#24172=CARTESIAN_POINT('Ctrl Pts',(-1.78598826343754,-1.,-0.399919403774155));
#24173=CARTESIAN_POINT('Ctrl Pts',(-1.80012077173238,-1.,-0.403107976163396));
#24174=CARTESIAN_POINT('Ctrl Pts',(-1.81223801812013,-1.,-0.405933518407175));
#24175=CARTESIAN_POINT('Ctrl Pts',(-1.82247022677562,-1.,-0.408428948106227));
#24176=CARTESIAN_POINT('Ctrl Pts',(-1.83100408895047,-1.,-0.410641256301276));
#24177=CARTESIAN_POINT('Ctrl Pts',(-1.8380895347617,-1.,-0.412633125322945));
#24178=CARTESIAN_POINT('Ctrl Pts',(-1.84405757074218,-1.,-0.414487438255542));
#24179=CARTESIAN_POINT('Ctrl Pts',(-1.84929312930314,-1.,-0.416300022039885));
#24180=CARTESIAN_POINT('Ctrl Pts',(-1.8541763285645,-1.,-0.418164129144045));
#24181=CARTESIAN_POINT('Ctrl Pts',(-1.8590328109667,-1.,-0.420157287975583));
#24182=CARTESIAN_POINT('Ctrl Pts',(-1.86408083333863,-1.,-0.422327307417884));
#24183=CARTESIAN_POINT('Ctrl Pts',(-1.8693780394412,-1.,-0.424678177290876));
#24184=CARTESIAN_POINT('Ctrl Pts',(-1.87486989291333,-1.,-0.427183828518743));
#24185=CARTESIAN_POINT('Ctrl Pts',(-1.88044229001778,-1.,-0.429803062482217));
#24186=CARTESIAN_POINT('Ctrl Pts',(-1.88596913666828,-1.,-0.432493038548833));
#24187=CARTESIAN_POINT('Ctrl Pts',(-1.89136993975585,-1.,-0.43522566096358));
#24188=CARTESIAN_POINT('Ctrl Pts',(-1.89663648956549,-1.,-0.437995003948443));
#24189=CARTESIAN_POINT('Ctrl Pts',(-1.90180124389137,-1.,-0.44080783370416));
#24190=CARTESIAN_POINT('Ctrl Pts',(-1.90691756144906,-1.,-0.44367755684917));
#24191=CARTESIAN_POINT('Ctrl Pts',(-1.91203699981095,-1.,-0.446617343485651));
#24192=CARTESIAN_POINT('Ctrl Pts',(-1.91718342555717,-1.,-0.449632260106572));
#24193=CARTESIAN_POINT('Ctrl Pts',(-1.9223538064847,-1.,-0.452719478359356));
#24194=CARTESIAN_POINT('Ctrl Pts',(-1.92753067150461,-1.,-0.455872005174335));
#24195=CARTESIAN_POINT('Ctrl Pts',(-1.93269066517936,-1.,-0.459081234547931));
#24196=CARTESIAN_POINT('Ctrl Pts',(-1.93781486640834,-1.,-0.462340031009087));
#24197=CARTESIAN_POINT('Ctrl Pts',(-1.94289794196205,-1.,-0.465645462026064));
#24198=CARTESIAN_POINT('Ctrl Pts',(-1.94794381136524,-1.,-0.468997482913158));
#24199=CARTESIAN_POINT('Ctrl Pts',(-1.95296148278136,-1.,-0.472397672264079));
#24200=CARTESIAN_POINT('Ctrl Pts',(-1.95796111148175,-1.,-0.475848034683171));
#24201=CARTESIAN_POINT('Ctrl Pts',(-1.96294933055938,-1.,-0.479349583074846));
#24202=CARTESIAN_POINT('Ctrl Pts',(-1.96792703422358,-1.,-0.482901662120686));
#24203=CARTESIAN_POINT('Ctrl Pts',(-1.97289186263272,-1.,-0.486502692907661));
#24204=CARTESIAN_POINT('Ctrl Pts',(-1.97783973019229,-1.,-0.490150627860955));
#24205=CARTESIAN_POINT('Ctrl Pts',(-1.9827665876182,-1.,-0.493843476541492));
#24206=CARTESIAN_POINT('Ctrl Pts',(-1.98767044752929,-1.,-0.497579909545564));
#24207=CARTESIAN_POINT('Ctrl Pts',(-1.9925514912615,-1.,-0.501359287727129));
#24208=CARTESIAN_POINT('Ctrl Pts',(-1.99741107463567,-1.,-0.505181361323011));
#24209=CARTESIAN_POINT('Ctrl Pts',(-2.00225107134733,-1.,-0.509046069886152));
#24210=CARTESIAN_POINT('Ctrl Pts',(-2.00707309946955,-1.,-0.512953306961813));
#24211=CARTESIAN_POINT('Ctrl Pts',(-2.01187773939257,-1.,-0.516902681728733));
#24212=CARTESIAN_POINT('Ctrl Pts',(-2.01666477917305,-1.,-0.520893590399428));
#24213=CARTESIAN_POINT('Ctrl Pts',(-2.02143356304712,-1.,-0.524925318333518));
#24214=CARTESIAN_POINT('Ctrl Pts',(-2.02618329083289,-1.,-0.52899712724191));
#24215=CARTESIAN_POINT('Ctrl Pts',(-2.03091336214401,-1.,-0.533108355132905));
#24216=CARTESIAN_POINT('Ctrl Pts',(-2.03562362953993,-1.,-0.537258489833134));
#24217=CARTESIAN_POINT('Ctrl Pts',(-2.0403142269048,-1.,-0.54144712061552));
#24218=CARTESIAN_POINT('Ctrl Pts',(-2.0449854471456,-1.,-0.545673903817348));
#24219=CARTESIAN_POINT('Ctrl Pts',(-2.04963761077974,-1.,-0.549938525150342));
#24220=CARTESIAN_POINT('Ctrl Pts',(-2.05427091604482,-1.,-0.554240657464109));
#24221=CARTESIAN_POINT('Ctrl Pts',(-2.05888537756571,-1.,-0.558579940185467));
#24222=CARTESIAN_POINT('Ctrl Pts',(-2.06348090160697,-1.,-0.562955993082574));
#24223=CARTESIAN_POINT('Ctrl Pts',(-2.06805732997383,-1.,-0.567368421181229));
#24224=CARTESIAN_POINT('Ctrl Pts',(-2.07261449292757,-1.,-0.571816823242411));
#24225=CARTESIAN_POINT('Ctrl Pts',(-2.07715226767361,-1.,-0.576300797416274));
#24226=CARTESIAN_POINT('Ctrl Pts',(-2.08167059018138,-1.,-0.580819952107257));
#24227=CARTESIAN_POINT('Ctrl Pts',(-2.086169437277,-1.,-0.585373918990895));
#24228=CARTESIAN_POINT('Ctrl Pts',(-2.09064881812053,-1.,-0.589962365403189));
#24229=CARTESIAN_POINT('Ctrl Pts',(-2.09510876220501,-1.,-0.594585006052823));
#24230=CARTESIAN_POINT('Ctrl Pts',(-2.09954930865331,-1.,-0.599241616422144));
#24231=CARTESIAN_POINT('Ctrl Pts',(-2.10397049887709,-1.,-0.603932030738212));
#24232=CARTESIAN_POINT('Ctrl Pts',(-2.10749199615859,-1.,-0.607711315456826));
#24233=CARTESIAN_POINT('Ctrl Pts',(-2.11012443807661,-1.,-0.610560911691113));
#24234=CARTESIAN_POINT('Ctrl Pts',(-2.11187554260142,-1.,-0.61246736556225));
#24235=CARTESIAN_POINT('Ctrl Pts',(-2.11275013067528,-1.,-0.61342227326009));
#24236=CARTESIAN_POINT('',(-2.0698113262342,-1.,-0.745574324794401));
#24237=CARTESIAN_POINT('',(-2.11275013067528,-1.,-0.61342227326009));
#24238=CARTESIAN_POINT('',(-1.60662857109684,-1.,-0.693717979106306));
#24239=CARTESIAN_POINT('Ctrl Pts',(-2.0698113262342,-1.,-0.745574324794401));
#24240=CARTESIAN_POINT('Ctrl Pts',(-2.06854248895575,-1.,-0.74583279137781));
#24241=CARTESIAN_POINT('Ctrl Pts',(-2.06600523016401,-1.,-0.746345871542695));
#24242=CARTESIAN_POINT('Ctrl Pts',(-2.06220058927162,-1.,-0.747103932785504));
#24243=CARTESIAN_POINT('Ctrl Pts',(-2.05713023030263,-1.,-0.748091554181101));
#24244=CARTESIAN_POINT('Ctrl Pts',(-2.05079645591606,-1.,-0.749287468663053));
#24245=CARTESIAN_POINT('Ctrl Pts',(-2.04446689147754,-1.,-0.750444657874758));
#24246=CARTESIAN_POINT('Ctrl Pts',(-2.03814160092173,-1.,-0.751562963361383));
#24247=CARTESIAN_POINT('Ctrl Pts',(-2.03182068456467,-1.,-0.752642180488104));
#24248=CARTESIAN_POINT('Ctrl Pts',(-2.02550428623587,-1.,-0.753682061113765));
#24249=CARTESIAN_POINT('Ctrl Pts',(-2.01919259406003,-1.,-0.75468233072352));
#24250=CARTESIAN_POINT('Ctrl Pts',(-2.01288584328149,-1.,-0.7556427049581));
#24251=CARTESIAN_POINT('Ctrl Pts',(-2.00658431587682,-1.,-0.756562904646496));
#24252=CARTESIAN_POINT('Ctrl Pts',(-2.00028834739072,-1.,-0.757442676862341));
#24253=CARTESIAN_POINT('Ctrl Pts',(-1.9939983109871,-1.,-0.758281796766377));
#24254=CARTESIAN_POINT('Ctrl Pts',(-1.98771456680806,-1.,-0.759080037802242));
#24255=CARTESIAN_POINT('Ctrl Pts',(-1.98143741418156,-1.,-0.759837147452135));
#24256=CARTESIAN_POINT('Ctrl Pts',(-1.97516705321521,-1.,-0.760552825409855));
#24257=CARTESIAN_POINT('Ctrl Pts',(-1.96890351582545,-1.,-0.761226690483986));
#24258=CARTESIAN_POINT('Ctrl Pts',(-1.96264672744229,-1.,-0.761858300014575));
#24259=CARTESIAN_POINT('Ctrl Pts',(-1.95639665309893,-1.,-0.762447203806263));
#24260=CARTESIAN_POINT('Ctrl Pts',(-1.95015342590025,-1.,-0.762992990878774));
#24261=CARTESIAN_POINT('Ctrl Pts',(-1.94391746617626,-1.,-0.76349533353858));
#24262=CARTESIAN_POINT('Ctrl Pts',(-1.93768964875867,-1.,-0.763954049121393));
#24263=CARTESIAN_POINT('Ctrl Pts',(-1.93147105496367,-1.,-0.764369010673889));
#24264=CARTESIAN_POINT('Ctrl Pts',(-1.92526263537041,-1.,-0.764740025488189));
#24265=CARTESIAN_POINT('Ctrl Pts',(-1.91906491634197,-1.,-0.765066729667095));
#24266=CARTESIAN_POINT('Ctrl Pts',(-1.91287765805174,-1.,-0.765348465884739));
#24267=CARTESIAN_POINT('Ctrl Pts',(-1.90669961402362,-1.,-0.765584196937936));
#24268=CARTESIAN_POINT('Ctrl Pts',(-1.90052930393599,-1.,-0.765772772593395));
#24269=CARTESIAN_POINT('Ctrl Pts',(-1.89436577771389,-1.,-0.765913193856979));
#24270=CARTESIAN_POINT('Ctrl Pts',(-1.88820926433409,-1.,-0.76600483706209));
#24271=CARTESIAN_POINT('Ctrl Pts',(-1.88206215302561,-1.,-0.766047794851868));
#24272=CARTESIAN_POINT('Ctrl Pts',(-1.87592888967886,-1.,-0.766042837036759));
#24273=CARTESIAN_POINT('Ctrl Pts',(-1.86981398314345,-1.,-0.765990708546111));
#24274=CARTESIAN_POINT('Ctrl Pts',(-1.86372027063314,-1.,-0.765891519092557));
#24275=CARTESIAN_POINT('Ctrl Pts',(-1.85764741390391,-1.,-0.765744212909305));
#24276=CARTESIAN_POINT('Ctrl Pts',(-1.85158945130054,-1.,-0.765545710619023));
#24277=CARTESIAN_POINT('Ctrl Pts',(-1.8455369887591,-1.,-0.765291664861971));
#24278=CARTESIAN_POINT('Ctrl Pts',(-1.83948181064823,-1.,-0.764978057881687));
#24279=CARTESIAN_POINT('Ctrl Pts',(-1.8334207722714,-1.,-0.764602549687845));
#24280=CARTESIAN_POINT('Ctrl Pts',(-1.8273599120008,-1.,-0.764165902606055));
#24281=CARTESIAN_POINT('Ctrl Pts',(-1.82131873145297,-1.,-0.763673465462854));
#24282=CARTESIAN_POINT('Ctrl Pts',(-1.81532118405566,-1.,-0.763132003836783));
#24283=CARTESIAN_POINT('Ctrl Pts',(-1.80938551463989,-1.,-0.762546129464036));
#24284=CARTESIAN_POINT('Ctrl Pts',(-1.80351583877334,-1.,-0.761915336443515));
#24285=CARTESIAN_POINT('Ctrl Pts',(-1.79768986997735,-1.,-0.761229695230359));
#24286=CARTESIAN_POINT('Ctrl Pts',(-1.79185815610802,-1.,-0.760469555880425));
#24287=CARTESIAN_POINT('Ctrl Pts',(-1.78596964884526,-1.,-0.759614401109868));
#24288=CARTESIAN_POINT('Ctrl Pts',(-1.77999411220912,-1.,-0.75865062667738));
#24289=CARTESIAN_POINT('Ctrl Pts',(-1.77394167108342,-1.,-0.757578264077238));
#24290=CARTESIAN_POINT('Ctrl Pts',(-1.76789396003141,-1.,-0.756421896028403));
#24291=CARTESIAN_POINT('Ctrl Pts',(-1.7619781724032,-1.,-0.755220979975262));
#24292=CARTESIAN_POINT('Ctrl Pts',(-1.75631083600175,-1.,-0.75400925402848));
#24293=CARTESIAN_POINT('Ctrl Pts',(-1.75095139468809,-1.,-0.752797683531377));
#24294=CARTESIAN_POINT('Ctrl Pts',(-1.74585086852298,-1.,-0.751555614163629));
#24295=CARTESIAN_POINT('Ctrl Pts',(-1.74080458266705,-1.,-0.75019343597954));
#24296=CARTESIAN_POINT('Ctrl Pts',(-1.73550351679848,-1.,-0.748582462954854));
#24297=CARTESIAN_POINT('Ctrl Pts',(-1.72958533647399,-1.,-0.746574710096436));
#24298=CARTESIAN_POINT('Ctrl Pts',(-1.7226822991693,-1.,-0.744021445433764));
#24299=CARTESIAN_POINT('Ctrl Pts',(-1.71447789751927,-1.,-0.740795162032087));
#24300=CARTESIAN_POINT('Ctrl Pts',(-1.70473309006121,-1.,-0.736799665724771));
#24301=CARTESIAN_POINT('Ctrl Pts',(-1.69326921975743,-1.,-0.731963238697195));
#24302=CARTESIAN_POINT('Ctrl Pts',(-1.67996158455503,-1.,-0.726235967997433));
#24303=CARTESIAN_POINT('Ctrl Pts',(-1.6647288055568,-1.,-0.719585433804282));
#24304=CARTESIAN_POINT('Ctrl Pts',(-1.64752408832016,-1.,-0.711993139355394));
#24305=CARTESIAN_POINT('Ctrl Pts',(-1.63216541664676,-1.,-0.705159151988319));
#24306=CARTESIAN_POINT('Ctrl Pts',(-1.61974673472612,-1.,-0.699605146405088));
#24307=CARTESIAN_POINT('Ctrl Pts',(-1.61106790958151,-1.,-0.695712097881194));
#24308=CARTESIAN_POINT('Ctrl Pts',(-1.60662857109684,-1.,-0.693717979106306));
#24309=CARTESIAN_POINT('',(-1.5055822144029,-1.,-0.892032620296855));
#24310=CARTESIAN_POINT('Origin',(0.,-1.,0.));
#24311=CARTESIAN_POINT('',(-1.81978687191668,-1.,-1.23627494547115));
#24312=CARTESIAN_POINT('Ctrl Pts',(-1.5055822144029,-1.,-0.892032620296855));
#24313=CARTESIAN_POINT('Ctrl Pts',(-1.50980486806688,-1.,-0.894452006964543));
#24314=CARTESIAN_POINT('Ctrl Pts',(-1.51805569590094,-1.,-0.899185047483511));
#24315=CARTESIAN_POINT('Ctrl Pts',(-1.52984849887993,-1.,-0.905967409625651));
#24316=CARTESIAN_POINT('Ctrl Pts',(-1.54440491149498,-1.,-0.914375919026456));
#24317=CARTESIAN_POINT('Ctrl Pts',(-1.56065988578893,-1.,-0.923832188944341));
#24318=CARTESIAN_POINT('Ctrl Pts',(-1.57499388382243,-1.,-0.932246680108685));
#24319=CARTESIAN_POINT('Ctrl Pts',(-1.58744937487176,-1.,-0.939646377893399));
#24320=CARTESIAN_POINT('Ctrl Pts',(-1.59810042043673,-1.,-0.946078063315257));
#24321=CARTESIAN_POINT('Ctrl Pts',(-1.60706069896936,-1.,-0.951613284356035));
#24322=CARTESIAN_POINT('Ctrl Pts',(-1.61449324337085,-1.,-0.956354422920671));
#24323=CARTESIAN_POINT('Ctrl Pts',(-1.62061638140221,-1.,-0.960438326101729));
#24324=CARTESIAN_POINT('Ctrl Pts',(-1.62571930670187,-1.,-0.964046107040536));
#24325=CARTESIAN_POINT('Ctrl Pts',(-1.63013849959461,-1.,-0.967387853230345));
#24326=CARTESIAN_POINT('Ctrl Pts',(-1.63420665729798,-1.,-0.970669715997509));
#24327=CARTESIAN_POINT('Ctrl Pts',(-1.63820952658144,-1.,-0.974066058287418));
#24328=CARTESIAN_POINT('Ctrl Pts',(-1.64233990826687,-1.,-0.977689794119416));
#24329=CARTESIAN_POINT('Ctrl Pts',(-1.64665139190656,-1.,-0.981562530939489));
#24330=CARTESIAN_POINT('Ctrl Pts',(-1.65110016612638,-1.,-0.985642622920821));
#24331=CARTESIAN_POINT('Ctrl Pts',(-1.65559044289699,-1.,-0.989855627854165));
#24332=CARTESIAN_POINT('Ctrl Pts',(-1.66001553809947,-1.,-0.994121836661306));
#24333=CARTESIAN_POINT('Ctrl Pts',(-1.66430758030376,-1.,-0.998389654952758));
#24334=CARTESIAN_POINT('Ctrl Pts',(-1.66846059277303,-1.,-1.00265091003727));
#24335=CARTESIAN_POINT('Ctrl Pts',(-1.67250335383293,-1.,-1.00692206696414));
#24336=CARTESIAN_POINT('Ctrl Pts',(-1.67648246776464,-1.,-1.01123236493511));
#24337=CARTESIAN_POINT('Ctrl Pts',(-1.68044289894798,-1.,-1.01561026162773));
#24338=CARTESIAN_POINT('Ctrl Pts',(-1.68440578021706,-1.,-1.02006795074201));
#24339=CARTESIAN_POINT('Ctrl Pts',(-1.68836910178447,-1.,-1.02460180535255));
#24340=CARTESIAN_POINT('Ctrl Pts',(-1.69231840863458,-1.,-1.02919977579147));
#24341=CARTESIAN_POINT('Ctrl Pts',(-1.69623414782771,-1.,-1.03384646003588));
#24342=CARTESIAN_POINT('Ctrl Pts',(-1.70010052930962,-1.,-1.03852922490789));
#24343=CARTESIAN_POINT('Ctrl Pts',(-1.70391338707982,-1.,-1.04324363334554));
#24344=CARTESIAN_POINT('Ctrl Pts',(-1.70767646263649,-1.,-1.04799085404995));
#24345=CARTESIAN_POINT('Ctrl Pts',(-1.71139783543989,-1.,-1.05277517202855));
#24346=CARTESIAN_POINT('Ctrl Pts',(-1.7150865442702,-1.,-1.05760163192479));
#24347=CARTESIAN_POINT('Ctrl Pts',(-1.71874858456904,-1.,-1.06247324680647));
#24348=CARTESIAN_POINT('Ctrl Pts',(-1.72238500928453,-1.,-1.06738966975462));
#24349=CARTESIAN_POINT('Ctrl Pts',(-1.72599406198488,-1.,-1.07234866990252));
#24350=CARTESIAN_POINT('Ctrl Pts',(-1.72957248977424,-1.,-1.0773470373727));
#24351=CARTESIAN_POINT('Ctrl Pts',(-1.73311705663407,-1.,-1.08238162784749));
#24352=CARTESIAN_POINT('Ctrl Pts',(-1.73662628326091,-1.,-1.08745056285427));
#24353=CARTESIAN_POINT('Ctrl Pts',(-1.74010053962247,-1.,-1.09255329056493));
#24354=CARTESIAN_POINT('Ctrl Pts',(-1.74354119236208,-1.,-1.09768999241225));
#24355=CARTESIAN_POINT('Ctrl Pts',(-1.74695004214923,-1.,-1.10286118991143));
#24356=CARTESIAN_POINT('Ctrl Pts',(-1.7503286607592,-1.,-1.10806728183007));
#24357=CARTESIAN_POINT('Ctrl Pts',(-1.7536777209463,-1.,-1.11330807582551));
#24358=CARTESIAN_POINT('Ctrl Pts',(-1.75699720772105,-1.,-1.11858293216763));
#24359=CARTESIAN_POINT('Ctrl Pts',(-1.76028671825096,-1.,-1.12389096855086));
#24360=CARTESIAN_POINT('Ctrl Pts',(-1.7635457196617,-1.,-1.12923123555075));
#24361=CARTESIAN_POINT('Ctrl Pts',(-1.76677384551862,-1.,-1.1346029180462));
#24362=CARTESIAN_POINT('Ctrl Pts',(-1.76997111386769,-1.,-1.14000548336975));
#24363=CARTESIAN_POINT('Ctrl Pts',(-1.77313777896194,-1.,-1.1454385822692));
#24364=CARTESIAN_POINT('Ctrl Pts',(-1.7762742255701,-1.,-1.15090197841515));
#24365=CARTESIAN_POINT('Ctrl Pts',(-1.77938085564275,-1.,-1.15639547194698));
#24366=CARTESIAN_POINT('Ctrl Pts',(-1.78245795881009,-1.,-1.16191881298499));
#24367=CARTESIAN_POINT('Ctrl Pts',(-1.78550566040443,-1.,-1.16747166312303));
#24368=CARTESIAN_POINT('Ctrl Pts',(-1.78852398877616,-1.,-1.17305363177328));
#24369=CARTESIAN_POINT('Ctrl Pts',(-1.79151291552689,-1.,-1.17866429440809));
#24370=CARTESIAN_POINT('Ctrl Pts',(-1.79447240321515,-1.,-1.18430321697432));
#24371=CARTESIAN_POINT('Ctrl Pts',(-1.79740245923478,-1.,-1.18996997934445));
#24372=CARTESIAN_POINT('Ctrl Pts',(-1.80030314369879,-1.,-1.19566418930242));
#24373=CARTESIAN_POINT('Ctrl Pts',(-1.80317454838603,-1.,-1.20138548938974));
#24374=CARTESIAN_POINT('Ctrl Pts',(-1.80601678480707,-1.,-1.20713356605475));
#24375=CARTESIAN_POINT('Ctrl Pts',(-1.80882996917129,-1.,-1.21290815708314));
#24376=CARTESIAN_POINT('Ctrl Pts',(-1.81161420806656,-1.,-1.21870906103557));
#24377=CARTESIAN_POINT('Ctrl Pts',(-1.81436959210434,-1.,-1.2245361330495));
#24378=CARTESIAN_POINT('Ctrl Pts',(-1.8165508718364,-1.,-1.2292186489137));
#24379=CARTESIAN_POINT('Ctrl Pts',(-1.81817389921279,-1.,-1.2327422452705));
#24380=CARTESIAN_POINT('Ctrl Pts',(-1.81925017193666,-1.,-1.23509651170476));
#24381=CARTESIAN_POINT('Ctrl Pts',(-1.81978687191668,-1.,-1.23627494547115));
#24382=CARTESIAN_POINT('',(-1.73811241238545,-1.,-1.34869019493419));
#24383=CARTESIAN_POINT('',(-1.81978687191668,-1.,-1.23627494547115));
#24384=CARTESIAN_POINT('',(-1.31362392696032,-1.,-1.15624053661742));
#24385=CARTESIAN_POINT('Ctrl Pts',(-1.73811241238545,-1.,-1.34869019493419));
#24386=CARTESIAN_POINT('Ctrl Pts',(-1.73682580585691,-1.,-1.34854391898045));
#24387=CARTESIAN_POINT('Ctrl Pts',(-1.73425417885907,-1.,-1.34824783112887));
#24388=CARTESIAN_POINT('Ctrl Pts',(-1.7304014965394,-1.,-1.34779309152035));
#24389=CARTESIAN_POINT('Ctrl Pts',(-1.72527410680674,-1.,-1.34716554819527));
#24390=CARTESIAN_POINT('Ctrl Pts',(-1.7188807715049,-1.,-1.34634568653227));
#24391=CARTESIAN_POINT('Ctrl Pts',(-1.71250340686822,-1.,-1.34549029589416));
#24392=CARTESIAN_POINT('Ctrl Pts',(-1.70614212266738,-1.,-1.34459924533831));
#24393=CARTESIAN_POINT('Ctrl Pts',(-1.69979707754427,-1.,-1.34367237124483));
#24394=CARTESIAN_POINT('Ctrl Pts',(-1.6934684849687,-1.,-1.34270948206319));
#24395=CARTESIAN_POINT('Ctrl Pts',(-1.68715660868764,-1.,-1.341710374848));
#24396=CARTESIAN_POINT('Ctrl Pts',(-1.68086176030362,-1.,-1.34067485185203));
#24397=CARTESIAN_POINT('Ctrl Pts',(-1.67458429426086,-1.,-1.3396027347034));
#24398=CARTESIAN_POINT('Ctrl Pts',(-1.66832460783989,-1.,-1.33849388654388));
#24399=CARTESIAN_POINT('Ctrl Pts',(-1.66208312541983,-1.,-1.33734820885262));
#24400=CARTESIAN_POINT('Ctrl Pts',(-1.65586025952593,-1.,-1.33616559745172));
#24401=CARTESIAN_POINT('Ctrl Pts',(-1.6496563728683,-1.,-1.33494590467993));
#24402=CARTESIAN_POINT('Ctrl Pts',(-1.6434717485603,-1.,-1.33368890676572));
#24403=CARTESIAN_POINT('Ctrl Pts',(-1.63730653475089,-1.,-1.33239425103724));
#24404=CARTESIAN_POINT('Ctrl Pts',(-1.63116079730923,-1.,-1.33106149345645));
#24405=CARTESIAN_POINT('Ctrl Pts',(-1.62503464209797,-1.,-1.3296901950568));
#24406=CARTESIAN_POINT('Ctrl Pts',(-1.61892832270724,-1.,-1.32828000610449));
#24407=CARTESIAN_POINT('Ctrl Pts',(-1.6128423401575,-1.,-1.32683074483356));
#24408=CARTESIAN_POINT('Ctrl Pts',(-1.60677758290954,-1.,-1.32534250785782));
#24409=CARTESIAN_POINT('Ctrl Pts',(-1.60073511858687,-1.,-1.32381550858256));
#24410=CARTESIAN_POINT('Ctrl Pts',(-1.59471591079403,-1.,-1.32224985747682));
#24411=CARTESIAN_POINT('Ctrl Pts',(-1.58872057258245,-1.,-1.32064537110892));
#24412=CARTESIAN_POINT('Ctrl Pts',(-1.58274907898834,-1.,-1.31900135021432));
#24413=CARTESIAN_POINT('Ctrl Pts',(-1.5768005650559,-1.,-1.31731642317187));
#24414=CARTESIAN_POINT('Ctrl Pts',(-1.57087397835723,-1.,-1.31558903860016));
#24415=CARTESIAN_POINT('Ctrl Pts',(-1.56496872402353,-1.,-1.31381795281002));
#24416=CARTESIAN_POINT('Ctrl Pts',(-1.55908521254821,-1.,-1.31200264341696));
#24417=CARTESIAN_POINT('Ctrl Pts',(-1.55322568759481,-1.,-1.31014393684222));
#24418=CARTESIAN_POINT('Ctrl Pts',(-1.54739413957185,-1.,-1.30824393907473));
#24419=CARTESIAN_POINT('Ctrl Pts',(-1.54159462645432,-1.,-1.30630475189556));
#24420=CARTESIAN_POINT('Ctrl Pts',(-1.53582981268977,-1.,-1.30432735639489));
#24421=CARTESIAN_POINT('Ctrl Pts',(-1.53009970283891,-1.,-1.30231064395568));
#24422=CARTESIAN_POINT('Ctrl Pts',(-1.52439957861062,-1.,-1.30024984366328));
#24423=CARTESIAN_POINT('Ctrl Pts',(-1.51872184912724,-1.,-1.29813791800747));
#24424=CARTESIAN_POINT('Ctrl Pts',(-1.51305994241402,-1.,-1.29596850710509));
#24425=CARTESIAN_POINT('Ctrl Pts',(-1.50741159078365,-1.,-1.29373841372842));
#24426=CARTESIAN_POINT('Ctrl Pts',(-1.50178230149776,-1.,-1.29145022885181));
#24427=CARTESIAN_POINT('Ctrl Pts',(-1.49618896881754,-1.,-1.28911506584254));
#24428=CARTESIAN_POINT('Ctrl Pts',(-1.4906522831278,-1.,-1.2867467611644));
#24429=CARTESIAN_POINT('Ctrl Pts',(-1.4851881711891,-1.,-1.28435533880201));
#24430=CARTESIAN_POINT('Ctrl Pts',(-1.47980070347095,-1.,-1.28194158939517));
#24431=CARTESIAN_POINT('Ctrl Pts',(-1.4744717526707,-1.,-1.2794891824849));
#24432=CARTESIAN_POINT('Ctrl Pts',(-1.46916035917133,-1.,-1.27696414831089));
#24433=CARTESIAN_POINT('Ctrl Pts',(-1.46382431332476,-1.,-1.27433119897822));
#24434=CARTESIAN_POINT('Ctrl Pts',(-1.45843906294697,-1.,-1.27156805265289));
#24435=CARTESIAN_POINT('Ctrl Pts',(-1.45301422764247,-1.,-1.2686778680489));
#24436=CARTESIAN_POINT('Ctrl Pts',(-1.44761985001662,-1.,-1.26570925118868));
#24437=CARTESIAN_POINT('Ctrl Pts',(-1.44236470511303,-1.,-1.26273903323859));
#24438=CARTESIAN_POINT('Ctrl Pts',(-1.43734919180848,-1.,-1.25983531012005));
#24439=CARTESIAN_POINT('Ctrl Pts',(-1.43262645609691,-1.,-1.25702687965755));
#24440=CARTESIAN_POINT('Ctrl Pts',(-1.42815938799387,-1.,-1.25426945222639));
#24441=CARTESIAN_POINT('Ctrl Pts',(-1.42378102115575,-1.,-1.2514145557001));
#24442=CARTESIAN_POINT('Ctrl Pts',(-1.41923722596025,-1.,-1.24824430986571));
#24443=CARTESIAN_POINT('Ctrl Pts',(-1.41422913175179,-1.,-1.24450600513056));
#24444=CARTESIAN_POINT('Ctrl Pts',(-1.40845295531283,-1.,-1.23994455029534));
#24445=CARTESIAN_POINT('Ctrl Pts',(-1.40164708206106,-1.,-1.23434087290423));
#24446=CARTESIAN_POINT('Ctrl Pts',(-1.39361389568796,-1.,-1.22752961899387));
#24447=CARTESIAN_POINT('Ctrl Pts',(-1.38420564527715,-1.,-1.21938737280852));
#24448=CARTESIAN_POINT('Ctrl Pts',(-1.37331915607905,-1.,-1.20982812925645));
#24449=CARTESIAN_POINT('Ctrl Pts',(-1.36088705043885,-1.,-1.1987959077932));
#24450=CARTESIAN_POINT('Ctrl Pts',(-1.34687054001093,-1.,-1.18625865667441));
#24451=CARTESIAN_POINT('Ctrl Pts',(-1.33437539347008,-1.,-1.17501305789857));
#24452=CARTESIAN_POINT('Ctrl Pts',(-1.32428080721772,-1.,-1.16589330093588));
#24453=CARTESIAN_POINT('Ctrl Pts',(-1.31722977216397,-1.,-1.15950888730809));
#24454=CARTESIAN_POINT('Ctrl Pts',(-1.31362392696032,-1.,-1.15624053661742));
#24455=CARTESIAN_POINT('',(-1.15624053661742,-1.,-1.31362392696033));
#24456=CARTESIAN_POINT('Origin',(0.,-1.,0.));
#24457=CARTESIAN_POINT('',(-1.34869019493419,-1.,-1.73811241238545));
#24458=CARTESIAN_POINT('Ctrl Pts',(-1.15624053661742,-1.,-1.31362392696033));
#24459=CARTESIAN_POINT('Ctrl Pts',(-1.15950888730433,-1.,-1.3172297721596));
#24460=CARTESIAN_POINT('Ctrl Pts',(-1.16589330092532,-1.,-1.32428080720544));
#24461=CARTESIAN_POINT('Ctrl Pts',(-1.17501305787994,-1.,-1.33437539344842));
#24462=CARTESIAN_POINT('Ctrl Pts',(-1.18625865664915,-1.,-1.34687053998157));
#24463=CARTESIAN_POINT('Ctrl Pts',(-1.1987959077656,-1.,-1.36088705040677));
#24464=CARTESIAN_POINT('Ctrl Pts',(-1.20982812923113,-1.,-1.37331915604962));
#24465=CARTESIAN_POINT('Ctrl Pts',(-1.21938737278853,-1.,-1.38420564525391));
#24466=CARTESIAN_POINT('Ctrl Pts',(-1.22752961898063,-1.,-1.39361389567257));
#24467=CARTESIAN_POINT('Ctrl Pts',(-1.23434087289768,-1.,-1.40164708205345));
#24468=CARTESIAN_POINT('Ctrl Pts',(-1.23994455029421,-1.,-1.40845295531151));
#24469=CARTESIAN_POINT('Ctrl Pts',(-1.24450600513278,-1.,-1.41422913175437));
#24470=CARTESIAN_POINT('Ctrl Pts',(-1.24824430986911,-1.,-1.41923722596421));
#24471=CARTESIAN_POINT('Ctrl Pts',(-1.25141455570299,-1.,-1.42378102115911));
#24472=CARTESIAN_POINT('Ctrl Pts',(-1.25426945222783,-1.,-1.42815938799555));
#24473=CARTESIAN_POINT('Ctrl Pts',(-1.25702687965744,-1.,-1.43262645609679));
#24474=CARTESIAN_POINT('Ctrl Pts',(-1.25983531011894,-1.,-1.43734919180719));
#24475=CARTESIAN_POINT('Ctrl Pts',(-1.26273903323723,-1.,-1.44236470511145));
#24476=CARTESIAN_POINT('Ctrl Pts',(-1.26570925118767,-1.,-1.44761985001544));
#24477=CARTESIAN_POINT('Ctrl Pts',(-1.26867786804854,-1.,-1.45301422764205));
#24478=CARTESIAN_POINT('Ctrl Pts',(-1.27156805265312,-1.,-1.45843906294725));
#24479=CARTESIAN_POINT('Ctrl Pts',(-1.27433119897877,-1.,-1.4638243133254));
#24480=CARTESIAN_POINT('Ctrl Pts',(-1.27696414831144,-1.,-1.46916035917197));
#24481=CARTESIAN_POINT('Ctrl Pts',(-1.27948918248524,-1.,-1.4744717526711));
#24482=CARTESIAN_POINT('Ctrl Pts',(-1.28194158939522,-1.,-1.47980070347102));
#24483=CARTESIAN_POINT('Ctrl Pts',(-1.28435533880184,-1.,-1.48518817118891));
#24484=CARTESIAN_POINT('Ctrl Pts',(-1.28674676116415,-1.,-1.4906522831275));
#24485=CARTESIAN_POINT('Ctrl Pts',(-1.28911506584232,-1.,-1.49618896881729));
#24486=CARTESIAN_POINT('Ctrl Pts',(-1.29145022885171,-1.,-1.50178230149764));
#24487=CARTESIAN_POINT('Ctrl Pts',(-1.29373841372843,-1.,-1.50741159078367));
#24488=CARTESIAN_POINT('Ctrl Pts',(-1.29596850710518,-1.,-1.51305994241412));
#24489=CARTESIAN_POINT('Ctrl Pts',(-1.29813791800757,-1.,-1.51872184912735));
#24490=CARTESIAN_POINT('Ctrl Pts',(-1.30024984366334,-1.,-1.5243995786107));
#24491=CARTESIAN_POINT('Ctrl Pts',(-1.3023106439557,-1.,-1.53009970283893));
#24492=CARTESIAN_POINT('Ctrl Pts',(-1.30432735639487,-1.,-1.53582981268976));
#24493=CARTESIAN_POINT('Ctrl Pts',(-1.30630475189553,-1.,-1.54159462645428));
#24494=CARTESIAN_POINT('Ctrl Pts',(-1.30824393907471,-1.,-1.54739413957183));
#24495=CARTESIAN_POINT('Ctrl Pts',(-1.31014393684221,-1.,-1.55322568759481));
#24496=CARTESIAN_POINT('Ctrl Pts',(-1.31200264341696,-1.,-1.55908521254822));
#24497=CARTESIAN_POINT('Ctrl Pts',(-1.31381795281002,-1.,-1.56496872402352));
#24498=CARTESIAN_POINT('Ctrl Pts',(-1.31558903860015,-1.,-1.57087397835721));
#24499=CARTESIAN_POINT('Ctrl Pts',(-1.31731642317183,-1.,-1.57680056505585));
#24500=CARTESIAN_POINT('Ctrl Pts',(-1.31900135021428,-1.,-1.58274907898829));
#24501=CARTESIAN_POINT('Ctrl Pts',(-1.32064537110891,-1.,-1.58872057258244));
#24502=CARTESIAN_POINT('Ctrl Pts',(-1.32224985747686,-1.,-1.59471591079408));
#24503=CARTESIAN_POINT('Ctrl Pts',(-1.32381550858266,-1.,-1.600735118587));
#24504=CARTESIAN_POINT('Ctrl Pts',(-1.32534250785794,-1.,-1.6067775829097));
#24505=CARTESIAN_POINT('Ctrl Pts',(-1.32683074483365,-1.,-1.61284234015762));
#24506=CARTESIAN_POINT('Ctrl Pts',(-1.32828000610448,-1.,-1.61892832270723));
#24507=CARTESIAN_POINT('Ctrl Pts',(-1.32969019505665,-1.,-1.62503464209777));
#24508=CARTESIAN_POINT('Ctrl Pts',(-1.33106149345618,-1.,-1.63116079730887));
#24509=CARTESIAN_POINT('Ctrl Pts',(-1.33239425103694,-1.,-1.6373065347505));
#24510=CARTESIAN_POINT('Ctrl Pts',(-1.33368890676554,-1.,-1.64347174856007));
#24511=CARTESIAN_POINT('Ctrl Pts',(-1.33494590468003,-1.,-1.64965637286843));
#24512=CARTESIAN_POINT('Ctrl Pts',(-1.33616559745217,-1.,-1.65586025952651));
#24513=CARTESIAN_POINT('Ctrl Pts',(-1.33734820885331,-1.,-1.66208312542073));
#24514=CARTESIAN_POINT('Ctrl Pts',(-1.33849388654458,-1.,-1.66832460784078));
#24515=CARTESIAN_POINT('Ctrl Pts',(-1.33960273470372,-1.,-1.67458429426126));
#24516=CARTESIAN_POINT('Ctrl Pts',(-1.3406748518516,-1.,-1.68086176030308));
#24517=CARTESIAN_POINT('Ctrl Pts',(-1.34171037484673,-1.,-1.68715660868602));
#24518=CARTESIAN_POINT('Ctrl Pts',(-1.34270948206139,-1.,-1.6934684849664));
#24519=CARTESIAN_POINT('Ctrl Pts',(-1.34367237124322,-1.,-1.69979707754221));
#24520=CARTESIAN_POINT('Ctrl Pts',(-1.34459924533783,-1.,-1.70614212266676));
#24521=CARTESIAN_POINT('Ctrl Pts',(-1.34549029589563,-1.,-1.71250340687011));
#24522=CARTESIAN_POINT('Ctrl Pts',(-1.34634568653586,-1.,-1.7188807715095));
#24523=CARTESIAN_POINT('Ctrl Pts',(-1.34716554820013,-1.,-1.72527410681298));
#24524=CARTESIAN_POINT('Ctrl Pts',(-1.3477930915247,-1.,-1.73040149654497));
#24525=CARTESIAN_POINT('Ctrl Pts',(-1.34824783113158,-1.,-1.73425417886255));
#24526=CARTESIAN_POINT('Ctrl Pts',(-1.34854391898145,-1.,-1.73682580585819));
#24527=CARTESIAN_POINT('Ctrl Pts',(-1.34869019493419,-1.,-1.73811241238545));
#24528=CARTESIAN_POINT('',(-1.23627494547115,-1.,-1.81978687191668));
#24529=CARTESIAN_POINT('',(-1.34869019493419,-1.,-1.73811241238545));
#24530=CARTESIAN_POINT('',(-0.892032620296855,-1.,-1.5055822144029));
#24531=CARTESIAN_POINT('Ctrl Pts',(-1.23627494547115,-1.,-1.81978687191668));
#24532=CARTESIAN_POINT('Ctrl Pts',(-1.23509651170384,-1.,-1.81925017193531));
#24533=CARTESIAN_POINT('Ctrl Pts',(-1.23274224526804,-1.,-1.81817389920914));
#24534=CARTESIAN_POINT('Ctrl Pts',(-1.22921864890975,-1.,-1.81655087183054));
#24535=CARTESIAN_POINT('Ctrl Pts',(-1.22453613304507,-1.,-1.81436959209778));
#24536=CARTESIAN_POINT('Ctrl Pts',(-1.2187090610323,-1.,-1.81161420806172));
#24537=CARTESIAN_POINT('Ctrl Pts',(-1.2129081570818,-1.,-1.80882996916931));
#24538=CARTESIAN_POINT('Ctrl Pts',(-1.20713356605519,-1.,-1.80601678480772));
#24539=CARTESIAN_POINT('Ctrl Pts',(-1.2013854893912,-1.,-1.8031745483882));
#24540=CARTESIAN_POINT('Ctrl Pts',(-1.19566418930405,-1.,-1.80030314370121));
#24541=CARTESIAN_POINT('Ctrl Pts',(-1.1899699793456,-1.,-1.79740245923649));
#24542=CARTESIAN_POINT('Ctrl Pts',(-1.18430321697471,-1.,-1.79447240321572));
#24543=CARTESIAN_POINT('Ctrl Pts',(-1.17866429440781,-1.,-1.79151291552646));
#24544=CARTESIAN_POINT('Ctrl Pts',(-1.17305363177265,-1.,-1.78852398877523));
#24545=CARTESIAN_POINT('Ctrl Pts',(-1.16747166312239,-1.,-1.78550566040349));
#24546=CARTESIAN_POINT('Ctrl Pts',(-1.16191881298458,-1.,-1.78245795880949));
#24547=CARTESIAN_POINT('Ctrl Pts',(-1.15639547194689,-1.,-1.77938085564261));
#24548=CARTESIAN_POINT('Ctrl Pts',(-1.15090197841531,-1.,-1.77627422557034));
#24549=CARTESIAN_POINT('Ctrl Pts',(-1.14543858226948,-1.,-1.77313777896234));
#24550=CARTESIAN_POINT('Ctrl Pts',(-1.14000548337,-1.,-1.76997111386806));
#24551=CARTESIAN_POINT('Ctrl Pts',(-1.13460291804635,-1.,-1.76677384551883));
#24552=CARTESIAN_POINT('Ctrl Pts',(-1.12923123555076,-1.,-1.76354571966171));
#24553=CARTESIAN_POINT('Ctrl Pts',(-1.12389096855078,-1.,-1.76028671825084));
#24554=CARTESIAN_POINT('Ctrl Pts',(-1.11858293216752,-1.,-1.75699720772089));
#24555=CARTESIAN_POINT('Ctrl Pts',(-1.11330807582542,-1.,-1.75367772094617));
#24556=CARTESIAN_POINT('Ctrl Pts',(-1.10806728183003,-1.,-1.75032866075914));
#24557=CARTESIAN_POINT('Ctrl Pts',(-1.10286118991144,-1.,-1.74695004214924));
#24558=CARTESIAN_POINT('Ctrl Pts',(-1.09768999241229,-1.,-1.74354119236212));
#24559=CARTESIAN_POINT('Ctrl Pts',(-1.09255329056496,-1.,-1.74010053962252));
#24560=CARTESIAN_POINT('Ctrl Pts',(-1.08745056285429,-1.,-1.73662628326093));
#24561=CARTESIAN_POINT('Ctrl Pts',(-1.08238162784749,-1.,-1.73311705663407));
#24562=CARTESIAN_POINT('Ctrl Pts',(-1.0773470373727,-1.,-1.72957248977424));
#24563=CARTESIAN_POINT('Ctrl Pts',(-1.07234866990252,-1.,-1.72599406198489));
#24564=CARTESIAN_POINT('Ctrl Pts',(-1.06738966975463,-1.,-1.72238500928456));
#24565=CARTESIAN_POINT('Ctrl Pts',(-1.0624732468065,-1.,-1.71874858456908));
#24566=CARTESIAN_POINT('Ctrl Pts',(-1.05760163192481,-1.,-1.71508654427022));
#24567=CARTESIAN_POINT('Ctrl Pts',(-1.05277517202854,-1.,-1.71139783543986));
#24568=CARTESIAN_POINT('Ctrl Pts',(-1.0479908540499,-1.,-1.70767646263641));
#24569=CARTESIAN_POINT('Ctrl Pts',(-1.04324363334546,-1.,-1.70391338707969));
#24570=CARTESIAN_POINT('Ctrl Pts',(-1.03852922490782,-1.,-1.70010052930951));
#24571=CARTESIAN_POINT('Ctrl Pts',(-1.03384646003587,-1.,-1.69623414782769));
#24572=CARTESIAN_POINT('Ctrl Pts',(-1.02919977579155,-1.,-1.69231840863471));
#24573=CARTESIAN_POINT('Ctrl Pts',(-1.02460180535272,-1.,-1.68836910178475));
#24574=CARTESIAN_POINT('Ctrl Pts',(-1.02006795074222,-1.,-1.68440578021739));
#24575=CARTESIAN_POINT('Ctrl Pts',(-1.01561026162787,-1.,-1.6804428989482));
#24576=CARTESIAN_POINT('Ctrl Pts',(-1.01123236493507,-1.,-1.67648246776457));
#24577=CARTESIAN_POINT('Ctrl Pts',(-1.00692206696387,-1.,-1.67250335383248));
#24578=CARTESIAN_POINT('Ctrl Pts',(-1.00265091003682,-1.,-1.66846059277231));
#24579=CARTESIAN_POINT('Ctrl Pts',(-0.998389654952317,-1.,-1.66430758030304));
#24580=CARTESIAN_POINT('Ctrl Pts',(-0.994121836661116,-1.,-1.66001553809916));
#24581=CARTESIAN_POINT('Ctrl Pts',(-0.98985562785445,-1.,-1.65559044289746));
#24582=CARTESIAN_POINT('Ctrl Pts',(-0.985642622921626,-1.,-1.6511001661277));
#24583=CARTESIAN_POINT('Ctrl Pts',(-0.981562530940574,-1.,-1.64665139190834));
#24584=CARTESIAN_POINT('Ctrl Pts',(-0.977689794120297,-1.,-1.64233990826831));
#24585=CARTESIAN_POINT('Ctrl Pts',(-0.974066058287501,-1.,-1.63820952658157));
#24586=CARTESIAN_POINT('Ctrl Pts',(-0.970669715996356,-1.,-1.63420665729609));
#24587=CARTESIAN_POINT('Ctrl Pts',(-0.967387853228041,-1.,-1.63013849959083));
#24588=CARTESIAN_POINT('Ctrl Pts',(-0.964046107037821,-1.,-1.6257193066974));
#24589=CARTESIAN_POINT('Ctrl Pts',(-0.960438326099958,-1.,-1.62061638139929));
#24590=CARTESIAN_POINT('Ctrl Pts',(-0.956354422921573,-1.,-1.61449324337233));
#24591=CARTESIAN_POINT('Ctrl Pts',(-0.951613284361248,-1.,-1.60706069897794));
#24592=CARTESIAN_POINT('Ctrl Pts',(-0.946078063325796,-1.,-1.59810042045408));
#24593=CARTESIAN_POINT('Ctrl Pts',(-0.939646377909319,-1.,-1.58744937489796));
#24594=CARTESIAN_POINT('Ctrl Pts',(-0.932246680128849,-1.,-1.57499388385561));
#24595=CARTESIAN_POINT('Ctrl Pts',(-0.923832188966322,-1.,-1.56065988582509));
#24596=CARTESIAN_POINT('Ctrl Pts',(-0.91437591904658,-1.,-1.54440491152808));
#24597=CARTESIAN_POINT('Ctrl Pts',(-0.905967409640499,-1.,-1.52984849890434));
#24598=CARTESIAN_POINT('Ctrl Pts',(-0.89918504749193,-1.,-1.51805569591479));
#24599=CARTESIAN_POINT('Ctrl Pts',(-0.894452006967538,-1.,-1.50980486807181));
#24600=CARTESIAN_POINT('Ctrl Pts',(-0.892032620296855,-1.,-1.5055822144029));
#24601=CARTESIAN_POINT('',(-0.693717979106305,-1.,-1.60662857109684));
#24602=CARTESIAN_POINT('Origin',(0.,-1.,0.));
#24603=CARTESIAN_POINT('',(-0.745574324794401,-1.,-2.0698113262342));
#24604=CARTESIAN_POINT('Ctrl Pts',(-0.693717979106305,-1.,-1.60662857109684));
#24605=CARTESIAN_POINT('Ctrl Pts',(-0.69571209787897,-1.,-1.61106790957619));
#24606=CARTESIAN_POINT('Ctrl Pts',(-0.699605146398837,-1.,-1.61974673471117));
#24607=CARTESIAN_POINT('Ctrl Pts',(-0.705159151977294,-1.,-1.6321654166204));
#24608=CARTESIAN_POINT('Ctrl Pts',(-0.711993139340447,-1.,-1.64752408828442));
#24609=CARTESIAN_POINT('Ctrl Pts',(-0.71958543378795,-1.,-1.66472880551777));
#24610=CARTESIAN_POINT('Ctrl Pts',(-0.726235967982445,-1.,-1.67996158451922));
#24611=CARTESIAN_POINT('Ctrl Pts',(-0.731963238685357,-1.,-1.69326921972915));
#24612=CARTESIAN_POINT('Ctrl Pts',(-0.736799665716932,-1.,-1.70473309004249));
#24613=CARTESIAN_POINT('Ctrl Pts',(-0.74079516202821,-1.,-1.71447789751001));
#24614=CARTESIAN_POINT('Ctrl Pts',(-0.744021445433093,-1.,-1.72268229916769));
#24615=CARTESIAN_POINT('Ctrl Pts',(-0.746574710097752,-1.,-1.72958533647714));
#24616=CARTESIAN_POINT('Ctrl Pts',(-0.74858246295687,-1.,-1.7355035168033));
#24617=CARTESIAN_POINT('Ctrl Pts',(-0.750193435981249,-1.,-1.74080458267114));
#24618=CARTESIAN_POINT('Ctrl Pts',(-0.751555614164482,-1.,-1.74585086852502));
#24619=CARTESIAN_POINT('Ctrl Pts',(-0.752797683531314,-1.,-1.75095139468794));
#24620=CARTESIAN_POINT('Ctrl Pts',(-0.754009254027829,-1.,-1.75631083600019));
#24621=CARTESIAN_POINT('Ctrl Pts',(-0.755220979974461,-1.,-1.76197817240128));
#24622=CARTESIAN_POINT('Ctrl Pts',(-0.75642189602781,-1.,-1.76789396002998));
#24623=CARTESIAN_POINT('Ctrl Pts',(-0.757578264077029,-1.,-1.77394167108292));
#24624=CARTESIAN_POINT('Ctrl Pts',(-0.758650626677518,-1.,-1.77999411220945));
#24625=CARTESIAN_POINT('Ctrl Pts',(-0.759614401110189,-1.,-1.78596964884604));
#24626=CARTESIAN_POINT('Ctrl Pts',(-0.760469555880749,-1.,-1.7918581561088));
#24627=CARTESIAN_POINT('Ctrl Pts',(-0.761229695230558,-1.,-1.79768986997783));
#24628=CARTESIAN_POINT('Ctrl Pts',(-0.761915336443547,-1.,-1.80351583877342));
#24629=CARTESIAN_POINT('Ctrl Pts',(-0.762546129463938,-1.,-1.80938551463965));
#24630=CARTESIAN_POINT('Ctrl Pts',(-0.763132003836634,-1.,-1.8153211840553));
#24631=CARTESIAN_POINT('Ctrl Pts',(-0.763673465462726,-1.,-1.82131873145266));
#24632=CARTESIAN_POINT('Ctrl Pts',(-0.764165902605995,-1.,-1.82735991200065));
#24633=CARTESIAN_POINT('Ctrl Pts',(-0.764602549687853,-1.,-1.83342077227142));
#24634=CARTESIAN_POINT('Ctrl Pts',(-0.764978057881737,-1.,-1.83948181064835));
#24635=CARTESIAN_POINT('Ctrl Pts',(-0.765291664862029,-1.,-1.84553698875924));
#24636=CARTESIAN_POINT('Ctrl Pts',(-0.765545710619062,-1.,-1.85158945130063));
#24637=CARTESIAN_POINT('Ctrl Pts',(-0.765744212909318,-1.,-1.85764741390394));
#24638=CARTESIAN_POINT('Ctrl Pts',(-0.765891519092547,-1.,-1.86372027063312));
#24639=CARTESIAN_POINT('Ctrl Pts',(-0.765990708546091,-1.,-1.86981398314341));
#24640=CARTESIAN_POINT('Ctrl Pts',(-0.766042837036744,-1.,-1.87592888967883));
#24641=CARTESIAN_POINT('Ctrl Pts',(-0.766047794851865,-1.,-1.88206215302561));
#24642=CARTESIAN_POINT('Ctrl Pts',(-0.766004837062091,-1.,-1.88820926433409));
#24643=CARTESIAN_POINT('Ctrl Pts',(-0.765913193856978,-1.,-1.89436577771388));
#24644=CARTESIAN_POINT('Ctrl Pts',(-0.765772772593386,-1.,-1.90052930393596));
#24645=CARTESIAN_POINT('Ctrl Pts',(-0.765584196937919,-1.,-1.90669961402356));
#24646=CARTESIAN_POINT('Ctrl Pts',(-0.765348465884722,-1.,-1.91287765805169));
#24647=CARTESIAN_POINT('Ctrl Pts',(-0.765066729667088,-1.,-1.91906491634196));
#24648=CARTESIAN_POINT('Ctrl Pts',(-0.764740025488211,-1.,-1.92526263537048));
#24649=CARTESIAN_POINT('Ctrl Pts',(-0.764369010673941,-1.,-1.93147105496382));
#24650=CARTESIAN_POINT('Ctrl Pts',(-0.763954049121458,-1.,-1.93768964875886));
#24651=CARTESIAN_POINT('Ctrl Pts',(-0.763495333538629,-1.,-1.9439174661764));
#24652=CARTESIAN_POINT('Ctrl Pts',(-0.762992990878769,-1.,-1.95015342590024));
#24653=CARTESIAN_POINT('Ctrl Pts',(-0.762447203806179,-1.,-1.95639665309869));
#24654=CARTESIAN_POINT('Ctrl Pts',(-0.761858300014423,-1.,-1.96264672744186));
#24655=CARTESIAN_POINT('Ctrl Pts',(-0.76122669048382,-1.,-1.96890351582499));
#24656=CARTESIAN_POINT('Ctrl Pts',(-0.760552825409757,-1.,-1.97516705321494));
#24657=CARTESIAN_POINT('Ctrl Pts',(-0.75983714745219,-1.,-1.98143741418172));
#24658=CARTESIAN_POINT('Ctrl Pts',(-0.759080037802488,-1.,-1.98771456680874));
#24659=CARTESIAN_POINT('Ctrl Pts',(-0.758281796766761,-1.,-1.99399831098817));
#24660=CARTESIAN_POINT('Ctrl Pts',(-0.757442676862724,-1.,-2.00028834739178));
#24661=CARTESIAN_POINT('Ctrl Pts',(-0.75656290464667,-1.,-2.0065843158773));
#24662=CARTESIAN_POINT('Ctrl Pts',(-0.755642704957865,-1.,-2.01288584328084));
#24663=CARTESIAN_POINT('Ctrl Pts',(-0.754682330722816,-1.,-2.01919259405809));
#24664=CARTESIAN_POINT('Ctrl Pts',(-0.753682061112768,-1.,-2.02550428623313));
#24665=CARTESIAN_POINT('Ctrl Pts',(-0.752642180487211,-1.,-2.03182068456221));
#24666=CARTESIAN_POINT('Ctrl Pts',(-0.751562963361115,-1.,-2.03814160092099));
#24667=CARTESIAN_POINT('Ctrl Pts',(-0.750444657875576,-1.,-2.04446689147979));
#24668=CARTESIAN_POINT('Ctrl Pts',(-0.749287468665046,-1.,-2.05079645592154));
#24669=CARTESIAN_POINT('Ctrl Pts',(-0.748091554183802,-1.,-2.05713023031006));
#24670=CARTESIAN_POINT('Ctrl Pts',(-0.747103932787919,-1.,-2.06220058927826));
#24671=CARTESIAN_POINT('Ctrl Pts',(-0.7463458715442,-1.,-2.06600523016815));
#24672=CARTESIAN_POINT('Ctrl Pts',(-0.745832791378367,-1.,-2.06854248895728));
#24673=CARTESIAN_POINT('Ctrl Pts',(-0.745574324794401,-1.,-2.0698113262342));
#24674=CARTESIAN_POINT('',(-0.61342227326009,-1.,-2.11275013067528));
#24675=CARTESIAN_POINT('',(-0.745574324794401,-1.,-2.0698113262342));
#24676=CARTESIAN_POINT('',(-0.383122945602004,-1.,-1.7075470150345));
#24677=CARTESIAN_POINT('Ctrl Pts',(-0.61342227326009,-1.,-2.11275013067528));
#24678=CARTESIAN_POINT('Ctrl Pts',(-0.6124673655618,-1.,-2.11187554259986));
#24679=CARTESIAN_POINT('Ctrl Pts',(-0.610560911689899,-1.,-2.11012443807238));
#24680=CARTESIAN_POINT('Ctrl Pts',(-0.607711315454876,-1.,-2.1074919961518));
#24681=CARTESIAN_POINT('Ctrl Pts',(-0.60393203073603,-1.,-2.10397049886949));
#24682=CARTESIAN_POINT('Ctrl Pts',(-0.599241616420533,-1.,-2.0995493086477));
#24683=CARTESIAN_POINT('Ctrl Pts',(-0.594585006052162,-1.,-2.0951087622027));
#24684=CARTESIAN_POINT('Ctrl Pts',(-0.589962365403406,-1.,-2.09064881812129));
#24685=CARTESIAN_POINT('Ctrl Pts',(-0.585373918991617,-1.,-2.08616943727951));
#24686=CARTESIAN_POINT('Ctrl Pts',(-0.580819952108063,-1.,-2.08167059018418));
#24687=CARTESIAN_POINT('Ctrl Pts',(-0.576300797416844,-1.,-2.07715226767559));
#24688=CARTESIAN_POINT('Ctrl Pts',(-0.571816823242603,-1.,-2.07261449292824));
#24689=CARTESIAN_POINT('Ctrl Pts',(-0.567368421181087,-1.,-2.06805732997334));
#24690=CARTESIAN_POINT('Ctrl Pts',(-0.562955993082261,-1.,-2.06348090160589));
#24691=CARTESIAN_POINT('Ctrl Pts',(-0.558579940185151,-1.,-2.05888537756462));
#24692=CARTESIAN_POINT('Ctrl Pts',(-0.554240657463906,-1.,-2.05427091604413));
#24693=CARTESIAN_POINT('Ctrl Pts',(-0.549938525150295,-1.,-2.04963761077958));
#24694=CARTESIAN_POINT('Ctrl Pts',(-0.54567390381743,-1.,-2.04498544714588));
#24695=CARTESIAN_POINT('Ctrl Pts',(-0.541447120615659,-1.,-2.04031422690527));
#24696=CARTESIAN_POINT('Ctrl Pts',(-0.537258489833262,-1.,-2.03562362954037));
#24697=CARTESIAN_POINT('Ctrl Pts',(-0.533108355132977,-1.,-2.03091336214426));
#24698=CARTESIAN_POINT('Ctrl Pts',(-0.528997127241914,-1.,-2.0261832908329));
#24699=CARTESIAN_POINT('Ctrl Pts',(-0.524925318333476,-1.,-2.02143356304698));
#24700=CARTESIAN_POINT('Ctrl Pts',(-0.52089359039937,-1.,-2.01666477917286));
#24701=CARTESIAN_POINT('Ctrl Pts',(-0.516902681728687,-1.,-2.01187773939242));
#24702=CARTESIAN_POINT('Ctrl Pts',(-0.512953306961792,-1.,-2.00707309946949));
#24703=CARTESIAN_POINT('Ctrl Pts',(-0.509046069886157,-1.,-2.00225107134734));
#24704=CARTESIAN_POINT('Ctrl Pts',(-0.505181361323026,-1.,-1.99741107463572));
#24705=CARTESIAN_POINT('Ctrl Pts',(-0.501359287727146,-1.,-1.99255149126155));
#24706=CARTESIAN_POINT('Ctrl Pts',(-0.497579909545574,-1.,-1.98767044752932));
#24707=CARTESIAN_POINT('Ctrl Pts',(-0.493843476541495,-1.,-1.98276658761821));
#24708=CARTESIAN_POINT('Ctrl Pts',(-0.490150627860952,-1.,-1.97783973019229));
#24709=CARTESIAN_POINT('Ctrl Pts',(-0.486502692907659,-1.,-1.97289186263272));
#24710=CARTESIAN_POINT('Ctrl Pts',(-0.482901662120691,-1.,-1.96792703422362));
#24711=CARTESIAN_POINT('Ctrl Pts',(-0.479349583074855,-1.,-1.96294933055943));
#24712=CARTESIAN_POINT('Ctrl Pts',(-0.475848034683176,-1.,-1.95796111148177));
#24713=CARTESIAN_POINT('Ctrl Pts',(-0.472397672264072,-1.,-1.95296148278133));
#24714=CARTESIAN_POINT('Ctrl Pts',(-0.468997482913135,-1.,-1.94794381136514));
#24715=CARTESIAN_POINT('Ctrl Pts',(-0.46564546202603,-1.,-1.9428979419619));
#24716=CARTESIAN_POINT('Ctrl Pts',(-0.462340031009056,-1.,-1.93781486640821));
#24717=CARTESIAN_POINT('Ctrl Pts',(-0.459081234547926,-1.,-1.93269066517934));
#24718=CARTESIAN_POINT('Ctrl Pts',(-0.455872005174371,-1.,-1.92753067150476));
#24719=CARTESIAN_POINT('Ctrl Pts',(-0.452719478359432,-1.,-1.92235380648502));
#24720=CARTESIAN_POINT('Ctrl Pts',(-0.449632260106662,-1.,-1.91718342555755));
#24721=CARTESIAN_POINT('Ctrl Pts',(-0.446617343485711,-1.,-1.9120369998112));
#24722=CARTESIAN_POINT('Ctrl Pts',(-0.443677556849151,-1.,-1.90691756144898));
#24723=CARTESIAN_POINT('Ctrl Pts',(-0.440807833704038,-1.,-1.90180124389086));
#24724=CARTESIAN_POINT('Ctrl Pts',(-0.437995003948244,-1.,-1.89663648956466));
#24725=CARTESIAN_POINT('Ctrl Pts',(-0.435225660963383,-1.,-1.89136993975504));
#24726=CARTESIAN_POINT('Ctrl Pts',(-0.432493038548748,-1.,-1.88596913666793));
#24727=CARTESIAN_POINT('Ctrl Pts',(-0.429803062482344,-1.,-1.88044229001832));
#24728=CARTESIAN_POINT('Ctrl Pts',(-0.427183828519102,-1.,-1.87486989291484));
#24729=CARTESIAN_POINT('Ctrl Pts',(-0.424678177291359,-1.,-1.86937803944323));
#24730=CARTESIAN_POINT('Ctrl Pts',(-0.422327307418275,-1.,-1.86408083334028));
#24731=CARTESIAN_POINT('Ctrl Pts',(-0.420157287975619,-1.,-1.85903281096686));
#24732=CARTESIAN_POINT('Ctrl Pts',(-0.418164129143534,-1.,-1.85417632856234));
#24733=CARTESIAN_POINT('Ctrl Pts',(-0.416300022038864,-1.,-1.84929312929882));
#24734=CARTESIAN_POINT('Ctrl Pts',(-0.41448743825434,-1.,-1.8440575707371));
#24735=CARTESIAN_POINT('Ctrl Pts',(-0.412633125322162,-1.,-1.83808953475839));
#24736=CARTESIAN_POINT('Ctrl Pts',(-0.410641256301675,-1.,-1.83100408895216));
#24737=CARTESIAN_POINT('Ctrl Pts',(-0.408428948108533,-1.,-1.8224702267854));
#24738=CARTESIAN_POINT('Ctrl Pts',(-0.405933518411838,-1.,-1.81223801813988));
#24739=CARTESIAN_POINT('Ctrl Pts',(-0.403107976170441,-1.,-1.80012077176221));
#24740=CARTESIAN_POINT('Ctrl Pts',(-0.39991940378308,-1.,-1.78598826347533));
#24741=CARTESIAN_POINT('Ctrl Pts',(-0.39634619612042,-1.,-1.7697556004756));
#24742=CARTESIAN_POINT('Ctrl Pts',(-0.392375812294307,-1.,-1.75137405313962));
#24743=CARTESIAN_POINT('Ctrl Pts',(-0.388877023509191,-1.,-1.7349317097561));
#24744=CARTESIAN_POINT('Ctrl Pts',(-0.38607079032701,-1.,-1.72162022246158));
#24745=CARTESIAN_POINT('Ctrl Pts',(-0.384119047315542,-1.,-1.71231062891958));
#24746=CARTESIAN_POINT('Ctrl Pts',(-0.383122945602004,-1.,-1.7075470150345));
#24747=CARTESIAN_POINT('',(-0.163289472382896,-1.,-1.74236521665491));
#24748=CARTESIAN_POINT('Origin',(0.,-1.,0.));
#24749=CARTESIAN_POINT('',(-0.0694764450219581,-1.,-2.19890268624765));
#24750=CARTESIAN_POINT('Ctrl Pts',(-0.163289472382896,-1.,-1.74236521665491));
#24751=CARTESIAN_POINT('Ctrl Pts',(-0.163814161002002,-1.,-1.7472034950333));
#24752=CARTESIAN_POINT('Ctrl Pts',(-0.164834765707158,-1.,-1.75666056638427));
#24753=CARTESIAN_POINT('Ctrl Pts',(-0.1662793551464,-1.,-1.77018771684844));
#24754=CARTESIAN_POINT('Ctrl Pts',(-0.168032772805197,-1.,-1.7869064998507));
#24755=CARTESIAN_POINT('Ctrl Pts',(-0.169936923904608,-1.,-1.80561530629706));
#24756=CARTESIAN_POINT('Ctrl Pts',(-0.171554770204119,-1.,-1.82215766811545));
#24757=CARTESIAN_POINT('Ctrl Pts',(-0.1728894428919,-1.,-1.83658380527692));
#24758=CARTESIAN_POINT('Ctrl Pts',(-0.173946627587731,-1.,-1.8489811319852));
#24759=CARTESIAN_POINT('Ctrl Pts',(-0.17473525927603,-1.,-1.85948367088837));
#24760=CARTESIAN_POINT('Ctrl Pts',(-0.175268337590758,-1.,-1.86828349694799));
#24761=CARTESIAN_POINT('Ctrl Pts',(-0.175563480746485,-1.,-1.87563767773588));
#24762=CARTESIAN_POINT('Ctrl Pts',(-0.175644148889699,-1.,-1.88188663145367));
#24763=CARTESIAN_POINT('Ctrl Pts',(-0.175538155840648,-1.,-1.88742606273259));
#24764=CARTESIAN_POINT('Ctrl Pts',(-0.175274276190844,-1.,-1.892646301985));
#24765=CARTESIAN_POINT('Ctrl Pts',(-0.174879405091263,-1.,-1.89788101117132));
#24766=CARTESIAN_POINT('Ctrl Pts',(-0.174375518661085,-1.,-1.90335253862834));
#24767=CARTESIAN_POINT('Ctrl Pts',(-0.173776635257817,-1.,-1.90911693975267));
#24768=CARTESIAN_POINT('Ctrl Pts',(-0.173090695383496,-1.,-1.91511429159527));
#24769=CARTESIAN_POINT('Ctrl Pts',(-0.172321621259514,-1.,-1.9212233439798));
#24770=CARTESIAN_POINT('Ctrl Pts',(-0.171471191532988,-1.,-1.92731093582036));
#24771=CARTESIAN_POINT('Ctrl Pts',(-0.170541253116202,-1.,-1.93329183155539));
#24772=CARTESIAN_POINT('Ctrl Pts',(-0.169534904817491,-1.,-1.93915639211581));
#24773=CARTESIAN_POINT('Ctrl Pts',(-0.168455741607556,-1.,-1.94493757756931));
#24774=CARTESIAN_POINT('Ctrl Pts',(-0.167307501784475,-1.,-1.95069027794294));
#24775=CARTESIAN_POINT('Ctrl Pts',(-0.166093592002812,-1.,-1.9564675971873));
#24776=CARTESIAN_POINT('Ctrl Pts',(-0.164816568920269,-1.,-1.96229379940136));
#24777=CARTESIAN_POINT('Ctrl Pts',(-0.163478185457734,-1.,-1.96816512677967));
#24778=CARTESIAN_POINT('Ctrl Pts',(-0.162079693556289,-1.,-1.97406280235188));
#24779=CARTESIAN_POINT('Ctrl Pts',(-0.160622060784611,-1.,-1.97996195437559));
#24780=CARTESIAN_POINT('Ctrl Pts',(-0.159106226437299,-1.,-1.98584238283292));
#24781=CARTESIAN_POINT('Ctrl Pts',(-0.157533331459227,-1.,-1.99169810931908));
#24782=CARTESIAN_POINT('Ctrl Pts',(-0.155904629548783,-1.,-1.99753284771497));
#24783=CARTESIAN_POINT('Ctrl Pts',(-0.154221403049722,-1.,-2.00335565310543));
#24784=CARTESIAN_POINT('Ctrl Pts',(-0.15248488362145,-1.,-2.00917680318424));
#24785=CARTESIAN_POINT('Ctrl Pts',(-0.150696157673078,-1.,-2.01500291940238));
#24786=CARTESIAN_POINT('Ctrl Pts',(-0.148856124775337,-1.,-2.02083464969894));
#24787=CARTESIAN_POINT('Ctrl Pts',(-0.146965557332583,-1.,-2.02666926182017));
#24788=CARTESIAN_POINT('Ctrl Pts',(-0.145025140186057,-1.,-2.03250223739942));
#24789=CARTESIAN_POINT('Ctrl Pts',(-0.143035515058209,-1.,-2.03832911025912));
#24790=CARTESIAN_POINT('Ctrl Pts',(-0.140997332152546,-1.,-2.04414757947916));
#24791=CARTESIAN_POINT('Ctrl Pts',(-0.138911255368966,-1.,-2.04995762001328));
#24792=CARTESIAN_POINT('Ctrl Pts',(-0.136777941218044,-1.,-2.05576044414264));
#24793=CARTESIAN_POINT('Ctrl Pts',(-0.134598026192106,-1.,-2.06155781517842));
#24794=CARTESIAN_POINT('Ctrl Pts',(-0.13237211154771,-1.,-2.06735123910326));
#24795=CARTESIAN_POINT('Ctrl Pts',(-0.130100748328403,-1.,-2.07314114713063));
#24796=CARTESIAN_POINT('Ctrl Pts',(-0.12778444527612,-1.,-2.07892715110987));
#24797=CARTESIAN_POINT('Ctrl Pts',(-0.125423679412061,-1.,-2.08470840653643));
#24798=CARTESIAN_POINT('Ctrl Pts',(-0.123018905621083,-1.,-2.09048392424825));
#24799=CARTESIAN_POINT('Ctrl Pts',(-0.120570567965122,-1.,-2.0962529286773));
#24800=CARTESIAN_POINT('Ctrl Pts',(-0.118079107988355,-1.,-2.102015121329));
#24801=CARTESIAN_POINT('Ctrl Pts',(-0.115544957687926,-1.,-2.10777050261309));
#24802=CARTESIAN_POINT('Ctrl Pts',(-0.112968534419737,-1.,-2.11351924490306));
#24803=CARTESIAN_POINT('Ctrl Pts',(-0.110350236135025,-1.,-2.11926155590865));
#24804=CARTESIAN_POINT('Ctrl Pts',(-0.10769043523109,-1.,-2.12499752307));
#24805=CARTESIAN_POINT('Ctrl Pts',(-0.104989479152739,-1.,-2.13072704887293));
#24806=CARTESIAN_POINT('Ctrl Pts',(-0.1022477005561,-1.,-2.13644992667165));
#24807=CARTESIAN_POINT('Ctrl Pts',(-0.0994654261990915,-1.,-2.14216588396025));
#24808=CARTESIAN_POINT('Ctrl Pts',(-0.0966429852305459,-1.,-2.14787463531795));
#24809=CARTESIAN_POINT('Ctrl Pts',(-0.0937807218867643,-1.,-2.1535759397817));
#24810=CARTESIAN_POINT('Ctrl Pts',(-0.0908789888107265,-1.,-2.15926961544516));
#24811=CARTESIAN_POINT('Ctrl Pts',(-0.0879381291386923,-1.,-2.16495552645014));
#24812=CARTESIAN_POINT('Ctrl Pts',(-0.0849584620835372,-1.,-2.17063357870952));
#24813=CARTESIAN_POINT('Ctrl Pts',(-0.0819402680872765,-1.,-2.176303712113));
#24814=CARTESIAN_POINT('Ctrl Pts',(-0.0788837727685243,-1.,-2.18196589448887));
#24815=CARTESIAN_POINT('Ctrl Pts',(-0.0757891465836148,-1.,-2.1876201139953));
#24816=CARTESIAN_POINT('Ctrl Pts',(-0.0732830357306725,-1.,-2.19213712013662));
#24817=CARTESIAN_POINT('Ctrl Pts',(-0.0713863779526154,-1.,-2.19552129484002));
#24818=CARTESIAN_POINT('Ctrl Pts',(-0.070114353632549,-1.,-2.19777582085423));
#24819=CARTESIAN_POINT('Ctrl Pts',(-0.0694764450219581,-1.,-2.19890268624765));
#24820=CARTESIAN_POINT('',(0.0694764450219584,-1.,-2.19890268624765));
#24821=CARTESIAN_POINT('',(-0.0694764450219581,-1.,-2.19890268624765));
#24822=CARTESIAN_POINT('',(0.163289472382896,-1.,-1.74236521665491));
#24823=CARTESIAN_POINT('Ctrl Pts',(0.0694764450219584,-1.,-2.19890268624765));
#24824=CARTESIAN_POINT('Ctrl Pts',(0.0701143536324926,-1.,-2.19777582085261));
#24825=CARTESIAN_POINT('Ctrl Pts',(0.0713863779524627,-1.,-2.19552129483562));
#24826=CARTESIAN_POINT('Ctrl Pts',(0.0732830357304276,-1.,-2.19213712012956));
#24827=CARTESIAN_POINT('Ctrl Pts',(0.0757891465833411,-1.,-2.1876201139874));
#24828=CARTESIAN_POINT('Ctrl Pts',(0.0788837727683228,-1.,-2.18196589448304));
#24829=CARTESIAN_POINT('Ctrl Pts',(0.0819402680871939,-1.,-2.1763037121106));
#24830=CARTESIAN_POINT('Ctrl Pts',(0.0849584620835643,-1.,-2.17063357871031));
#24831=CARTESIAN_POINT('Ctrl Pts',(0.0879381291387823,-1.,-2.16495552645275));
#24832=CARTESIAN_POINT('Ctrl Pts',(0.0908789888108266,-1.,-2.15926961544808));
#24833=CARTESIAN_POINT('Ctrl Pts',(0.0937807218868345,-1.,-2.15357593978377));
#24834=CARTESIAN_POINT('Ctrl Pts',(0.0966429852305689,-1.,-2.14787463531864));
#24835=CARTESIAN_POINT('Ctrl Pts',(0.0994654261990743,-1.,-2.14216588395974));
#24836=CARTESIAN_POINT('Ctrl Pts',(0.102247700556064,-1.,-2.13644992667052));
#24837=CARTESIAN_POINT('Ctrl Pts',(0.104989479152703,-1.,-2.1307270488718));
#24838=CARTESIAN_POINT('Ctrl Pts',(0.107690435231068,-1.,-2.12499752306927));
#24839=CARTESIAN_POINT('Ctrl Pts',(0.11035023613502,-1.,-2.11926155590849));
#24840=CARTESIAN_POINT('Ctrl Pts',(0.112968534419746,-1.,-2.11351924490335));
#24841=CARTESIAN_POINT('Ctrl Pts',(0.11554495768794,-1.,-2.10777050261359));
#24842=CARTESIAN_POINT('Ctrl Pts',(0.118079107988368,-1.,-2.10201512132945));
#24843=CARTESIAN_POINT('Ctrl Pts',(0.120570567965129,-1.,-2.09625292867756));
#24844=CARTESIAN_POINT('Ctrl Pts',(0.123018905621083,-1.,-2.09048392424826));
#24845=CARTESIAN_POINT('Ctrl Pts',(0.125423679412058,-1.,-2.08470840653628));
#24846=CARTESIAN_POINT('Ctrl Pts',(0.127784445276116,-1.,-2.07892715110967));
#24847=CARTESIAN_POINT('Ctrl Pts',(0.1301007483284,-1.,-2.07314114713047));
#24848=CARTESIAN_POINT('Ctrl Pts',(0.13237211154771,-1.,-2.06735123910319));
#24849=CARTESIAN_POINT('Ctrl Pts',(0.134598026192107,-1.,-2.06155781517844));
#24850=CARTESIAN_POINT('Ctrl Pts',(0.136777941218044,-1.,-2.0557604441427));
#24851=CARTESIAN_POINT('Ctrl Pts',(0.138911255368966,-1.,-2.04995762001333));
#24852=CARTESIAN_POINT('Ctrl Pts',(0.140997332152545,-1.,-2.04414757947919));
#24853=CARTESIAN_POINT('Ctrl Pts',(0.143035515058208,-1.,-2.03832911025913));
#24854=CARTESIAN_POINT('Ctrl Pts',(0.145025140186058,-1.,-2.03250223739941));
#24855=CARTESIAN_POINT('Ctrl Pts',(0.146965557332586,-1.,-2.02666926182017));
#24856=CARTESIAN_POINT('Ctrl Pts',(0.148856124775343,-1.,-2.02083464969897));
#24857=CARTESIAN_POINT('Ctrl Pts',(0.150696157673084,-1.,-2.01500291940243));
#24858=CARTESIAN_POINT('Ctrl Pts',(0.152484883621452,-1.,-2.00917680318426));
#24859=CARTESIAN_POINT('Ctrl Pts',(0.154221403049719,-1.,-2.00335565310539));
#24860=CARTESIAN_POINT('Ctrl Pts',(0.155904629548774,-1.,-1.99753284771487));
#24861=CARTESIAN_POINT('Ctrl Pts',(0.157533331459215,-1.,-1.99169810931893));
#24862=CARTESIAN_POINT('Ctrl Pts',(0.159106226437288,-1.,-1.98584238283279));
#24863=CARTESIAN_POINT('Ctrl Pts',(0.16062206078461,-1.,-1.97996195437557));
#24864=CARTESIAN_POINT('Ctrl Pts',(0.162079693556302,-1.,-1.97406280235204));
#24865=CARTESIAN_POINT('Ctrl Pts',(0.16347818545776,-1.,-1.96816512678));
#24866=CARTESIAN_POINT('Ctrl Pts',(0.1648165689203,-1.,-1.96229379940174));
#24867=CARTESIAN_POINT('Ctrl Pts',(0.166093592002833,-1.,-1.95646759718755));
#24868=CARTESIAN_POINT('Ctrl Pts',(0.167307501784469,-1.,-1.95069027794286));
#24869=CARTESIAN_POINT('Ctrl Pts',(0.168455741607516,-1.,-1.94493757756879));
#24870=CARTESIAN_POINT('Ctrl Pts',(0.169534904817425,-1.,-1.93915639211497));
#24871=CARTESIAN_POINT('Ctrl Pts',(0.170541253116136,-1.,-1.93329183155455));
#24872=CARTESIAN_POINT('Ctrl Pts',(0.17147119153296,-1.,-1.92731093582));
#24873=CARTESIAN_POINT('Ctrl Pts',(0.172321621259557,-1.,-1.92122334398034));
#24874=CARTESIAN_POINT('Ctrl Pts',(0.173090695383619,-1.,-1.91511429159681));
#24875=CARTESIAN_POINT('Ctrl Pts',(0.173776635257984,-1.,-1.90911693975475));
#24876=CARTESIAN_POINT('Ctrl Pts',(0.174375518661222,-1.,-1.90335253863003));
#24877=CARTESIAN_POINT('Ctrl Pts',(0.174879405091277,-1.,-1.89788101117148));
#24878=CARTESIAN_POINT('Ctrl Pts',(0.175274276190664,-1.,-1.89264630198279));
#24879=CARTESIAN_POINT('Ctrl Pts',(0.175538155840286,-1.,-1.88742606272818));
#24880=CARTESIAN_POINT('Ctrl Pts',(0.175644148889271,-1.,-1.88188663144846));
#24881=CARTESIAN_POINT('Ctrl Pts',(0.175563480746205,-1.,-1.87563767773249));
#24882=CARTESIAN_POINT('Ctrl Pts',(0.175268337590901,-1.,-1.86828349694972));
#24883=CARTESIAN_POINT('Ctrl Pts',(0.174735259276856,-1.,-1.85948367089838));
#24884=CARTESIAN_POINT('Ctrl Pts',(0.173946627589401,-1.,-1.84898113200543));
#24885=CARTESIAN_POINT('Ctrl Pts',(0.17288944289442,-1.,-1.83658380530747));
#24886=CARTESIAN_POINT('Ctrl Pts',(0.171554770207306,-1.,-1.82215766815414));
#24887=CARTESIAN_POINT('Ctrl Pts',(0.169936923908078,-1.,-1.80561530633924));
#24888=CARTESIAN_POINT('Ctrl Pts',(0.16803277280837,-1.,-1.78690649988931));
#24889=CARTESIAN_POINT('Ctrl Pts',(0.166279355148738,-1.,-1.77018771687692));
#24890=CARTESIAN_POINT('Ctrl Pts',(0.164834765708484,-1.,-1.75666056640041));
#24891=CARTESIAN_POINT('Ctrl Pts',(0.163814161002474,-1.,-1.74720349503904));
#24892=CARTESIAN_POINT('Ctrl Pts',(0.163289472382896,-1.,-1.74236521665491));
#24893=CARTESIAN_POINT('',(0.383122945602004,-1.,-1.7075470150345));
#24894=CARTESIAN_POINT('Origin',(0.,-1.,0.));
#24895=CARTESIAN_POINT('',(0.61342227326009,-1.,-2.11275013067528));
#24896=CARTESIAN_POINT('Ctrl Pts',(0.383122945602004,-1.,-1.7075470150345));
#24897=CARTESIAN_POINT('Ctrl Pts',(0.384119047314215,-1.,-1.71231062891398));
#24898=CARTESIAN_POINT('Ctrl Pts',(0.386070790323281,-1.,-1.72162022244582));
#24899=CARTESIAN_POINT('Ctrl Pts',(0.388877023502615,-1.,-1.73493170972829));
#24900=CARTESIAN_POINT('Ctrl Pts',(0.392375812285395,-1.,-1.75137405310193));
#24901=CARTESIAN_POINT('Ctrl Pts',(0.396346196110688,-1.,-1.76975560043442));
#24902=CARTESIAN_POINT('Ctrl Pts',(0.399919403774155,-1.,-1.78598826343754));
#24903=CARTESIAN_POINT('Ctrl Pts',(0.403107976163396,-1.,-1.80012077173238));
#24904=CARTESIAN_POINT('Ctrl Pts',(0.405933518407175,-1.,-1.81223801812013));
#24905=CARTESIAN_POINT('Ctrl Pts',(0.408428948106227,-1.,-1.82247022677562));
#24906=CARTESIAN_POINT('Ctrl Pts',(0.410641256301276,-1.,-1.83100408895047));
#24907=CARTESIAN_POINT('Ctrl Pts',(0.412633125322945,-1.,-1.8380895347617));
#24908=CARTESIAN_POINT('Ctrl Pts',(0.414487438255542,-1.,-1.84405757074218));
#24909=CARTESIAN_POINT('Ctrl Pts',(0.416300022039885,-1.,-1.84929312930314));
#24910=CARTESIAN_POINT('Ctrl Pts',(0.418164129144045,-1.,-1.8541763285645));
#24911=CARTESIAN_POINT('Ctrl Pts',(0.420157287975583,-1.,-1.8590328109667));
#24912=CARTESIAN_POINT('Ctrl Pts',(0.422327307417884,-1.,-1.86408083333863));
#24913=CARTESIAN_POINT('Ctrl Pts',(0.424678177290876,-1.,-1.8693780394412));
#24914=CARTESIAN_POINT('Ctrl Pts',(0.427183828518743,-1.,-1.87486989291334));
#24915=CARTESIAN_POINT('Ctrl Pts',(0.429803062482217,-1.,-1.88044229001779));
#24916=CARTESIAN_POINT('Ctrl Pts',(0.432493038548833,-1.,-1.88596913666828));
#24917=CARTESIAN_POINT('Ctrl Pts',(0.43522566096358,-1.,-1.89136993975585));
#24918=CARTESIAN_POINT('Ctrl Pts',(0.437995003948443,-1.,-1.89663648956549));
#24919=CARTESIAN_POINT('Ctrl Pts',(0.44080783370416,-1.,-1.90180124389137));
#24920=CARTESIAN_POINT('Ctrl Pts',(0.44367755684917,-1.,-1.90691756144906));
#24921=CARTESIAN_POINT('Ctrl Pts',(0.446617343485651,-1.,-1.91203699981095));
#24922=CARTESIAN_POINT('Ctrl Pts',(0.449632260106572,-1.,-1.91718342555717));
#24923=CARTESIAN_POINT('Ctrl Pts',(0.452719478359356,-1.,-1.9223538064847));
#24924=CARTESIAN_POINT('Ctrl Pts',(0.455872005174335,-1.,-1.92753067150461));
#24925=CARTESIAN_POINT('Ctrl Pts',(0.459081234547931,-1.,-1.93269066517936));
#24926=CARTESIAN_POINT('Ctrl Pts',(0.462340031009087,-1.,-1.93781486640834));
#24927=CARTESIAN_POINT('Ctrl Pts',(0.465645462026064,-1.,-1.94289794196205));
#24928=CARTESIAN_POINT('Ctrl Pts',(0.468997482913158,-1.,-1.94794381136524));
#24929=CARTESIAN_POINT('Ctrl Pts',(0.472397672264079,-1.,-1.95296148278136));
#24930=CARTESIAN_POINT('Ctrl Pts',(0.475848034683171,-1.,-1.95796111148175));
#24931=CARTESIAN_POINT('Ctrl Pts',(0.479349583074846,-1.,-1.96294933055938));
#24932=CARTESIAN_POINT('Ctrl Pts',(0.482901662120686,-1.,-1.96792703422358));
#24933=CARTESIAN_POINT('Ctrl Pts',(0.486502692907661,-1.,-1.97289186263272));
#24934=CARTESIAN_POINT('Ctrl Pts',(0.490150627860955,-1.,-1.97783973019229));
#24935=CARTESIAN_POINT('Ctrl Pts',(0.493843476541492,-1.,-1.9827665876182));
#24936=CARTESIAN_POINT('Ctrl Pts',(0.497579909545564,-1.,-1.98767044752929));
#24937=CARTESIAN_POINT('Ctrl Pts',(0.501359287727129,-1.,-1.9925514912615));
#24938=CARTESIAN_POINT('Ctrl Pts',(0.505181361323011,-1.,-1.99741107463567));
#24939=CARTESIAN_POINT('Ctrl Pts',(0.509046069886152,-1.,-2.00225107134733));
#24940=CARTESIAN_POINT('Ctrl Pts',(0.512953306961813,-1.,-2.00707309946955));
#24941=CARTESIAN_POINT('Ctrl Pts',(0.516902681728733,-1.,-2.01187773939257));
#24942=CARTESIAN_POINT('Ctrl Pts',(0.520893590399428,-1.,-2.01666477917306));
#24943=CARTESIAN_POINT('Ctrl Pts',(0.524925318333518,-1.,-2.02143356304712));
#24944=CARTESIAN_POINT('Ctrl Pts',(0.52899712724191,-1.,-2.02618329083289));
#24945=CARTESIAN_POINT('Ctrl Pts',(0.533108355132905,-1.,-2.03091336214401));
#24946=CARTESIAN_POINT('Ctrl Pts',(0.537258489833134,-1.,-2.03562362953993));
#24947=CARTESIAN_POINT('Ctrl Pts',(0.54144712061552,-1.,-2.0403142269048));
#24948=CARTESIAN_POINT('Ctrl Pts',(0.545673903817348,-1.,-2.0449854471456));
#24949=CARTESIAN_POINT('Ctrl Pts',(0.549938525150342,-1.,-2.04963761077974));
#24950=CARTESIAN_POINT('Ctrl Pts',(0.554240657464109,-1.,-2.05427091604482));
#24951=CARTESIAN_POINT('Ctrl Pts',(0.558579940185467,-1.,-2.05888537756571));
#24952=CARTESIAN_POINT('Ctrl Pts',(0.562955993082574,-1.,-2.06348090160697));
#24953=CARTESIAN_POINT('Ctrl Pts',(0.567368421181229,-1.,-2.06805732997383));
#24954=CARTESIAN_POINT('Ctrl Pts',(0.571816823242411,-1.,-2.07261449292758));
#24955=CARTESIAN_POINT('Ctrl Pts',(0.576300797416274,-1.,-2.07715226767361));
#24956=CARTESIAN_POINT('Ctrl Pts',(0.580819952107256,-1.,-2.08167059018138));
#24957=CARTESIAN_POINT('Ctrl Pts',(0.585373918990895,-1.,-2.086169437277));
#24958=CARTESIAN_POINT('Ctrl Pts',(0.589962365403189,-1.,-2.09064881812053));
#24959=CARTESIAN_POINT('Ctrl Pts',(0.594585006052823,-1.,-2.09510876220501));
#24960=CARTESIAN_POINT('Ctrl Pts',(0.599241616422144,-1.,-2.09954930865331));
#24961=CARTESIAN_POINT('Ctrl Pts',(0.603932030738212,-1.,-2.10397049887709));
#24962=CARTESIAN_POINT('Ctrl Pts',(0.607711315456826,-1.,-2.10749199615859));
#24963=CARTESIAN_POINT('Ctrl Pts',(0.610560911691113,-1.,-2.11012443807661));
#24964=CARTESIAN_POINT('Ctrl Pts',(0.61246736556225,-1.,-2.11187554260142));
#24965=CARTESIAN_POINT('Ctrl Pts',(0.61342227326009,-1.,-2.11275013067528));
#24966=CARTESIAN_POINT('',(0.745574324794401,-1.,-2.0698113262342));
#24967=CARTESIAN_POINT('',(0.61342227326009,-1.,-2.11275013067528));
#24968=CARTESIAN_POINT('',(0.693717979106306,-1.,-1.60662857109684));
#24969=CARTESIAN_POINT('Ctrl Pts',(0.745574324794401,-1.,-2.0698113262342));
#24970=CARTESIAN_POINT('Ctrl Pts',(0.74583279137781,-1.,-2.06854248895575));
#24971=CARTESIAN_POINT('Ctrl Pts',(0.746345871542695,-1.,-2.06600523016401));
#24972=CARTESIAN_POINT('Ctrl Pts',(0.747103932785504,-1.,-2.06220058927162));
#24973=CARTESIAN_POINT('Ctrl Pts',(0.748091554181101,-1.,-2.05713023030263));
#24974=CARTESIAN_POINT('Ctrl Pts',(0.749287468663053,-1.,-2.05079645591606));
#24975=CARTESIAN_POINT('Ctrl Pts',(0.750444657874758,-1.,-2.04446689147754));
#24976=CARTESIAN_POINT('Ctrl Pts',(0.751562963361383,-1.,-2.03814160092173));
#24977=CARTESIAN_POINT('Ctrl Pts',(0.752642180488104,-1.,-2.03182068456467));
#24978=CARTESIAN_POINT('Ctrl Pts',(0.753682061113765,-1.,-2.02550428623587));
#24979=CARTESIAN_POINT('Ctrl Pts',(0.75468233072352,-1.,-2.01919259406003));
#24980=CARTESIAN_POINT('Ctrl Pts',(0.7556427049581,-1.,-2.01288584328149));
#24981=CARTESIAN_POINT('Ctrl Pts',(0.756562904646496,-1.,-2.00658431587682));
#24982=CARTESIAN_POINT('Ctrl Pts',(0.757442676862341,-1.,-2.00028834739072));
#24983=CARTESIAN_POINT('Ctrl Pts',(0.758281796766377,-1.,-1.9939983109871));
#24984=CARTESIAN_POINT('Ctrl Pts',(0.759080037802242,-1.,-1.98771456680806));
#24985=CARTESIAN_POINT('Ctrl Pts',(0.759837147452135,-1.,-1.98143741418156));
#24986=CARTESIAN_POINT('Ctrl Pts',(0.760552825409855,-1.,-1.97516705321521));
#24987=CARTESIAN_POINT('Ctrl Pts',(0.761226690483986,-1.,-1.96890351582545));
#24988=CARTESIAN_POINT('Ctrl Pts',(0.761858300014575,-1.,-1.96264672744229));
#24989=CARTESIAN_POINT('Ctrl Pts',(0.762447203806263,-1.,-1.95639665309893));
#24990=CARTESIAN_POINT('Ctrl Pts',(0.762992990878774,-1.,-1.95015342590025));
#24991=CARTESIAN_POINT('Ctrl Pts',(0.76349533353858,-1.,-1.94391746617626));
#24992=CARTESIAN_POINT('Ctrl Pts',(0.763954049121393,-1.,-1.93768964875867));
#24993=CARTESIAN_POINT('Ctrl Pts',(0.764369010673889,-1.,-1.93147105496367));
#24994=CARTESIAN_POINT('Ctrl Pts',(0.764740025488189,-1.,-1.92526263537041));
#24995=CARTESIAN_POINT('Ctrl Pts',(0.765066729667095,-1.,-1.91906491634197));
#24996=CARTESIAN_POINT('Ctrl Pts',(0.765348465884739,-1.,-1.91287765805174));
#24997=CARTESIAN_POINT('Ctrl Pts',(0.765584196937936,-1.,-1.90669961402362));
#24998=CARTESIAN_POINT('Ctrl Pts',(0.765772772593395,-1.,-1.90052930393599));
#24999=CARTESIAN_POINT('Ctrl Pts',(0.765913193856979,-1.,-1.89436577771389));
#25000=CARTESIAN_POINT('Ctrl Pts',(0.76600483706209,-1.,-1.88820926433409));
#25001=CARTESIAN_POINT('Ctrl Pts',(0.766047794851868,-1.,-1.88206215302561));
#25002=CARTESIAN_POINT('Ctrl Pts',(0.766042837036759,-1.,-1.87592888967886));
#25003=CARTESIAN_POINT('Ctrl Pts',(0.765990708546111,-1.,-1.86981398314345));
#25004=CARTESIAN_POINT('Ctrl Pts',(0.765891519092557,-1.,-1.86372027063315));
#25005=CARTESIAN_POINT('Ctrl Pts',(0.765744212909305,-1.,-1.85764741390391));
#25006=CARTESIAN_POINT('Ctrl Pts',(0.765545710619023,-1.,-1.85158945130054));
#25007=CARTESIAN_POINT('Ctrl Pts',(0.765291664861971,-1.,-1.84553698875911));
#25008=CARTESIAN_POINT('Ctrl Pts',(0.764978057881687,-1.,-1.83948181064823));
#25009=CARTESIAN_POINT('Ctrl Pts',(0.764602549687845,-1.,-1.8334207722714));
#25010=CARTESIAN_POINT('Ctrl Pts',(0.764165902606055,-1.,-1.8273599120008));
#25011=CARTESIAN_POINT('Ctrl Pts',(0.763673465462854,-1.,-1.82131873145297));
#25012=CARTESIAN_POINT('Ctrl Pts',(0.763132003836783,-1.,-1.81532118405566));
#25013=CARTESIAN_POINT('Ctrl Pts',(0.762546129464036,-1.,-1.80938551463989));
#25014=CARTESIAN_POINT('Ctrl Pts',(0.761915336443515,-1.,-1.80351583877334));
#25015=CARTESIAN_POINT('Ctrl Pts',(0.761229695230359,-1.,-1.79768986997735));
#25016=CARTESIAN_POINT('Ctrl Pts',(0.760469555880425,-1.,-1.79185815610802));
#25017=CARTESIAN_POINT('Ctrl Pts',(0.759614401109868,-1.,-1.78596964884527));
#25018=CARTESIAN_POINT('Ctrl Pts',(0.75865062667738,-1.,-1.77999411220912));
#25019=CARTESIAN_POINT('Ctrl Pts',(0.757578264077238,-1.,-1.77394167108342));
#25020=CARTESIAN_POINT('Ctrl Pts',(0.756421896028403,-1.,-1.76789396003141));
#25021=CARTESIAN_POINT('Ctrl Pts',(0.755220979975262,-1.,-1.7619781724032));
#25022=CARTESIAN_POINT('Ctrl Pts',(0.75400925402848,-1.,-1.75631083600175));
#25023=CARTESIAN_POINT('Ctrl Pts',(0.752797683531377,-1.,-1.75095139468809));
#25024=CARTESIAN_POINT('Ctrl Pts',(0.751555614163629,-1.,-1.74585086852298));
#25025=CARTESIAN_POINT('Ctrl Pts',(0.75019343597954,-1.,-1.74080458266705));
#25026=CARTESIAN_POINT('Ctrl Pts',(0.748582462954854,-1.,-1.73550351679848));
#25027=CARTESIAN_POINT('Ctrl Pts',(0.746574710096436,-1.,-1.72958533647399));
#25028=CARTESIAN_POINT('Ctrl Pts',(0.744021445433764,-1.,-1.7226822991693));
#25029=CARTESIAN_POINT('Ctrl Pts',(0.740795162032087,-1.,-1.71447789751927));
#25030=CARTESIAN_POINT('Ctrl Pts',(0.736799665724771,-1.,-1.70473309006121));
#25031=CARTESIAN_POINT('Ctrl Pts',(0.731963238697195,-1.,-1.69326921975743));
#25032=CARTESIAN_POINT('Ctrl Pts',(0.726235967997433,-1.,-1.67996158455503));
#25033=CARTESIAN_POINT('Ctrl Pts',(0.719585433804282,-1.,-1.6647288055568));
#25034=CARTESIAN_POINT('Ctrl Pts',(0.711993139355394,-1.,-1.64752408832016));
#25035=CARTESIAN_POINT('Ctrl Pts',(0.705159151988319,-1.,-1.63216541664676));
#25036=CARTESIAN_POINT('Ctrl Pts',(0.699605146405088,-1.,-1.61974673472612));
#25037=CARTESIAN_POINT('Ctrl Pts',(0.695712097881194,-1.,-1.61106790958151));
#25038=CARTESIAN_POINT('Ctrl Pts',(0.693717979106306,-1.,-1.60662857109684));
#25039=CARTESIAN_POINT('',(0.892032620296855,-1.,-1.5055822144029));
#25040=CARTESIAN_POINT('Origin',(0.,-1.,0.));
#25041=CARTESIAN_POINT('',(1.23627494547115,-1.,-1.81978687191668));
#25042=CARTESIAN_POINT('Ctrl Pts',(0.892032620296855,-1.,-1.5055822144029));
#25043=CARTESIAN_POINT('Ctrl Pts',(0.894452006964543,-1.,-1.50980486806688));
#25044=CARTESIAN_POINT('Ctrl Pts',(0.89918504748351,-1.,-1.51805569590094));
#25045=CARTESIAN_POINT('Ctrl Pts',(0.905967409625651,-1.,-1.52984849887993));
#25046=CARTESIAN_POINT('Ctrl Pts',(0.914375919026456,-1.,-1.54440491149498));
#25047=CARTESIAN_POINT('Ctrl Pts',(0.923832188944341,-1.,-1.56065988578893));
#25048=CARTESIAN_POINT('Ctrl Pts',(0.932246680108685,-1.,-1.57499388382243));
#25049=CARTESIAN_POINT('Ctrl Pts',(0.939646377893399,-1.,-1.58744937487176));
#25050=CARTESIAN_POINT('Ctrl Pts',(0.946078063315257,-1.,-1.59810042043673));
#25051=CARTESIAN_POINT('Ctrl Pts',(0.951613284356035,-1.,-1.60706069896936));
#25052=CARTESIAN_POINT('Ctrl Pts',(0.95635442292067,-1.,-1.61449324337085));
#25053=CARTESIAN_POINT('Ctrl Pts',(0.960438326101728,-1.,-1.62061638140221));
#25054=CARTESIAN_POINT('Ctrl Pts',(0.964046107040535,-1.,-1.62571930670187));
#25055=CARTESIAN_POINT('Ctrl Pts',(0.967387853230345,-1.,-1.63013849959462));
#25056=CARTESIAN_POINT('Ctrl Pts',(0.970669715997509,-1.,-1.63420665729798));
#25057=CARTESIAN_POINT('Ctrl Pts',(0.974066058287418,-1.,-1.63820952658144));
#25058=CARTESIAN_POINT('Ctrl Pts',(0.977689794119416,-1.,-1.64233990826687));
#25059=CARTESIAN_POINT('Ctrl Pts',(0.981562530939489,-1.,-1.64665139190656));
#25060=CARTESIAN_POINT('Ctrl Pts',(0.98564262292082,-1.,-1.65110016612638));
#25061=CARTESIAN_POINT('Ctrl Pts',(0.989855627854164,-1.,-1.65559044289699));
#25062=CARTESIAN_POINT('Ctrl Pts',(0.994121836661305,-1.,-1.66001553809947));
#25063=CARTESIAN_POINT('Ctrl Pts',(0.998389654952757,-1.,-1.66430758030376));
#25064=CARTESIAN_POINT('Ctrl Pts',(1.00265091003727,-1.,-1.66846059277303));
#25065=CARTESIAN_POINT('Ctrl Pts',(1.00692206696414,-1.,-1.67250335383293));
#25066=CARTESIAN_POINT('Ctrl Pts',(1.01123236493511,-1.,-1.67648246776464));
#25067=CARTESIAN_POINT('Ctrl Pts',(1.01561026162773,-1.,-1.68044289894798));
#25068=CARTESIAN_POINT('Ctrl Pts',(1.02006795074201,-1.,-1.68440578021706));
#25069=CARTESIAN_POINT('Ctrl Pts',(1.02460180535255,-1.,-1.68836910178447));
#25070=CARTESIAN_POINT('Ctrl Pts',(1.02919977579147,-1.,-1.69231840863458));
#25071=CARTESIAN_POINT('Ctrl Pts',(1.03384646003588,-1.,-1.69623414782771));
#25072=CARTESIAN_POINT('Ctrl Pts',(1.03852922490789,-1.,-1.70010052930962));
#25073=CARTESIAN_POINT('Ctrl Pts',(1.04324363334554,-1.,-1.70391338707982));
#25074=CARTESIAN_POINT('Ctrl Pts',(1.04799085404995,-1.,-1.70767646263649));
#25075=CARTESIAN_POINT('Ctrl Pts',(1.05277517202855,-1.,-1.71139783543989));
#25076=CARTESIAN_POINT('Ctrl Pts',(1.05760163192479,-1.,-1.7150865442702));
#25077=CARTESIAN_POINT('Ctrl Pts',(1.06247324680647,-1.,-1.71874858456904));
#25078=CARTESIAN_POINT('Ctrl Pts',(1.06738966975462,-1.,-1.72238500928453));
#25079=CARTESIAN_POINT('Ctrl Pts',(1.07234866990252,-1.,-1.72599406198488));
#25080=CARTESIAN_POINT('Ctrl Pts',(1.0773470373727,-1.,-1.72957248977424));
#25081=CARTESIAN_POINT('Ctrl Pts',(1.08238162784749,-1.,-1.73311705663407));
#25082=CARTESIAN_POINT('Ctrl Pts',(1.08745056285427,-1.,-1.73662628326091));
#25083=CARTESIAN_POINT('Ctrl Pts',(1.09255329056493,-1.,-1.74010053962247));
#25084=CARTESIAN_POINT('Ctrl Pts',(1.09768999241225,-1.,-1.74354119236208));
#25085=CARTESIAN_POINT('Ctrl Pts',(1.10286118991143,-1.,-1.74695004214923));
#25086=CARTESIAN_POINT('Ctrl Pts',(1.10806728183007,-1.,-1.7503286607592));
#25087=CARTESIAN_POINT('Ctrl Pts',(1.11330807582551,-1.,-1.7536777209463));
#25088=CARTESIAN_POINT('Ctrl Pts',(1.11858293216763,-1.,-1.75699720772105));
#25089=CARTESIAN_POINT('Ctrl Pts',(1.12389096855086,-1.,-1.76028671825096));
#25090=CARTESIAN_POINT('Ctrl Pts',(1.12923123555075,-1.,-1.7635457196617));
#25091=CARTESIAN_POINT('Ctrl Pts',(1.1346029180462,-1.,-1.76677384551862));
#25092=CARTESIAN_POINT('Ctrl Pts',(1.14000548336975,-1.,-1.76997111386769));
#25093=CARTESIAN_POINT('Ctrl Pts',(1.1454385822692,-1.,-1.77313777896194));
#25094=CARTESIAN_POINT('Ctrl Pts',(1.15090197841514,-1.,-1.7762742255701));
#25095=CARTESIAN_POINT('Ctrl Pts',(1.15639547194698,-1.,-1.77938085564275));
#25096=CARTESIAN_POINT('Ctrl Pts',(1.16191881298499,-1.,-1.78245795881009));
#25097=CARTESIAN_POINT('Ctrl Pts',(1.16747166312303,-1.,-1.78550566040443));
#25098=CARTESIAN_POINT('Ctrl Pts',(1.17305363177328,-1.,-1.78852398877617));
#25099=CARTESIAN_POINT('Ctrl Pts',(1.17866429440809,-1.,-1.79151291552689));
#25100=CARTESIAN_POINT('Ctrl Pts',(1.18430321697432,-1.,-1.79447240321515));
#25101=CARTESIAN_POINT('Ctrl Pts',(1.18996997934445,-1.,-1.79740245923478));
#25102=CARTESIAN_POINT('Ctrl Pts',(1.19566418930242,-1.,-1.80030314369879));
#25103=CARTESIAN_POINT('Ctrl Pts',(1.20138548938974,-1.,-1.80317454838603));
#25104=CARTESIAN_POINT('Ctrl Pts',(1.20713356605475,-1.,-1.80601678480707));
#25105=CARTESIAN_POINT('Ctrl Pts',(1.21290815708314,-1.,-1.80882996917129));
#25106=CARTESIAN_POINT('Ctrl Pts',(1.21870906103557,-1.,-1.81161420806656));
#25107=CARTESIAN_POINT('Ctrl Pts',(1.2245361330495,-1.,-1.81436959210434));
#25108=CARTESIAN_POINT('Ctrl Pts',(1.2292186489137,-1.,-1.8165508718364));
#25109=CARTESIAN_POINT('Ctrl Pts',(1.2327422452705,-1.,-1.81817389921279));
#25110=CARTESIAN_POINT('Ctrl Pts',(1.23509651170476,-1.,-1.81925017193666));
#25111=CARTESIAN_POINT('Ctrl Pts',(1.23627494547115,-1.,-1.81978687191668));
#25112=CARTESIAN_POINT('',(1.34869019493419,-1.,-1.73811241238545));
#25113=CARTESIAN_POINT('',(1.23627494547115,-1.,-1.81978687191668));
#25114=CARTESIAN_POINT('',(1.15624053661742,-1.,-1.31362392696032));
#25115=CARTESIAN_POINT('Ctrl Pts',(1.34869019493419,-1.,-1.73811241238545));
#25116=CARTESIAN_POINT('Ctrl Pts',(1.34854391898045,-1.,-1.73682580585691));
#25117=CARTESIAN_POINT('Ctrl Pts',(1.34824783112887,-1.,-1.73425417885907));
#25118=CARTESIAN_POINT('Ctrl Pts',(1.34779309152035,-1.,-1.7304014965394));
#25119=CARTESIAN_POINT('Ctrl Pts',(1.34716554819527,-1.,-1.72527410680674));
#25120=CARTESIAN_POINT('Ctrl Pts',(1.34634568653227,-1.,-1.7188807715049));
#25121=CARTESIAN_POINT('Ctrl Pts',(1.34549029589416,-1.,-1.71250340686822));
#25122=CARTESIAN_POINT('Ctrl Pts',(1.34459924533831,-1.,-1.70614212266738));
#25123=CARTESIAN_POINT('Ctrl Pts',(1.34367237124483,-1.,-1.69979707754427));
#25124=CARTESIAN_POINT('Ctrl Pts',(1.34270948206319,-1.,-1.6934684849687));
#25125=CARTESIAN_POINT('Ctrl Pts',(1.341710374848,-1.,-1.68715660868764));
#25126=CARTESIAN_POINT('Ctrl Pts',(1.34067485185203,-1.,-1.68086176030362));
#25127=CARTESIAN_POINT('Ctrl Pts',(1.3396027347034,-1.,-1.67458429426086));
#25128=CARTESIAN_POINT('Ctrl Pts',(1.33849388654388,-1.,-1.66832460783989));
#25129=CARTESIAN_POINT('Ctrl Pts',(1.33734820885262,-1.,-1.66208312541983));
#25130=CARTESIAN_POINT('Ctrl Pts',(1.33616559745172,-1.,-1.65586025952593));
#25131=CARTESIAN_POINT('Ctrl Pts',(1.33494590467993,-1.,-1.6496563728683));
#25132=CARTESIAN_POINT('Ctrl Pts',(1.33368890676572,-1.,-1.6434717485603));
#25133=CARTESIAN_POINT('Ctrl Pts',(1.33239425103724,-1.,-1.63730653475089));
#25134=CARTESIAN_POINT('Ctrl Pts',(1.33106149345645,-1.,-1.63116079730923));
#25135=CARTESIAN_POINT('Ctrl Pts',(1.3296901950568,-1.,-1.62503464209797));
#25136=CARTESIAN_POINT('Ctrl Pts',(1.32828000610449,-1.,-1.61892832270724));
#25137=CARTESIAN_POINT('Ctrl Pts',(1.32683074483356,-1.,-1.6128423401575));
#25138=CARTESIAN_POINT('Ctrl Pts',(1.32534250785782,-1.,-1.60677758290954));
#25139=CARTESIAN_POINT('Ctrl Pts',(1.32381550858256,-1.,-1.60073511858687));
#25140=CARTESIAN_POINT('Ctrl Pts',(1.32224985747682,-1.,-1.59471591079403));
#25141=CARTESIAN_POINT('Ctrl Pts',(1.32064537110892,-1.,-1.58872057258245));
#25142=CARTESIAN_POINT('Ctrl Pts',(1.31900135021432,-1.,-1.58274907898834));
#25143=CARTESIAN_POINT('Ctrl Pts',(1.31731642317187,-1.,-1.5768005650559));
#25144=CARTESIAN_POINT('Ctrl Pts',(1.31558903860016,-1.,-1.57087397835723));
#25145=CARTESIAN_POINT('Ctrl Pts',(1.31381795281002,-1.,-1.56496872402353));
#25146=CARTESIAN_POINT('Ctrl Pts',(1.31200264341696,-1.,-1.55908521254821));
#25147=CARTESIAN_POINT('Ctrl Pts',(1.31014393684222,-1.,-1.55322568759481));
#25148=CARTESIAN_POINT('Ctrl Pts',(1.30824393907473,-1.,-1.54739413957185));
#25149=CARTESIAN_POINT('Ctrl Pts',(1.30630475189556,-1.,-1.54159462645432));
#25150=CARTESIAN_POINT('Ctrl Pts',(1.30432735639489,-1.,-1.53582981268977));
#25151=CARTESIAN_POINT('Ctrl Pts',(1.30231064395568,-1.,-1.53009970283891));
#25152=CARTESIAN_POINT('Ctrl Pts',(1.30024984366328,-1.,-1.52439957861062));
#25153=CARTESIAN_POINT('Ctrl Pts',(1.29813791800747,-1.,-1.51872184912724));
#25154=CARTESIAN_POINT('Ctrl Pts',(1.29596850710509,-1.,-1.51305994241402));
#25155=CARTESIAN_POINT('Ctrl Pts',(1.29373841372842,-1.,-1.50741159078365));
#25156=CARTESIAN_POINT('Ctrl Pts',(1.29145022885181,-1.,-1.50178230149776));
#25157=CARTESIAN_POINT('Ctrl Pts',(1.28911506584254,-1.,-1.49618896881754));
#25158=CARTESIAN_POINT('Ctrl Pts',(1.2867467611644,-1.,-1.4906522831278));
#25159=CARTESIAN_POINT('Ctrl Pts',(1.28435533880201,-1.,-1.4851881711891));
#25160=CARTESIAN_POINT('Ctrl Pts',(1.28194158939517,-1.,-1.47980070347096));
#25161=CARTESIAN_POINT('Ctrl Pts',(1.2794891824849,-1.,-1.4744717526707));
#25162=CARTESIAN_POINT('Ctrl Pts',(1.27696414831089,-1.,-1.46916035917133));
#25163=CARTESIAN_POINT('Ctrl Pts',(1.27433119897822,-1.,-1.46382431332476));
#25164=CARTESIAN_POINT('Ctrl Pts',(1.27156805265289,-1.,-1.45843906294697));
#25165=CARTESIAN_POINT('Ctrl Pts',(1.2686778680489,-1.,-1.45301422764247));
#25166=CARTESIAN_POINT('Ctrl Pts',(1.26570925118868,-1.,-1.44761985001662));
#25167=CARTESIAN_POINT('Ctrl Pts',(1.26273903323858,-1.,-1.44236470511303));
#25168=CARTESIAN_POINT('Ctrl Pts',(1.25983531012005,-1.,-1.43734919180848));
#25169=CARTESIAN_POINT('Ctrl Pts',(1.25702687965755,-1.,-1.43262645609691));
#25170=CARTESIAN_POINT('Ctrl Pts',(1.25426945222639,-1.,-1.42815938799387));
#25171=CARTESIAN_POINT('Ctrl Pts',(1.2514145557001,-1.,-1.42378102115575));
#25172=CARTESIAN_POINT('Ctrl Pts',(1.24824430986571,-1.,-1.41923722596025));
#25173=CARTESIAN_POINT('Ctrl Pts',(1.24450600513056,-1.,-1.41422913175179));
#25174=CARTESIAN_POINT('Ctrl Pts',(1.23994455029534,-1.,-1.40845295531283));
#25175=CARTESIAN_POINT('Ctrl Pts',(1.23434087290423,-1.,-1.40164708206106));
#25176=CARTESIAN_POINT('Ctrl Pts',(1.22752961899387,-1.,-1.39361389568796));
#25177=CARTESIAN_POINT('Ctrl Pts',(1.21938737280852,-1.,-1.38420564527715));
#25178=CARTESIAN_POINT('Ctrl Pts',(1.20982812925645,-1.,-1.37331915607905));
#25179=CARTESIAN_POINT('Ctrl Pts',(1.1987959077932,-1.,-1.36088705043885));
#25180=CARTESIAN_POINT('Ctrl Pts',(1.18625865667441,-1.,-1.34687054001093));
#25181=CARTESIAN_POINT('Ctrl Pts',(1.17501305789857,-1.,-1.33437539347008));
#25182=CARTESIAN_POINT('Ctrl Pts',(1.16589330093588,-1.,-1.32428080721772));
#25183=CARTESIAN_POINT('Ctrl Pts',(1.15950888730809,-1.,-1.31722977216397));
#25184=CARTESIAN_POINT('Ctrl Pts',(1.15624053661742,-1.,-1.31362392696032));
#25185=CARTESIAN_POINT('',(1.31362392696032,-1.,-1.15624053661742));
#25186=CARTESIAN_POINT('Origin',(0.,-1.,0.));
#25187=CARTESIAN_POINT('',(1.73811241238545,-1.,-1.34869019493419));
#25188=CARTESIAN_POINT('Ctrl Pts',(1.31362392696032,-1.,-1.15624053661742));
#25189=CARTESIAN_POINT('Ctrl Pts',(1.3172297721596,-1.,-1.15950888730433));
#25190=CARTESIAN_POINT('Ctrl Pts',(1.32428080720544,-1.,-1.16589330092532));
#25191=CARTESIAN_POINT('Ctrl Pts',(1.33437539344842,-1.,-1.17501305787994));
#25192=CARTESIAN_POINT('Ctrl Pts',(1.34687053998157,-1.,-1.18625865664915));
#25193=CARTESIAN_POINT('Ctrl Pts',(1.36088705040677,-1.,-1.1987959077656));
#25194=CARTESIAN_POINT('Ctrl Pts',(1.37331915604962,-1.,-1.20982812923113));
#25195=CARTESIAN_POINT('Ctrl Pts',(1.38420564525391,-1.,-1.21938737278853));
#25196=CARTESIAN_POINT('Ctrl Pts',(1.39361389567257,-1.,-1.22752961898063));
#25197=CARTESIAN_POINT('Ctrl Pts',(1.40164708205345,-1.,-1.23434087289768));
#25198=CARTESIAN_POINT('Ctrl Pts',(1.40845295531151,-1.,-1.23994455029421));
#25199=CARTESIAN_POINT('Ctrl Pts',(1.41422913175437,-1.,-1.24450600513278));
#25200=CARTESIAN_POINT('Ctrl Pts',(1.41923722596421,-1.,-1.24824430986911));
#25201=CARTESIAN_POINT('Ctrl Pts',(1.42378102115911,-1.,-1.25141455570299));
#25202=CARTESIAN_POINT('Ctrl Pts',(1.42815938799555,-1.,-1.25426945222783));
#25203=CARTESIAN_POINT('Ctrl Pts',(1.43262645609679,-1.,-1.25702687965744));
#25204=CARTESIAN_POINT('Ctrl Pts',(1.43734919180719,-1.,-1.25983531011894));
#25205=CARTESIAN_POINT('Ctrl Pts',(1.44236470511145,-1.,-1.26273903323723));
#25206=CARTESIAN_POINT('Ctrl Pts',(1.44761985001544,-1.,-1.26570925118767));
#25207=CARTESIAN_POINT('Ctrl Pts',(1.45301422764205,-1.,-1.26867786804854));
#25208=CARTESIAN_POINT('Ctrl Pts',(1.45843906294725,-1.,-1.27156805265312));
#25209=CARTESIAN_POINT('Ctrl Pts',(1.4638243133254,-1.,-1.27433119897877));
#25210=CARTESIAN_POINT('Ctrl Pts',(1.46916035917197,-1.,-1.27696414831144));
#25211=CARTESIAN_POINT('Ctrl Pts',(1.4744717526711,-1.,-1.27948918248524));
#25212=CARTESIAN_POINT('Ctrl Pts',(1.47980070347102,-1.,-1.28194158939522));
#25213=CARTESIAN_POINT('Ctrl Pts',(1.48518817118891,-1.,-1.28435533880184));
#25214=CARTESIAN_POINT('Ctrl Pts',(1.4906522831275,-1.,-1.28674676116415));
#25215=CARTESIAN_POINT('Ctrl Pts',(1.49618896881729,-1.,-1.28911506584232));
#25216=CARTESIAN_POINT('Ctrl Pts',(1.50178230149764,-1.,-1.29145022885171));
#25217=CARTESIAN_POINT('Ctrl Pts',(1.50741159078367,-1.,-1.29373841372843));
#25218=CARTESIAN_POINT('Ctrl Pts',(1.51305994241412,-1.,-1.29596850710518));
#25219=CARTESIAN_POINT('Ctrl Pts',(1.51872184912735,-1.,-1.29813791800757));
#25220=CARTESIAN_POINT('Ctrl Pts',(1.5243995786107,-1.,-1.30024984366334));
#25221=CARTESIAN_POINT('Ctrl Pts',(1.53009970283893,-1.,-1.3023106439557));
#25222=CARTESIAN_POINT('Ctrl Pts',(1.53582981268976,-1.,-1.30432735639487));
#25223=CARTESIAN_POINT('Ctrl Pts',(1.54159462645428,-1.,-1.30630475189553));
#25224=CARTESIAN_POINT('Ctrl Pts',(1.54739413957183,-1.,-1.30824393907471));
#25225=CARTESIAN_POINT('Ctrl Pts',(1.55322568759481,-1.,-1.31014393684221));
#25226=CARTESIAN_POINT('Ctrl Pts',(1.55908521254822,-1.,-1.31200264341696));
#25227=CARTESIAN_POINT('Ctrl Pts',(1.56496872402352,-1.,-1.31381795281002));
#25228=CARTESIAN_POINT('Ctrl Pts',(1.57087397835721,-1.,-1.31558903860015));
#25229=CARTESIAN_POINT('Ctrl Pts',(1.57680056505585,-1.,-1.31731642317183));
#25230=CARTESIAN_POINT('Ctrl Pts',(1.58274907898829,-1.,-1.31900135021428));
#25231=CARTESIAN_POINT('Ctrl Pts',(1.58872057258244,-1.,-1.32064537110891));
#25232=CARTESIAN_POINT('Ctrl Pts',(1.59471591079408,-1.,-1.32224985747686));
#25233=CARTESIAN_POINT('Ctrl Pts',(1.600735118587,-1.,-1.32381550858266));
#25234=CARTESIAN_POINT('Ctrl Pts',(1.6067775829097,-1.,-1.32534250785794));
#25235=CARTESIAN_POINT('Ctrl Pts',(1.61284234015762,-1.,-1.32683074483365));
#25236=CARTESIAN_POINT('Ctrl Pts',(1.61892832270723,-1.,-1.32828000610448));
#25237=CARTESIAN_POINT('Ctrl Pts',(1.62503464209777,-1.,-1.32969019505665));
#25238=CARTESIAN_POINT('Ctrl Pts',(1.63116079730887,-1.,-1.33106149345618));
#25239=CARTESIAN_POINT('Ctrl Pts',(1.63730653475049,-1.,-1.33239425103694));
#25240=CARTESIAN_POINT('Ctrl Pts',(1.64347174856007,-1.,-1.33368890676554));
#25241=CARTESIAN_POINT('Ctrl Pts',(1.64965637286843,-1.,-1.33494590468003));
#25242=CARTESIAN_POINT('Ctrl Pts',(1.65586025952651,-1.,-1.33616559745217));
#25243=CARTESIAN_POINT('Ctrl Pts',(1.66208312542073,-1.,-1.33734820885331));
#25244=CARTESIAN_POINT('Ctrl Pts',(1.66832460784078,-1.,-1.33849388654458));
#25245=CARTESIAN_POINT('Ctrl Pts',(1.67458429426126,-1.,-1.33960273470372));
#25246=CARTESIAN_POINT('Ctrl Pts',(1.68086176030308,-1.,-1.3406748518516));
#25247=CARTESIAN_POINT('Ctrl Pts',(1.68715660868602,-1.,-1.34171037484673));
#25248=CARTESIAN_POINT('Ctrl Pts',(1.6934684849664,-1.,-1.34270948206139));
#25249=CARTESIAN_POINT('Ctrl Pts',(1.69979707754221,-1.,-1.34367237124322));
#25250=CARTESIAN_POINT('Ctrl Pts',(1.70614212266676,-1.,-1.34459924533783));
#25251=CARTESIAN_POINT('Ctrl Pts',(1.71250340687011,-1.,-1.34549029589563));
#25252=CARTESIAN_POINT('Ctrl Pts',(1.7188807715095,-1.,-1.34634568653586));
#25253=CARTESIAN_POINT('Ctrl Pts',(1.72527410681298,-1.,-1.34716554820013));
#25254=CARTESIAN_POINT('Ctrl Pts',(1.73040149654497,-1.,-1.3477930915247));
#25255=CARTESIAN_POINT('Ctrl Pts',(1.73425417886254,-1.,-1.34824783113158));
#25256=CARTESIAN_POINT('Ctrl Pts',(1.73682580585819,-1.,-1.34854391898145));
#25257=CARTESIAN_POINT('Ctrl Pts',(1.73811241238545,-1.,-1.34869019493419));
#25258=CARTESIAN_POINT('',(1.81978687191668,-1.,-1.23627494547115));
#25259=CARTESIAN_POINT('',(1.73811241238545,-1.,-1.34869019493419));
#25260=CARTESIAN_POINT('',(1.5055822144029,-1.,-0.892032620296855));
#25261=CARTESIAN_POINT('Ctrl Pts',(1.81978687191668,-1.,-1.23627494547115));
#25262=CARTESIAN_POINT('Ctrl Pts',(1.81925017193531,-1.,-1.23509651170384));
#25263=CARTESIAN_POINT('Ctrl Pts',(1.81817389920914,-1.,-1.23274224526804));
#25264=CARTESIAN_POINT('Ctrl Pts',(1.81655087183054,-1.,-1.22921864890975));
#25265=CARTESIAN_POINT('Ctrl Pts',(1.81436959209778,-1.,-1.22453613304507));
#25266=CARTESIAN_POINT('Ctrl Pts',(1.81161420806172,-1.,-1.2187090610323));
#25267=CARTESIAN_POINT('Ctrl Pts',(1.80882996916931,-1.,-1.2129081570818));
#25268=CARTESIAN_POINT('Ctrl Pts',(1.80601678480772,-1.,-1.20713356605519));
#25269=CARTESIAN_POINT('Ctrl Pts',(1.8031745483882,-1.,-1.2013854893912));
#25270=CARTESIAN_POINT('Ctrl Pts',(1.80030314370121,-1.,-1.19566418930405));
#25271=CARTESIAN_POINT('Ctrl Pts',(1.79740245923649,-1.,-1.1899699793456));
#25272=CARTESIAN_POINT('Ctrl Pts',(1.79447240321572,-1.,-1.18430321697471));
#25273=CARTESIAN_POINT('Ctrl Pts',(1.79151291552646,-1.,-1.17866429440781));
#25274=CARTESIAN_POINT('Ctrl Pts',(1.78852398877523,-1.,-1.17305363177265));
#25275=CARTESIAN_POINT('Ctrl Pts',(1.78550566040349,-1.,-1.16747166312239));
#25276=CARTESIAN_POINT('Ctrl Pts',(1.78245795880949,-1.,-1.16191881298458));
#25277=CARTESIAN_POINT('Ctrl Pts',(1.77938085564261,-1.,-1.15639547194689));
#25278=CARTESIAN_POINT('Ctrl Pts',(1.77627422557034,-1.,-1.15090197841531));
#25279=CARTESIAN_POINT('Ctrl Pts',(1.77313777896234,-1.,-1.14543858226948));
#25280=CARTESIAN_POINT('Ctrl Pts',(1.76997111386806,-1.,-1.14000548337));
#25281=CARTESIAN_POINT('Ctrl Pts',(1.76677384551883,-1.,-1.13460291804635));
#25282=CARTESIAN_POINT('Ctrl Pts',(1.76354571966171,-1.,-1.12923123555076));
#25283=CARTESIAN_POINT('Ctrl Pts',(1.76028671825084,-1.,-1.12389096855078));
#25284=CARTESIAN_POINT('Ctrl Pts',(1.75699720772089,-1.,-1.11858293216752));
#25285=CARTESIAN_POINT('Ctrl Pts',(1.75367772094617,-1.,-1.11330807582542));
#25286=CARTESIAN_POINT('Ctrl Pts',(1.75032866075914,-1.,-1.10806728183003));
#25287=CARTESIAN_POINT('Ctrl Pts',(1.74695004214924,-1.,-1.10286118991144));
#25288=CARTESIAN_POINT('Ctrl Pts',(1.74354119236212,-1.,-1.09768999241229));
#25289=CARTESIAN_POINT('Ctrl Pts',(1.74010053962252,-1.,-1.09255329056496));
#25290=CARTESIAN_POINT('Ctrl Pts',(1.73662628326093,-1.,-1.08745056285429));
#25291=CARTESIAN_POINT('Ctrl Pts',(1.73311705663407,-1.,-1.08238162784749));
#25292=CARTESIAN_POINT('Ctrl Pts',(1.72957248977424,-1.,-1.0773470373727));
#25293=CARTESIAN_POINT('Ctrl Pts',(1.72599406198489,-1.,-1.07234866990252));
#25294=CARTESIAN_POINT('Ctrl Pts',(1.72238500928456,-1.,-1.06738966975463));
#25295=CARTESIAN_POINT('Ctrl Pts',(1.71874858456908,-1.,-1.0624732468065));
#25296=CARTESIAN_POINT('Ctrl Pts',(1.71508654427022,-1.,-1.05760163192481));
#25297=CARTESIAN_POINT('Ctrl Pts',(1.71139783543986,-1.,-1.05277517202854));
#25298=CARTESIAN_POINT('Ctrl Pts',(1.70767646263641,-1.,-1.0479908540499));
#25299=CARTESIAN_POINT('Ctrl Pts',(1.70391338707969,-1.,-1.04324363334546));
#25300=CARTESIAN_POINT('Ctrl Pts',(1.70010052930951,-1.,-1.03852922490782));
#25301=CARTESIAN_POINT('Ctrl Pts',(1.69623414782769,-1.,-1.03384646003587));
#25302=CARTESIAN_POINT('Ctrl Pts',(1.69231840863471,-1.,-1.02919977579155));
#25303=CARTESIAN_POINT('Ctrl Pts',(1.68836910178475,-1.,-1.02460180535272));
#25304=CARTESIAN_POINT('Ctrl Pts',(1.68440578021739,-1.,-1.02006795074222));
#25305=CARTESIAN_POINT('Ctrl Pts',(1.6804428989482,-1.,-1.01561026162787));
#25306=CARTESIAN_POINT('Ctrl Pts',(1.67648246776457,-1.,-1.01123236493507));
#25307=CARTESIAN_POINT('Ctrl Pts',(1.67250335383248,-1.,-1.00692206696387));
#25308=CARTESIAN_POINT('Ctrl Pts',(1.66846059277231,-1.,-1.00265091003682));
#25309=CARTESIAN_POINT('Ctrl Pts',(1.66430758030304,-1.,-0.998389654952317));
#25310=CARTESIAN_POINT('Ctrl Pts',(1.66001553809916,-1.,-0.994121836661116));
#25311=CARTESIAN_POINT('Ctrl Pts',(1.65559044289746,-1.,-0.98985562785445));
#25312=CARTESIAN_POINT('Ctrl Pts',(1.6511001661277,-1.,-0.985642622921626));
#25313=CARTESIAN_POINT('Ctrl Pts',(1.64665139190834,-1.,-0.981562530940574));
#25314=CARTESIAN_POINT('Ctrl Pts',(1.64233990826831,-1.,-0.977689794120297));
#25315=CARTESIAN_POINT('Ctrl Pts',(1.63820952658157,-1.,-0.974066058287501));
#25316=CARTESIAN_POINT('Ctrl Pts',(1.63420665729609,-1.,-0.970669715996356));
#25317=CARTESIAN_POINT('Ctrl Pts',(1.63013849959083,-1.,-0.967387853228041));
#25318=CARTESIAN_POINT('Ctrl Pts',(1.6257193066974,-1.,-0.964046107037821));
#25319=CARTESIAN_POINT('Ctrl Pts',(1.62061638139929,-1.,-0.960438326099958));
#25320=CARTESIAN_POINT('Ctrl Pts',(1.61449324337233,-1.,-0.956354422921573));
#25321=CARTESIAN_POINT('Ctrl Pts',(1.60706069897794,-1.,-0.951613284361248));
#25322=CARTESIAN_POINT('Ctrl Pts',(1.59810042045408,-1.,-0.946078063325796));
#25323=CARTESIAN_POINT('Ctrl Pts',(1.58744937489796,-1.,-0.939646377909319));
#25324=CARTESIAN_POINT('Ctrl Pts',(1.57499388385561,-1.,-0.932246680128849));
#25325=CARTESIAN_POINT('Ctrl Pts',(1.56065988582509,-1.,-0.923832188966322));
#25326=CARTESIAN_POINT('Ctrl Pts',(1.54440491152807,-1.,-0.91437591904658));
#25327=CARTESIAN_POINT('Ctrl Pts',(1.52984849890434,-1.,-0.905967409640499));
#25328=CARTESIAN_POINT('Ctrl Pts',(1.51805569591479,-1.,-0.89918504749193));
#25329=CARTESIAN_POINT('Ctrl Pts',(1.50980486807181,-1.,-0.894452006967538));
#25330=CARTESIAN_POINT('Ctrl Pts',(1.5055822144029,-1.,-0.892032620296855));
#25331=CARTESIAN_POINT('',(1.60662857109684,-1.,-0.693717979106306));
#25332=CARTESIAN_POINT('Origin',(0.,-1.,0.));
#25333=CARTESIAN_POINT('',(2.0698113262342,-1.,-0.745574324794401));
#25334=CARTESIAN_POINT('Ctrl Pts',(1.60662857109684,-1.,-0.693717979106306));
#25335=CARTESIAN_POINT('Ctrl Pts',(1.61106790957619,-1.,-0.69571209787897));
#25336=CARTESIAN_POINT('Ctrl Pts',(1.61974673471117,-1.,-0.699605146398837));
#25337=CARTESIAN_POINT('Ctrl Pts',(1.6321654166204,-1.,-0.705159151977294));
#25338=CARTESIAN_POINT('Ctrl Pts',(1.64752408828442,-1.,-0.711993139340448));
#25339=CARTESIAN_POINT('Ctrl Pts',(1.66472880551777,-1.,-0.71958543378795));
#25340=CARTESIAN_POINT('Ctrl Pts',(1.67996158451922,-1.,-0.726235967982445));
#25341=CARTESIAN_POINT('Ctrl Pts',(1.69326921972915,-1.,-0.731963238685357));
#25342=CARTESIAN_POINT('Ctrl Pts',(1.70473309004249,-1.,-0.736799665716932));
#25343=CARTESIAN_POINT('Ctrl Pts',(1.71447789751001,-1.,-0.74079516202821));
#25344=CARTESIAN_POINT('Ctrl Pts',(1.72268229916769,-1.,-0.744021445433094));
#25345=CARTESIAN_POINT('Ctrl Pts',(1.72958533647714,-1.,-0.746574710097752));
#25346=CARTESIAN_POINT('Ctrl Pts',(1.7355035168033,-1.,-0.74858246295687));
#25347=CARTESIAN_POINT('Ctrl Pts',(1.74080458267114,-1.,-0.75019343598125));
#25348=CARTESIAN_POINT('Ctrl Pts',(1.74585086852502,-1.,-0.751555614164483));
#25349=CARTESIAN_POINT('Ctrl Pts',(1.75095139468794,-1.,-0.752797683531314));
#25350=CARTESIAN_POINT('Ctrl Pts',(1.75631083600019,-1.,-0.754009254027829));
#25351=CARTESIAN_POINT('Ctrl Pts',(1.76197817240128,-1.,-0.755220979974462));
#25352=CARTESIAN_POINT('Ctrl Pts',(1.76789396002998,-1.,-0.75642189602781));
#25353=CARTESIAN_POINT('Ctrl Pts',(1.77394167108292,-1.,-0.757578264077029));
#25354=CARTESIAN_POINT('Ctrl Pts',(1.77999411220945,-1.,-0.758650626677519));
#25355=CARTESIAN_POINT('Ctrl Pts',(1.78596964884604,-1.,-0.75961440111019));
#25356=CARTESIAN_POINT('Ctrl Pts',(1.7918581561088,-1.,-0.760469555880749));
#25357=CARTESIAN_POINT('Ctrl Pts',(1.79768986997783,-1.,-0.761229695230558));
#25358=CARTESIAN_POINT('Ctrl Pts',(1.80351583877342,-1.,-0.761915336443547));
#25359=CARTESIAN_POINT('Ctrl Pts',(1.80938551463965,-1.,-0.762546129463938));
#25360=CARTESIAN_POINT('Ctrl Pts',(1.8153211840553,-1.,-0.763132003836634));
#25361=CARTESIAN_POINT('Ctrl Pts',(1.82131873145266,-1.,-0.763673465462727));
#25362=CARTESIAN_POINT('Ctrl Pts',(1.82735991200065,-1.,-0.764165902605995));
#25363=CARTESIAN_POINT('Ctrl Pts',(1.83342077227142,-1.,-0.764602549687853));
#25364=CARTESIAN_POINT('Ctrl Pts',(1.83948181064835,-1.,-0.764978057881738));
#25365=CARTESIAN_POINT('Ctrl Pts',(1.84553698875924,-1.,-0.765291664862029));
#25366=CARTESIAN_POINT('Ctrl Pts',(1.85158945130063,-1.,-0.765545710619063));
#25367=CARTESIAN_POINT('Ctrl Pts',(1.85764741390394,-1.,-0.765744212909319));
#25368=CARTESIAN_POINT('Ctrl Pts',(1.86372027063312,-1.,-0.765891519092547));
#25369=CARTESIAN_POINT('Ctrl Pts',(1.86981398314341,-1.,-0.765990708546091));
#25370=CARTESIAN_POINT('Ctrl Pts',(1.87592888967883,-1.,-0.766042837036744));
#25371=CARTESIAN_POINT('Ctrl Pts',(1.88206215302561,-1.,-0.766047794851865));
#25372=CARTESIAN_POINT('Ctrl Pts',(1.88820926433409,-1.,-0.766004837062091));
#25373=CARTESIAN_POINT('Ctrl Pts',(1.89436577771388,-1.,-0.765913193856978));
#25374=CARTESIAN_POINT('Ctrl Pts',(1.90052930393596,-1.,-0.765772772593386));
#25375=CARTESIAN_POINT('Ctrl Pts',(1.90669961402356,-1.,-0.765584196937919));
#25376=CARTESIAN_POINT('Ctrl Pts',(1.91287765805169,-1.,-0.765348465884722));
#25377=CARTESIAN_POINT('Ctrl Pts',(1.91906491634196,-1.,-0.765066729667089));
#25378=CARTESIAN_POINT('Ctrl Pts',(1.92526263537048,-1.,-0.764740025488212));
#25379=CARTESIAN_POINT('Ctrl Pts',(1.93147105496382,-1.,-0.764369010673941));
#25380=CARTESIAN_POINT('Ctrl Pts',(1.93768964875886,-1.,-0.763954049121459));
#25381=CARTESIAN_POINT('Ctrl Pts',(1.9439174661764,-1.,-0.763495333538629));
#25382=CARTESIAN_POINT('Ctrl Pts',(1.95015342590024,-1.,-0.762992990878769));
#25383=CARTESIAN_POINT('Ctrl Pts',(1.95639665309869,-1.,-0.762447203806179));
#25384=CARTESIAN_POINT('Ctrl Pts',(1.96264672744186,-1.,-0.761858300014424));
#25385=CARTESIAN_POINT('Ctrl Pts',(1.96890351582499,-1.,-0.761226690483821));
#25386=CARTESIAN_POINT('Ctrl Pts',(1.97516705321494,-1.,-0.760552825409757));
#25387=CARTESIAN_POINT('Ctrl Pts',(1.98143741418172,-1.,-0.75983714745219));
#25388=CARTESIAN_POINT('Ctrl Pts',(1.98771456680874,-1.,-0.759080037802488));
#25389=CARTESIAN_POINT('Ctrl Pts',(1.99399831098817,-1.,-0.758281796766761));
#25390=CARTESIAN_POINT('Ctrl Pts',(2.00028834739178,-1.,-0.757442676862724));
#25391=CARTESIAN_POINT('Ctrl Pts',(2.0065843158773,-1.,-0.756562904646671));
#25392=CARTESIAN_POINT('Ctrl Pts',(2.01288584328084,-1.,-0.755642704957865));
#25393=CARTESIAN_POINT('Ctrl Pts',(2.01919259405809,-1.,-0.754682330722816));
#25394=CARTESIAN_POINT('Ctrl Pts',(2.02550428623313,-1.,-0.753682061112768));
#25395=CARTESIAN_POINT('Ctrl Pts',(2.03182068456221,-1.,-0.752642180487211));
#25396=CARTESIAN_POINT('Ctrl Pts',(2.03814160092099,-1.,-0.751562963361115));
#25397=CARTESIAN_POINT('Ctrl Pts',(2.04446689147979,-1.,-0.750444657875576));
#25398=CARTESIAN_POINT('Ctrl Pts',(2.05079645592154,-1.,-0.749287468665046));
#25399=CARTESIAN_POINT('Ctrl Pts',(2.05713023031006,-1.,-0.748091554183803));
#25400=CARTESIAN_POINT('Ctrl Pts',(2.06220058927826,-1.,-0.74710393278792));
#25401=CARTESIAN_POINT('Ctrl Pts',(2.06600523016815,-1.,-0.746345871544201));
#25402=CARTESIAN_POINT('Ctrl Pts',(2.06854248895728,-1.,-0.745832791378367));
#25403=CARTESIAN_POINT('Ctrl Pts',(2.0698113262342,-1.,-0.745574324794401));
#25404=CARTESIAN_POINT('',(2.11275013067528,-1.,-0.61342227326009));
#25405=CARTESIAN_POINT('',(2.0698113262342,-1.,-0.745574324794401));
#25406=CARTESIAN_POINT('',(1.7075470150345,-1.,-0.383122945602004));
#25407=CARTESIAN_POINT('Ctrl Pts',(2.11275013067528,-1.,-0.61342227326009));
#25408=CARTESIAN_POINT('Ctrl Pts',(2.11187554259986,-1.,-0.6124673655618));
#25409=CARTESIAN_POINT('Ctrl Pts',(2.11012443807238,-1.,-0.610560911689899));
#25410=CARTESIAN_POINT('Ctrl Pts',(2.1074919961518,-1.,-0.607711315454876));
#25411=CARTESIAN_POINT('Ctrl Pts',(2.10397049886949,-1.,-0.60393203073603));
#25412=CARTESIAN_POINT('Ctrl Pts',(2.0995493086477,-1.,-0.599241616420534));
#25413=CARTESIAN_POINT('Ctrl Pts',(2.0951087622027,-1.,-0.594585006052162));
#25414=CARTESIAN_POINT('Ctrl Pts',(2.09064881812129,-1.,-0.589962365403406));
#25415=CARTESIAN_POINT('Ctrl Pts',(2.08616943727951,-1.,-0.585373918991617));
#25416=CARTESIAN_POINT('Ctrl Pts',(2.08167059018418,-1.,-0.580819952108064));
#25417=CARTESIAN_POINT('Ctrl Pts',(2.07715226767559,-1.,-0.576300797416845));
#25418=CARTESIAN_POINT('Ctrl Pts',(2.07261449292824,-1.,-0.571816823242603));
#25419=CARTESIAN_POINT('Ctrl Pts',(2.06805732997334,-1.,-0.567368421181087));
#25420=CARTESIAN_POINT('Ctrl Pts',(2.06348090160589,-1.,-0.562955993082262));
#25421=CARTESIAN_POINT('Ctrl Pts',(2.05888537756462,-1.,-0.558579940185152));
#25422=CARTESIAN_POINT('Ctrl Pts',(2.05427091604413,-1.,-0.554240657463906));
#25423=CARTESIAN_POINT('Ctrl Pts',(2.04963761077958,-1.,-0.549938525150295));
#25424=CARTESIAN_POINT('Ctrl Pts',(2.04498544714588,-1.,-0.54567390381743));
#25425=CARTESIAN_POINT('Ctrl Pts',(2.04031422690527,-1.,-0.541447120615659));
#25426=CARTESIAN_POINT('Ctrl Pts',(2.03562362954037,-1.,-0.537258489833262));
#25427=CARTESIAN_POINT('Ctrl Pts',(2.03091336214426,-1.,-0.533108355132977));
#25428=CARTESIAN_POINT('Ctrl Pts',(2.0261832908329,-1.,-0.528997127241914));
#25429=CARTESIAN_POINT('Ctrl Pts',(2.02143356304698,-1.,-0.524925318333476));
#25430=CARTESIAN_POINT('Ctrl Pts',(2.01666477917286,-1.,-0.520893590399371));
#25431=CARTESIAN_POINT('Ctrl Pts',(2.01187773939242,-1.,-0.516902681728687));
#25432=CARTESIAN_POINT('Ctrl Pts',(2.00707309946949,-1.,-0.512953306961793));
#25433=CARTESIAN_POINT('Ctrl Pts',(2.00225107134734,-1.,-0.509046069886157));
#25434=CARTESIAN_POINT('Ctrl Pts',(1.99741107463572,-1.,-0.505181361323026));
#25435=CARTESIAN_POINT('Ctrl Pts',(1.99255149126155,-1.,-0.501359287727146));
#25436=CARTESIAN_POINT('Ctrl Pts',(1.98767044752932,-1.,-0.497579909545574));
#25437=CARTESIAN_POINT('Ctrl Pts',(1.98276658761821,-1.,-0.493843476541495));
#25438=CARTESIAN_POINT('Ctrl Pts',(1.97783973019229,-1.,-0.490150627860953));
#25439=CARTESIAN_POINT('Ctrl Pts',(1.97289186263272,-1.,-0.486502692907659));
#25440=CARTESIAN_POINT('Ctrl Pts',(1.96792703422362,-1.,-0.482901662120691));
#25441=CARTESIAN_POINT('Ctrl Pts',(1.96294933055943,-1.,-0.479349583074855));
#25442=CARTESIAN_POINT('Ctrl Pts',(1.95796111148177,-1.,-0.475848034683176));
#25443=CARTESIAN_POINT('Ctrl Pts',(1.95296148278133,-1.,-0.472397672264072));
#25444=CARTESIAN_POINT('Ctrl Pts',(1.94794381136514,-1.,-0.468997482913135));
#25445=CARTESIAN_POINT('Ctrl Pts',(1.9428979419619,-1.,-0.46564546202603));
#25446=CARTESIAN_POINT('Ctrl Pts',(1.93781486640821,-1.,-0.462340031009057));
#25447=CARTESIAN_POINT('Ctrl Pts',(1.93269066517934,-1.,-0.459081234547926));
#25448=CARTESIAN_POINT('Ctrl Pts',(1.92753067150476,-1.,-0.455872005174371));
#25449=CARTESIAN_POINT('Ctrl Pts',(1.92235380648502,-1.,-0.452719478359433));
#25450=CARTESIAN_POINT('Ctrl Pts',(1.91718342555755,-1.,-0.449632260106662));
#25451=CARTESIAN_POINT('Ctrl Pts',(1.9120369998112,-1.,-0.446617343485711));
#25452=CARTESIAN_POINT('Ctrl Pts',(1.90691756144898,-1.,-0.443677556849151));
#25453=CARTESIAN_POINT('Ctrl Pts',(1.90180124389086,-1.,-0.440807833704038));
#25454=CARTESIAN_POINT('Ctrl Pts',(1.89663648956466,-1.,-0.437995003948244));
#25455=CARTESIAN_POINT('Ctrl Pts',(1.89136993975504,-1.,-0.435225660963383));
#25456=CARTESIAN_POINT('Ctrl Pts',(1.88596913666793,-1.,-0.432493038548748));
#25457=CARTESIAN_POINT('Ctrl Pts',(1.88044229001832,-1.,-0.429803062482345));
#25458=CARTESIAN_POINT('Ctrl Pts',(1.87486989291484,-1.,-0.427183828519102));
#25459=CARTESIAN_POINT('Ctrl Pts',(1.86937803944323,-1.,-0.424678177291359));
#25460=CARTESIAN_POINT('Ctrl Pts',(1.86408083334028,-1.,-0.422327307418275));
#25461=CARTESIAN_POINT('Ctrl Pts',(1.85903281096686,-1.,-0.42015728797562));
#25462=CARTESIAN_POINT('Ctrl Pts',(1.85417632856234,-1.,-0.418164129143534));
#25463=CARTESIAN_POINT('Ctrl Pts',(1.84929312929882,-1.,-0.416300022038864));
#25464=CARTESIAN_POINT('Ctrl Pts',(1.8440575707371,-1.,-0.41448743825434));
#25465=CARTESIAN_POINT('Ctrl Pts',(1.83808953475839,-1.,-0.412633125322162));
#25466=CARTESIAN_POINT('Ctrl Pts',(1.83100408895216,-1.,-0.410641256301675));
#25467=CARTESIAN_POINT('Ctrl Pts',(1.8224702267854,-1.,-0.408428948108534));
#25468=CARTESIAN_POINT('Ctrl Pts',(1.81223801813988,-1.,-0.405933518411838));
#25469=CARTESIAN_POINT('Ctrl Pts',(1.80012077176221,-1.,-0.403107976170441));
#25470=CARTESIAN_POINT('Ctrl Pts',(1.78598826347533,-1.,-0.399919403783081));
#25471=CARTESIAN_POINT('Ctrl Pts',(1.7697556004756,-1.,-0.39634619612042));
#25472=CARTESIAN_POINT('Ctrl Pts',(1.75137405313962,-1.,-0.392375812294307));
#25473=CARTESIAN_POINT('Ctrl Pts',(1.7349317097561,-1.,-0.388877023509192));
#25474=CARTESIAN_POINT('Ctrl Pts',(1.72162022246158,-1.,-0.38607079032701));
#25475=CARTESIAN_POINT('Ctrl Pts',(1.71231062891958,-1.,-0.384119047315542));
#25476=CARTESIAN_POINT('Ctrl Pts',(1.7075470150345,-1.,-0.383122945602004));
#25477=CARTESIAN_POINT('',(1.74236521665491,-1.,-0.163289472382896));
#25478=CARTESIAN_POINT('Origin',(0.,-1.,0.));
#25479=CARTESIAN_POINT('',(2.19890268624765,-1.,-0.0694764450219582));
#25480=CARTESIAN_POINT('Ctrl Pts',(1.74236521665491,-1.,-0.163289472382896));
#25481=CARTESIAN_POINT('Ctrl Pts',(1.7472034950333,-1.,-0.163814161002002));
#25482=CARTESIAN_POINT('Ctrl Pts',(1.75666056638427,-1.,-0.164834765707159));
#25483=CARTESIAN_POINT('Ctrl Pts',(1.77018771684844,-1.,-0.1662793551464));
#25484=CARTESIAN_POINT('Ctrl Pts',(1.7869064998507,-1.,-0.168032772805197));
#25485=CARTESIAN_POINT('Ctrl Pts',(1.80561530629706,-1.,-0.169936923904608));
#25486=CARTESIAN_POINT('Ctrl Pts',(1.82215766811545,-1.,-0.171554770204119));
#25487=CARTESIAN_POINT('Ctrl Pts',(1.83658380527692,-1.,-0.1728894428919));
#25488=CARTESIAN_POINT('Ctrl Pts',(1.8489811319852,-1.,-0.173946627587732));
#25489=CARTESIAN_POINT('Ctrl Pts',(1.85948367088837,-1.,-0.17473525927603));
#25490=CARTESIAN_POINT('Ctrl Pts',(1.86828349694799,-1.,-0.175268337590758));
#25491=CARTESIAN_POINT('Ctrl Pts',(1.87563767773588,-1.,-0.175563480746485));
#25492=CARTESIAN_POINT('Ctrl Pts',(1.88188663145367,-1.,-0.175644148889699));
#25493=CARTESIAN_POINT('Ctrl Pts',(1.88742606273259,-1.,-0.175538155840648));
#25494=CARTESIAN_POINT('Ctrl Pts',(1.892646301985,-1.,-0.175274276190844));
#25495=CARTESIAN_POINT('Ctrl Pts',(1.89788101117132,-1.,-0.174879405091263));
#25496=CARTESIAN_POINT('Ctrl Pts',(1.90335253862834,-1.,-0.174375518661085));
#25497=CARTESIAN_POINT('Ctrl Pts',(1.90911693975267,-1.,-0.173776635257817));
#25498=CARTESIAN_POINT('Ctrl Pts',(1.91511429159527,-1.,-0.173090695383496));
#25499=CARTESIAN_POINT('Ctrl Pts',(1.9212233439798,-1.,-0.172321621259514));
#25500=CARTESIAN_POINT('Ctrl Pts',(1.92731093582036,-1.,-0.171471191532988));
#25501=CARTESIAN_POINT('Ctrl Pts',(1.93329183155539,-1.,-0.170541253116202));
#25502=CARTESIAN_POINT('Ctrl Pts',(1.93915639211581,-1.,-0.169534904817491));
#25503=CARTESIAN_POINT('Ctrl Pts',(1.94493757756931,-1.,-0.168455741607556));
#25504=CARTESIAN_POINT('Ctrl Pts',(1.95069027794294,-1.,-0.167307501784476));
#25505=CARTESIAN_POINT('Ctrl Pts',(1.9564675971873,-1.,-0.166093592002813));
#25506=CARTESIAN_POINT('Ctrl Pts',(1.96229379940136,-1.,-0.164816568920269));
#25507=CARTESIAN_POINT('Ctrl Pts',(1.96816512677967,-1.,-0.163478185457734));
#25508=CARTESIAN_POINT('Ctrl Pts',(1.97406280235188,-1.,-0.162079693556289));
#25509=CARTESIAN_POINT('Ctrl Pts',(1.97996195437559,-1.,-0.160622060784611));
#25510=CARTESIAN_POINT('Ctrl Pts',(1.98584238283292,-1.,-0.159106226437299));
#25511=CARTESIAN_POINT('Ctrl Pts',(1.99169810931908,-1.,-0.157533331459227));
#25512=CARTESIAN_POINT('Ctrl Pts',(1.99753284771497,-1.,-0.155904629548784));
#25513=CARTESIAN_POINT('Ctrl Pts',(2.00335565310543,-1.,-0.154221403049722));
#25514=CARTESIAN_POINT('Ctrl Pts',(2.00917680318424,-1.,-0.15248488362145));
#25515=CARTESIAN_POINT('Ctrl Pts',(2.01500291940238,-1.,-0.150696157673078));
#25516=CARTESIAN_POINT('Ctrl Pts',(2.02083464969894,-1.,-0.148856124775337));
#25517=CARTESIAN_POINT('Ctrl Pts',(2.02666926182017,-1.,-0.146965557332583));
#25518=CARTESIAN_POINT('Ctrl Pts',(2.03250223739942,-1.,-0.145025140186058));
#25519=CARTESIAN_POINT('Ctrl Pts',(2.03832911025912,-1.,-0.143035515058209));
#25520=CARTESIAN_POINT('Ctrl Pts',(2.04414757947916,-1.,-0.140997332152546));
#25521=CARTESIAN_POINT('Ctrl Pts',(2.04995762001328,-1.,-0.138911255368966));
#25522=CARTESIAN_POINT('Ctrl Pts',(2.05576044414264,-1.,-0.136777941218044));
#25523=CARTESIAN_POINT('Ctrl Pts',(2.06155781517842,-1.,-0.134598026192106));
#25524=CARTESIAN_POINT('Ctrl Pts',(2.06735123910326,-1.,-0.132372111547711));
#25525=CARTESIAN_POINT('Ctrl Pts',(2.07314114713063,-1.,-0.130100748328404));
#25526=CARTESIAN_POINT('Ctrl Pts',(2.07892715110987,-1.,-0.12778444527612));
#25527=CARTESIAN_POINT('Ctrl Pts',(2.08470840653643,-1.,-0.125423679412062));
#25528=CARTESIAN_POINT('Ctrl Pts',(2.09048392424825,-1.,-0.123018905621083));
#25529=CARTESIAN_POINT('Ctrl Pts',(2.0962529286773,-1.,-0.120570567965122));
#25530=CARTESIAN_POINT('Ctrl Pts',(2.102015121329,-1.,-0.118079107988356));
#25531=CARTESIAN_POINT('Ctrl Pts',(2.10777050261309,-1.,-0.115544957687927));
#25532=CARTESIAN_POINT('Ctrl Pts',(2.11351924490306,-1.,-0.112968534419737));
#25533=CARTESIAN_POINT('Ctrl Pts',(2.11926155590865,-1.,-0.110350236135025));
#25534=CARTESIAN_POINT('Ctrl Pts',(2.12499752307,-1.,-0.10769043523109));
#25535=CARTESIAN_POINT('Ctrl Pts',(2.13072704887293,-1.,-0.10498947915274));
#25536=CARTESIAN_POINT('Ctrl Pts',(2.13644992667165,-1.,-0.102247700556101));
#25537=CARTESIAN_POINT('Ctrl Pts',(2.14216588396025,-1.,-0.0994654261990917));
#25538=CARTESIAN_POINT('Ctrl Pts',(2.14787463531795,-1.,-0.096642985230546));
#25539=CARTESIAN_POINT('Ctrl Pts',(2.1535759397817,-1.,-0.0937807218867645));
#25540=CARTESIAN_POINT('Ctrl Pts',(2.15926961544516,-1.,-0.0908789888107267));
#25541=CARTESIAN_POINT('Ctrl Pts',(2.16495552645014,-1.,-0.0879381291386924));
#25542=CARTESIAN_POINT('Ctrl Pts',(2.17063357870952,-1.,-0.0849584620835374));
#25543=CARTESIAN_POINT('Ctrl Pts',(2.176303712113,-1.,-0.0819402680872767));
#25544=CARTESIAN_POINT('Ctrl Pts',(2.18196589448887,-1.,-0.0788837727685244));
#25545=CARTESIAN_POINT('Ctrl Pts',(2.1876201139953,-1.,-0.0757891465836149));
#25546=CARTESIAN_POINT('Ctrl Pts',(2.19213712013662,-1.,-0.0732830357306726));
#25547=CARTESIAN_POINT('Ctrl Pts',(2.19552129484002,-1.,-0.0713863779526155));
#25548=CARTESIAN_POINT('Ctrl Pts',(2.19777582085423,-1.,-0.0701143536325491));
#25549=CARTESIAN_POINT('Ctrl Pts',(2.19890268624765,-1.,-0.0694764450219582));
#25550=CARTESIAN_POINT('',(2.19890268624765,-1.,0.0694764450219582));
#25551=CARTESIAN_POINT('',(2.19890268624765,-1.,-0.0694764450219582));
#25552=CARTESIAN_POINT('',(1.74236521665491,-1.,0.163289472382896));
#25553=CARTESIAN_POINT('Ctrl Pts',(2.19890268624765,-1.,0.0694764450219582));
#25554=CARTESIAN_POINT('Ctrl Pts',(2.19777582085261,-1.,0.0701143536324925));
#25555=CARTESIAN_POINT('Ctrl Pts',(2.19552129483562,-1.,0.0713863779524626));
#25556=CARTESIAN_POINT('Ctrl Pts',(2.19213712012956,-1.,0.0732830357304275));
#25557=CARTESIAN_POINT('Ctrl Pts',(2.1876201139874,-1.,0.075789146583341));
#25558=CARTESIAN_POINT('Ctrl Pts',(2.18196589448304,-1.,0.0788837727683226));
#25559=CARTESIAN_POINT('Ctrl Pts',(2.1763037121106,-1.,0.0819402680871938));
#25560=CARTESIAN_POINT('Ctrl Pts',(2.17063357871031,-1.,0.0849584620835642));
#25561=CARTESIAN_POINT('Ctrl Pts',(2.16495552645275,-1.,0.0879381291387821));
#25562=CARTESIAN_POINT('Ctrl Pts',(2.15926961544808,-1.,0.0908789888108265));
#25563=CARTESIAN_POINT('Ctrl Pts',(2.15357593978377,-1.,0.0937807218868344));
#25564=CARTESIAN_POINT('Ctrl Pts',(2.14787463531864,-1.,0.0966429852305688));
#25565=CARTESIAN_POINT('Ctrl Pts',(2.14216588395974,-1.,0.0994654261990741));
#25566=CARTESIAN_POINT('Ctrl Pts',(2.13644992667052,-1.,0.102247700556063));
#25567=CARTESIAN_POINT('Ctrl Pts',(2.1307270488718,-1.,0.104989479152703));
#25568=CARTESIAN_POINT('Ctrl Pts',(2.12499752306927,-1.,0.107690435231068));
#25569=CARTESIAN_POINT('Ctrl Pts',(2.11926155590849,-1.,0.11035023613502));
#25570=CARTESIAN_POINT('Ctrl Pts',(2.11351924490335,-1.,0.112968534419746));
#25571=CARTESIAN_POINT('Ctrl Pts',(2.10777050261359,-1.,0.11554495768794));
#25572=CARTESIAN_POINT('Ctrl Pts',(2.10201512132945,-1.,0.118079107988368));
#25573=CARTESIAN_POINT('Ctrl Pts',(2.09625292867756,-1.,0.120570567965129));
#25574=CARTESIAN_POINT('Ctrl Pts',(2.09048392424826,-1.,0.123018905621083));
#25575=CARTESIAN_POINT('Ctrl Pts',(2.08470840653628,-1.,0.125423679412058));
#25576=CARTESIAN_POINT('Ctrl Pts',(2.07892715110967,-1.,0.127784445276116));
#25577=CARTESIAN_POINT('Ctrl Pts',(2.07314114713047,-1.,0.1301007483284));
#25578=CARTESIAN_POINT('Ctrl Pts',(2.06735123910319,-1.,0.132372111547709));
#25579=CARTESIAN_POINT('Ctrl Pts',(2.06155781517844,-1.,0.134598026192107));
#25580=CARTESIAN_POINT('Ctrl Pts',(2.0557604441427,-1.,0.136777941218044));
#25581=CARTESIAN_POINT('Ctrl Pts',(2.04995762001333,-1.,0.138911255368966));
#25582=CARTESIAN_POINT('Ctrl Pts',(2.04414757947919,-1.,0.140997332152545));
#25583=CARTESIAN_POINT('Ctrl Pts',(2.03832911025913,-1.,0.143035515058208));
#25584=CARTESIAN_POINT('Ctrl Pts',(2.03250223739941,-1.,0.145025140186058));
#25585=CARTESIAN_POINT('Ctrl Pts',(2.02666926182017,-1.,0.146965557332586));
#25586=CARTESIAN_POINT('Ctrl Pts',(2.02083464969897,-1.,0.148856124775342));
#25587=CARTESIAN_POINT('Ctrl Pts',(2.01500291940243,-1.,0.150696157673084));
#25588=CARTESIAN_POINT('Ctrl Pts',(2.00917680318426,-1.,0.152484883621452));
#25589=CARTESIAN_POINT('Ctrl Pts',(2.00335565310539,-1.,0.154221403049719));
#25590=CARTESIAN_POINT('Ctrl Pts',(1.99753284771487,-1.,0.155904629548774));
#25591=CARTESIAN_POINT('Ctrl Pts',(1.99169810931893,-1.,0.157533331459215));
#25592=CARTESIAN_POINT('Ctrl Pts',(1.98584238283279,-1.,0.159106226437288));
#25593=CARTESIAN_POINT('Ctrl Pts',(1.97996195437557,-1.,0.16062206078461));
#25594=CARTESIAN_POINT('Ctrl Pts',(1.97406280235204,-1.,0.162079693556302));
#25595=CARTESIAN_POINT('Ctrl Pts',(1.96816512678,-1.,0.16347818545776));
#25596=CARTESIAN_POINT('Ctrl Pts',(1.96229379940174,-1.,0.1648165689203));
#25597=CARTESIAN_POINT('Ctrl Pts',(1.95646759718755,-1.,0.166093592002832));
#25598=CARTESIAN_POINT('Ctrl Pts',(1.95069027794286,-1.,0.167307501784469));
#25599=CARTESIAN_POINT('Ctrl Pts',(1.94493757756879,-1.,0.168455741607515));
#25600=CARTESIAN_POINT('Ctrl Pts',(1.93915639211497,-1.,0.169534904817425));
#25601=CARTESIAN_POINT('Ctrl Pts',(1.93329183155455,-1.,0.170541253116136));
#25602=CARTESIAN_POINT('Ctrl Pts',(1.92731093582,-1.,0.17147119153296));
#25603=CARTESIAN_POINT('Ctrl Pts',(1.92122334398034,-1.,0.172321621259556));
#25604=CARTESIAN_POINT('Ctrl Pts',(1.91511429159681,-1.,0.173090695383619));
#25605=CARTESIAN_POINT('Ctrl Pts',(1.90911693975475,-1.,0.173776635257983));
#25606=CARTESIAN_POINT('Ctrl Pts',(1.90335253863003,-1.,0.174375518661222));
#25607=CARTESIAN_POINT('Ctrl Pts',(1.89788101117148,-1.,0.174879405091277));
#25608=CARTESIAN_POINT('Ctrl Pts',(1.89264630198279,-1.,0.175274276190664));
#25609=CARTESIAN_POINT('Ctrl Pts',(1.88742606272818,-1.,0.175538155840286));
#25610=CARTESIAN_POINT('Ctrl Pts',(1.88188663144846,-1.,0.175644148889271));
#25611=CARTESIAN_POINT('Ctrl Pts',(1.87563767773249,-1.,0.175563480746205));
#25612=CARTESIAN_POINT('Ctrl Pts',(1.86828349694972,-1.,0.1752683375909));
#25613=CARTESIAN_POINT('Ctrl Pts',(1.85948367089838,-1.,0.174735259276856));
#25614=CARTESIAN_POINT('Ctrl Pts',(1.84898113200543,-1.,0.173946627589401));
#25615=CARTESIAN_POINT('Ctrl Pts',(1.83658380530747,-1.,0.17288944289442));
#25616=CARTESIAN_POINT('Ctrl Pts',(1.82215766815414,-1.,0.171554770207306));
#25617=CARTESIAN_POINT('Ctrl Pts',(1.80561530633924,-1.,0.169936923908078));
#25618=CARTESIAN_POINT('Ctrl Pts',(1.78690649988931,-1.,0.16803277280837));
#25619=CARTESIAN_POINT('Ctrl Pts',(1.77018771687692,-1.,0.166279355148738));
#25620=CARTESIAN_POINT('Ctrl Pts',(1.75666056640041,-1.,0.164834765708484));
#25621=CARTESIAN_POINT('Ctrl Pts',(1.74720349503904,-1.,0.163814161002474));
#25622=CARTESIAN_POINT('Ctrl Pts',(1.74236521665491,-1.,0.163289472382896));
#25623=CARTESIAN_POINT('',(1.7075470150345,-1.,0.383122945602004));
#25624=CARTESIAN_POINT('Origin',(0.,-1.,0.));
#25625=CARTESIAN_POINT('',(2.11275013067528,-1.,0.613422273260091));
#25626=CARTESIAN_POINT('Ctrl Pts',(1.7075470150345,-1.,0.383122945602004));
#25627=CARTESIAN_POINT('Ctrl Pts',(1.71231062891398,-1.,0.384119047314215));
#25628=CARTESIAN_POINT('Ctrl Pts',(1.72162022244582,-1.,0.386070790323281));
#25629=CARTESIAN_POINT('Ctrl Pts',(1.73493170972829,-1.,0.388877023502615));
#25630=CARTESIAN_POINT('Ctrl Pts',(1.75137405310193,-1.,0.392375812285396));
#25631=CARTESIAN_POINT('Ctrl Pts',(1.76975560043442,-1.,0.396346196110688));
#25632=CARTESIAN_POINT('Ctrl Pts',(1.78598826343754,-1.,0.399919403774156));
#25633=CARTESIAN_POINT('Ctrl Pts',(1.80012077173238,-1.,0.403107976163396));
#25634=CARTESIAN_POINT('Ctrl Pts',(1.81223801812013,-1.,0.405933518407176));
#25635=CARTESIAN_POINT('Ctrl Pts',(1.82247022677562,-1.,0.408428948106228));
#25636=CARTESIAN_POINT('Ctrl Pts',(1.83100408895047,-1.,0.410641256301276));
#25637=CARTESIAN_POINT('Ctrl Pts',(1.8380895347617,-1.,0.412633125322945));
#25638=CARTESIAN_POINT('Ctrl Pts',(1.84405757074218,-1.,0.414487438255542));
#25639=CARTESIAN_POINT('Ctrl Pts',(1.84929312930314,-1.,0.416300022039885));
#25640=CARTESIAN_POINT('Ctrl Pts',(1.8541763285645,-1.,0.418164129144046));
#25641=CARTESIAN_POINT('Ctrl Pts',(1.8590328109667,-1.,0.420157287975583));
#25642=CARTESIAN_POINT('Ctrl Pts',(1.86408083333863,-1.,0.422327307417885));
#25643=CARTESIAN_POINT('Ctrl Pts',(1.8693780394412,-1.,0.424678177290876));
#25644=CARTESIAN_POINT('Ctrl Pts',(1.87486989291333,-1.,0.427183828518743));
#25645=CARTESIAN_POINT('Ctrl Pts',(1.88044229001778,-1.,0.429803062482217));
#25646=CARTESIAN_POINT('Ctrl Pts',(1.88596913666828,-1.,0.432493038548833));
#25647=CARTESIAN_POINT('Ctrl Pts',(1.89136993975585,-1.,0.43522566096358));
#25648=CARTESIAN_POINT('Ctrl Pts',(1.89663648956549,-1.,0.437995003948443));
#25649=CARTESIAN_POINT('Ctrl Pts',(1.90180124389137,-1.,0.440807833704161));
#25650=CARTESIAN_POINT('Ctrl Pts',(1.90691756144906,-1.,0.443677556849171));
#25651=CARTESIAN_POINT('Ctrl Pts',(1.91203699981095,-1.,0.446617343485651));
#25652=CARTESIAN_POINT('Ctrl Pts',(1.91718342555717,-1.,0.449632260106572));
#25653=CARTESIAN_POINT('Ctrl Pts',(1.9223538064847,-1.,0.452719478359356));
#25654=CARTESIAN_POINT('Ctrl Pts',(1.92753067150461,-1.,0.455872005174336));
#25655=CARTESIAN_POINT('Ctrl Pts',(1.93269066517936,-1.,0.459081234547932));
#25656=CARTESIAN_POINT('Ctrl Pts',(1.93781486640834,-1.,0.462340031009087));
#25657=CARTESIAN_POINT('Ctrl Pts',(1.94289794196205,-1.,0.465645462026065));
#25658=CARTESIAN_POINT('Ctrl Pts',(1.94794381136524,-1.,0.468997482913158));
#25659=CARTESIAN_POINT('Ctrl Pts',(1.95296148278136,-1.,0.47239767226408));
#25660=CARTESIAN_POINT('Ctrl Pts',(1.95796111148175,-1.,0.475848034683172));
#25661=CARTESIAN_POINT('Ctrl Pts',(1.96294933055938,-1.,0.479349583074846));
#25662=CARTESIAN_POINT('Ctrl Pts',(1.96792703422358,-1.,0.482901662120687));
#25663=CARTESIAN_POINT('Ctrl Pts',(1.97289186263272,-1.,0.486502692907661));
#25664=CARTESIAN_POINT('Ctrl Pts',(1.97783973019229,-1.,0.490150627860955));
#25665=CARTESIAN_POINT('Ctrl Pts',(1.9827665876182,-1.,0.493843476541493));
#25666=CARTESIAN_POINT('Ctrl Pts',(1.98767044752929,-1.,0.497579909545564));
#25667=CARTESIAN_POINT('Ctrl Pts',(1.9925514912615,-1.,0.501359287727129));
#25668=CARTESIAN_POINT('Ctrl Pts',(1.99741107463567,-1.,0.505181361323011));
#25669=CARTESIAN_POINT('Ctrl Pts',(2.00225107134733,-1.,0.509046069886152));
#25670=CARTESIAN_POINT('Ctrl Pts',(2.00707309946955,-1.,0.512953306961814));
#25671=CARTESIAN_POINT('Ctrl Pts',(2.01187773939257,-1.,0.516902681728733));
#25672=CARTESIAN_POINT('Ctrl Pts',(2.01666477917305,-1.,0.520893590399429));
#25673=CARTESIAN_POINT('Ctrl Pts',(2.02143356304712,-1.,0.524925318333519));
#25674=CARTESIAN_POINT('Ctrl Pts',(2.02618329083289,-1.,0.528997127241911));
#25675=CARTESIAN_POINT('Ctrl Pts',(2.03091336214401,-1.,0.533108355132905));
#25676=CARTESIAN_POINT('Ctrl Pts',(2.03562362953993,-1.,0.537258489833135));
#25677=CARTESIAN_POINT('Ctrl Pts',(2.0403142269048,-1.,0.54144712061552));
#25678=CARTESIAN_POINT('Ctrl Pts',(2.0449854471456,-1.,0.545673903817349));
#25679=CARTESIAN_POINT('Ctrl Pts',(2.04963761077974,-1.,0.549938525150342));
#25680=CARTESIAN_POINT('Ctrl Pts',(2.05427091604482,-1.,0.55424065746411));
#25681=CARTESIAN_POINT('Ctrl Pts',(2.05888537756571,-1.,0.558579940185468));
#25682=CARTESIAN_POINT('Ctrl Pts',(2.06348090160697,-1.,0.562955993082574));
#25683=CARTESIAN_POINT('Ctrl Pts',(2.06805732997383,-1.,0.56736842118123));
#25684=CARTESIAN_POINT('Ctrl Pts',(2.07261449292757,-1.,0.571816823242411));
#25685=CARTESIAN_POINT('Ctrl Pts',(2.07715226767361,-1.,0.576300797416275));
#25686=CARTESIAN_POINT('Ctrl Pts',(2.08167059018138,-1.,0.580819952107257));
#25687=CARTESIAN_POINT('Ctrl Pts',(2.086169437277,-1.,0.585373918990895));
#25688=CARTESIAN_POINT('Ctrl Pts',(2.09064881812053,-1.,0.58996236540319));
#25689=CARTESIAN_POINT('Ctrl Pts',(2.09510876220501,-1.,0.594585006052824));
#25690=CARTESIAN_POINT('Ctrl Pts',(2.09954930865331,-1.,0.599241616422144));
#25691=CARTESIAN_POINT('Ctrl Pts',(2.10397049887709,-1.,0.603932030738212));
#25692=CARTESIAN_POINT('Ctrl Pts',(2.10749199615859,-1.,0.607711315456826));
#25693=CARTESIAN_POINT('Ctrl Pts',(2.11012443807661,-1.,0.610560911691114));
#25694=CARTESIAN_POINT('Ctrl Pts',(2.11187554260142,-1.,0.61246736556225));
#25695=CARTESIAN_POINT('Ctrl Pts',(2.11275013067528,-1.,0.613422273260091));
#25696=CARTESIAN_POINT('',(2.0698113262342,-1.,0.745574324794401));
#25697=CARTESIAN_POINT('',(2.11275013067528,-1.,0.613422273260091));
#25698=CARTESIAN_POINT('Ctrl Pts',(2.0698113262342,-1.,0.745574324794401));
#25699=CARTESIAN_POINT('Ctrl Pts',(2.06854248895575,-1.,0.74583279137781));
#25700=CARTESIAN_POINT('Ctrl Pts',(2.06600523016401,-1.,0.746345871542696));
#25701=CARTESIAN_POINT('Ctrl Pts',(2.06220058927162,-1.,0.747103932785504));
#25702=CARTESIAN_POINT('Ctrl Pts',(2.05713023030263,-1.,0.748091554181101));
#25703=CARTESIAN_POINT('Ctrl Pts',(2.05079645591606,-1.,0.749287468663053));
#25704=CARTESIAN_POINT('Ctrl Pts',(2.04446689147754,-1.,0.750444657874758));
#25705=CARTESIAN_POINT('Ctrl Pts',(2.03814160092173,-1.,0.751562963361384));
#25706=CARTESIAN_POINT('Ctrl Pts',(2.03182068456467,-1.,0.752642180488104));
#25707=CARTESIAN_POINT('Ctrl Pts',(2.02550428623587,-1.,0.753682061113766));
#25708=CARTESIAN_POINT('Ctrl Pts',(2.01919259406003,-1.,0.75468233072352));
#25709=CARTESIAN_POINT('Ctrl Pts',(2.01288584328149,-1.,0.755642704958101));
#25710=CARTESIAN_POINT('Ctrl Pts',(2.00658431587682,-1.,0.756562904646496));
#25711=CARTESIAN_POINT('Ctrl Pts',(2.00028834739072,-1.,0.757442676862342));
#25712=CARTESIAN_POINT('Ctrl Pts',(1.9939983109871,-1.,0.758281796766377));
#25713=CARTESIAN_POINT('Ctrl Pts',(1.98771456680806,-1.,0.759080037802243));
#25714=CARTESIAN_POINT('Ctrl Pts',(1.98143741418156,-1.,0.759837147452135));
#25715=CARTESIAN_POINT('Ctrl Pts',(1.97516705321521,-1.,0.760552825409856));
#25716=CARTESIAN_POINT('Ctrl Pts',(1.96890351582545,-1.,0.761226690483986));
#25717=CARTESIAN_POINT('Ctrl Pts',(1.96264672744229,-1.,0.761858300014575));
#25718=CARTESIAN_POINT('Ctrl Pts',(1.95639665309893,-1.,0.762447203806264));
#25719=CARTESIAN_POINT('Ctrl Pts',(1.95015342590025,-1.,0.762992990878774));
#25720=CARTESIAN_POINT('Ctrl Pts',(1.94391746617626,-1.,0.763495333538581));
#25721=CARTESIAN_POINT('Ctrl Pts',(1.93768964875867,-1.,0.763954049121394));
#25722=CARTESIAN_POINT('Ctrl Pts',(1.93147105496367,-1.,0.76436901067389));
#25723=CARTESIAN_POINT('Ctrl Pts',(1.92526263537041,-1.,0.764740025488189));
#25724=CARTESIAN_POINT('Ctrl Pts',(1.91906491634197,-1.,0.765066729667095));
#25725=CARTESIAN_POINT('Ctrl Pts',(1.91287765805174,-1.,0.765348465884739));
#25726=CARTESIAN_POINT('Ctrl Pts',(1.90669961402362,-1.,0.765584196937937));
#25727=CARTESIAN_POINT('Ctrl Pts',(1.90052930393599,-1.,0.765772772593395));
#25728=CARTESIAN_POINT('Ctrl Pts',(1.89436577771389,-1.,0.765913193856979));
#25729=CARTESIAN_POINT('Ctrl Pts',(1.88820926433409,-1.,0.76600483706209));
#25730=CARTESIAN_POINT('Ctrl Pts',(1.88206215302561,-1.,0.766047794851869));
#25731=CARTESIAN_POINT('Ctrl Pts',(1.87592888967886,-1.,0.766042837036759));
#25732=CARTESIAN_POINT('Ctrl Pts',(1.86981398314345,-1.,0.765990708546112));
#25733=CARTESIAN_POINT('Ctrl Pts',(1.86372027063314,-1.,0.765891519092557));
#25734=CARTESIAN_POINT('Ctrl Pts',(1.85764741390391,-1.,0.765744212909305));
#25735=CARTESIAN_POINT('Ctrl Pts',(1.85158945130054,-1.,0.765545710619023));
#25736=CARTESIAN_POINT('Ctrl Pts',(1.8455369887591,-1.,0.765291664861972));
#25737=CARTESIAN_POINT('Ctrl Pts',(1.83948181064823,-1.,0.764978057881688));
#25738=CARTESIAN_POINT('Ctrl Pts',(1.8334207722714,-1.,0.764602549687846));
#25739=CARTESIAN_POINT('Ctrl Pts',(1.8273599120008,-1.,0.764165902606056));
#25740=CARTESIAN_POINT('Ctrl Pts',(1.82131873145297,-1.,0.763673465462854));
#25741=CARTESIAN_POINT('Ctrl Pts',(1.81532118405566,-1.,0.763132003836783));
#25742=CARTESIAN_POINT('Ctrl Pts',(1.80938551463989,-1.,0.762546129464036));
#25743=CARTESIAN_POINT('Ctrl Pts',(1.80351583877334,-1.,0.761915336443516));
#25744=CARTESIAN_POINT('Ctrl Pts',(1.79768986997735,-1.,0.761229695230359));
#25745=CARTESIAN_POINT('Ctrl Pts',(1.79185815610802,-1.,0.760469555880425));
#25746=CARTESIAN_POINT('Ctrl Pts',(1.78596964884526,-1.,0.759614401109868));
#25747=CARTESIAN_POINT('Ctrl Pts',(1.77999411220912,-1.,0.75865062667738));
#25748=CARTESIAN_POINT('Ctrl Pts',(1.77394167108342,-1.,0.757578264077238));
#25749=CARTESIAN_POINT('Ctrl Pts',(1.76789396003141,-1.,0.756421896028403));
#25750=CARTESIAN_POINT('Ctrl Pts',(1.7619781724032,-1.,0.755220979975262));
#25751=CARTESIAN_POINT('Ctrl Pts',(1.75631083600175,-1.,0.75400925402848));
#25752=CARTESIAN_POINT('Ctrl Pts',(1.75095139468809,-1.,0.752797683531377));
#25753=CARTESIAN_POINT('Ctrl Pts',(1.74585086852298,-1.,0.751555614163629));
#25754=CARTESIAN_POINT('Ctrl Pts',(1.74080458266705,-1.,0.750193435979541));
#25755=CARTESIAN_POINT('Ctrl Pts',(1.73550351679848,-1.,0.748582462954855));
#25756=CARTESIAN_POINT('Ctrl Pts',(1.72958533647399,-1.,0.746574710096437));
#25757=CARTESIAN_POINT('Ctrl Pts',(1.7226822991693,-1.,0.744021445433765));
#25758=CARTESIAN_POINT('Ctrl Pts',(1.71447789751927,-1.,0.740795162032088));
#25759=CARTESIAN_POINT('Ctrl Pts',(1.70473309006121,-1.,0.736799665724771));
#25760=CARTESIAN_POINT('Ctrl Pts',(1.69326921975743,-1.,0.731963238697195));
#25761=CARTESIAN_POINT('Ctrl Pts',(1.67996158455503,-1.,0.726235967997433));
#25762=CARTESIAN_POINT('Ctrl Pts',(1.6647288055568,-1.,0.719585433804282));
#25763=CARTESIAN_POINT('Ctrl Pts',(1.64752408832016,-1.,0.711993139355394));
#25764=CARTESIAN_POINT('Ctrl Pts',(1.63216541664676,-1.,0.705159151988319));
#25765=CARTESIAN_POINT('Ctrl Pts',(1.61974673472612,-1.,0.699605146405088));
#25766=CARTESIAN_POINT('Ctrl Pts',(1.61106790958151,-1.,0.695712097881194));
#25767=CARTESIAN_POINT('Ctrl Pts',(1.60662857109684,-1.,0.693717979106306));
#25768=CARTESIAN_POINT('Origin',(0.,-1.,0.));
#25769=CARTESIAN_POINT('Origin',(0.,0.,0.));
#25770=CARTESIAN_POINT('Origin',(0.,2.2,0.));
#25771=CARTESIAN_POINT('Origin',(0.,1.,0.));
#25772=CARTESIAN_POINT('',(-1.4,2.2,1.71450551880629E-16));
#25773=CARTESIAN_POINT('Origin',(0.,2.2,0.));
#25774=CARTESIAN_POINT('',(-1.4,1.,1.71450551880629E-16));
#25775=CARTESIAN_POINT('',(-1.4,1.,1.71450551880629E-16));
#25776=CARTESIAN_POINT('Origin',(0.,1.,0.));
#25777=CARTESIAN_POINT('Origin',(0.,2.2,0.));
#25778=CARTESIAN_POINT('Ctrl Pts',(2.11275013067528,-1.,0.613422273260091));
#25779=CARTESIAN_POINT('Ctrl Pts',(2.11275013067528,1.,0.613422273260091));
#25780=CARTESIAN_POINT('Ctrl Pts',(2.11187554260142,-1.,0.61246736556225));
#25781=CARTESIAN_POINT('Ctrl Pts',(2.11187554260142,1.,0.61246736556225));
#25782=CARTESIAN_POINT('Ctrl Pts',(2.11012443807661,-1.,0.610560911691114));
#25783=CARTESIAN_POINT('Ctrl Pts',(2.11012443807661,1.,0.610560911691114));
#25784=CARTESIAN_POINT('Ctrl Pts',(2.10749199615859,-1.,0.607711315456826));
#25785=CARTESIAN_POINT('Ctrl Pts',(2.10749199615859,1.,0.607711315456826));
#25786=CARTESIAN_POINT('Ctrl Pts',(2.10397049887709,-1.,0.603932030738212));
#25787=CARTESIAN_POINT('Ctrl Pts',(2.10397049887709,1.,0.603932030738212));
#25788=CARTESIAN_POINT('Ctrl Pts',(2.09954930865331,-1.,0.599241616422144));
#25789=CARTESIAN_POINT('Ctrl Pts',(2.09954930865331,1.,0.599241616422144));
#25790=CARTESIAN_POINT('Ctrl Pts',(2.09510876220501,-1.,0.594585006052824));
#25791=CARTESIAN_POINT('Ctrl Pts',(2.09510876220501,1.,0.594585006052824));
#25792=CARTESIAN_POINT('Ctrl Pts',(2.09064881812053,-1.,0.58996236540319));
#25793=CARTESIAN_POINT('Ctrl Pts',(2.09064881812053,1.,0.58996236540319));
#25794=CARTESIAN_POINT('Ctrl Pts',(2.086169437277,-1.,0.585373918990895));
#25795=CARTESIAN_POINT('Ctrl Pts',(2.086169437277,1.,0.585373918990895));
#25796=CARTESIAN_POINT('Ctrl Pts',(2.08167059018138,-1.,0.580819952107257));
#25797=CARTESIAN_POINT('Ctrl Pts',(2.08167059018138,1.,0.580819952107257));
#25798=CARTESIAN_POINT('Ctrl Pts',(2.07715226767361,-1.,0.576300797416275));
#25799=CARTESIAN_POINT('Ctrl Pts',(2.07715226767361,1.,0.576300797416275));
#25800=CARTESIAN_POINT('Ctrl Pts',(2.07261449292757,-1.,0.571816823242411));
#25801=CARTESIAN_POINT('Ctrl Pts',(2.07261449292757,1.,0.571816823242411));
#25802=CARTESIAN_POINT('Ctrl Pts',(2.06805732997383,-1.,0.56736842118123));
#25803=CARTESIAN_POINT('Ctrl Pts',(2.06805732997383,1.,0.56736842118123));
#25804=CARTESIAN_POINT('Ctrl Pts',(2.06348090160697,-1.,0.562955993082574));
#25805=CARTESIAN_POINT('Ctrl Pts',(2.06348090160697,1.,0.562955993082574));
#25806=CARTESIAN_POINT('Ctrl Pts',(2.05888537756571,-1.,0.558579940185468));
#25807=CARTESIAN_POINT('Ctrl Pts',(2.05888537756571,1.,0.558579940185468));
#25808=CARTESIAN_POINT('Ctrl Pts',(2.05427091604482,-1.,0.55424065746411));
#25809=CARTESIAN_POINT('Ctrl Pts',(2.05427091604482,1.,0.55424065746411));
#25810=CARTESIAN_POINT('Ctrl Pts',(2.04963761077974,-1.,0.549938525150342));
#25811=CARTESIAN_POINT('Ctrl Pts',(2.04963761077974,1.,0.549938525150342));
#25812=CARTESIAN_POINT('Ctrl Pts',(2.0449854471456,-1.,0.545673903817349));
#25813=CARTESIAN_POINT('Ctrl Pts',(2.0449854471456,1.,0.545673903817349));
#25814=CARTESIAN_POINT('Ctrl Pts',(2.0403142269048,-1.,0.54144712061552));
#25815=CARTESIAN_POINT('Ctrl Pts',(2.0403142269048,1.,0.54144712061552));
#25816=CARTESIAN_POINT('Ctrl Pts',(2.03562362953993,-1.,0.537258489833135));
#25817=CARTESIAN_POINT('Ctrl Pts',(2.03562362953993,1.,0.537258489833135));
#25818=CARTESIAN_POINT('Ctrl Pts',(2.03091336214401,-1.,0.533108355132905));
#25819=CARTESIAN_POINT('Ctrl Pts',(2.03091336214401,1.,0.533108355132905));
#25820=CARTESIAN_POINT('Ctrl Pts',(2.02618329083289,-1.,0.528997127241911));
#25821=CARTESIAN_POINT('Ctrl Pts',(2.02618329083289,1.,0.528997127241911));
#25822=CARTESIAN_POINT('Ctrl Pts',(2.02143356304712,-1.,0.524925318333519));
#25823=CARTESIAN_POINT('Ctrl Pts',(2.02143356304712,1.,0.524925318333519));
#25824=CARTESIAN_POINT('Ctrl Pts',(2.01666477917305,-1.,0.520893590399429));
#25825=CARTESIAN_POINT('Ctrl Pts',(2.01666477917305,1.,0.520893590399429));
#25826=CARTESIAN_POINT('Ctrl Pts',(2.01187773939257,-1.,0.516902681728733));
#25827=CARTESIAN_POINT('Ctrl Pts',(2.01187773939257,1.,0.516902681728733));
#25828=CARTESIAN_POINT('Ctrl Pts',(2.00707309946955,-1.,0.512953306961814));
#25829=CARTESIAN_POINT('Ctrl Pts',(2.00707309946955,1.,0.512953306961814));
#25830=CARTESIAN_POINT('Ctrl Pts',(2.00225107134733,-1.,0.509046069886152));
#25831=CARTESIAN_POINT('Ctrl Pts',(2.00225107134733,1.,0.509046069886152));
#25832=CARTESIAN_POINT('Ctrl Pts',(1.99741107463567,-1.,0.505181361323011));
#25833=CARTESIAN_POINT('Ctrl Pts',(1.99741107463567,1.,0.505181361323011));
#25834=CARTESIAN_POINT('Ctrl Pts',(1.9925514912615,-1.,0.501359287727129));
#25835=CARTESIAN_POINT('Ctrl Pts',(1.9925514912615,1.,0.501359287727129));
#25836=CARTESIAN_POINT('Ctrl Pts',(1.98767044752929,-1.,0.497579909545564));
#25837=CARTESIAN_POINT('Ctrl Pts',(1.98767044752929,1.,0.497579909545564));
#25838=CARTESIAN_POINT('Ctrl Pts',(1.9827665876182,-1.,0.493843476541493));
#25839=CARTESIAN_POINT('Ctrl Pts',(1.9827665876182,1.,0.493843476541493));
#25840=CARTESIAN_POINT('Ctrl Pts',(1.97783973019229,-1.,0.490150627860955));
#25841=CARTESIAN_POINT('Ctrl Pts',(1.97783973019229,1.,0.490150627860955));
#25842=CARTESIAN_POINT('Ctrl Pts',(1.97289186263272,-1.,0.486502692907661));
#25843=CARTESIAN_POINT('Ctrl Pts',(1.97289186263272,1.,0.486502692907661));
#25844=CARTESIAN_POINT('Ctrl Pts',(1.96792703422358,-1.,0.482901662120687));
#25845=CARTESIAN_POINT('Ctrl Pts',(1.96792703422358,1.,0.482901662120687));
#25846=CARTESIAN_POINT('Ctrl Pts',(1.96294933055938,-1.,0.479349583074846));
#25847=CARTESIAN_POINT('Ctrl Pts',(1.96294933055938,1.,0.479349583074846));
#25848=CARTESIAN_POINT('Ctrl Pts',(1.95796111148175,-1.,0.475848034683172));
#25849=CARTESIAN_POINT('Ctrl Pts',(1.95796111148175,1.,0.475848034683172));
#25850=CARTESIAN_POINT('Ctrl Pts',(1.95296148278136,-1.,0.47239767226408));
#25851=CARTESIAN_POINT('Ctrl Pts',(1.95296148278136,1.,0.47239767226408));
#25852=CARTESIAN_POINT('Ctrl Pts',(1.94794381136524,-1.,0.468997482913158));
#25853=CARTESIAN_POINT('Ctrl Pts',(1.94794381136524,1.,0.468997482913158));
#25854=CARTESIAN_POINT('Ctrl Pts',(1.94289794196205,-1.,0.465645462026065));
#25855=CARTESIAN_POINT('Ctrl Pts',(1.94289794196205,1.,0.465645462026065));
#25856=CARTESIAN_POINT('Ctrl Pts',(1.93781486640834,-1.,0.462340031009087));
#25857=CARTESIAN_POINT('Ctrl Pts',(1.93781486640834,1.,0.462340031009087));
#25858=CARTESIAN_POINT('Ctrl Pts',(1.93269066517936,-1.,0.459081234547932));
#25859=CARTESIAN_POINT('Ctrl Pts',(1.93269066517936,1.,0.459081234547932));
#25860=CARTESIAN_POINT('Ctrl Pts',(1.92753067150461,-1.,0.455872005174336));
#25861=CARTESIAN_POINT('Ctrl Pts',(1.92753067150461,1.,0.455872005174336));
#25862=CARTESIAN_POINT('Ctrl Pts',(1.9223538064847,-1.,0.452719478359356));
#25863=CARTESIAN_POINT('Ctrl Pts',(1.9223538064847,1.,0.452719478359356));
#25864=CARTESIAN_POINT('Ctrl Pts',(1.91718342555717,-1.,0.449632260106572));
#25865=CARTESIAN_POINT('Ctrl Pts',(1.91718342555717,1.,0.449632260106572));
#25866=CARTESIAN_POINT('Ctrl Pts',(1.91203699981095,-1.,0.446617343485651));
#25867=CARTESIAN_POINT('Ctrl Pts',(1.91203699981095,1.,0.446617343485651));
#25868=CARTESIAN_POINT('Ctrl Pts',(1.90691756144906,-1.,0.443677556849171));
#25869=CARTESIAN_POINT('Ctrl Pts',(1.90691756144906,1.,0.443677556849171));
#25870=CARTESIAN_POINT('Ctrl Pts',(1.90180124389137,-1.,0.440807833704161));
#25871=CARTESIAN_POINT('Ctrl Pts',(1.90180124389137,1.,0.440807833704161));
#25872=CARTESIAN_POINT('Ctrl Pts',(1.89663648956549,-1.,0.437995003948443));
#25873=CARTESIAN_POINT('Ctrl Pts',(1.89663648956549,1.,0.437995003948443));
#25874=CARTESIAN_POINT('Ctrl Pts',(1.89136993975585,-1.,0.43522566096358));
#25875=CARTESIAN_POINT('Ctrl Pts',(1.89136993975585,1.,0.43522566096358));
#25876=CARTESIAN_POINT('Ctrl Pts',(1.88596913666828,-1.,0.432493038548833));
#25877=CARTESIAN_POINT('Ctrl Pts',(1.88596913666828,1.,0.432493038548833));
#25878=CARTESIAN_POINT('Ctrl Pts',(1.88044229001778,-1.,0.429803062482217));
#25879=CARTESIAN_POINT('Ctrl Pts',(1.88044229001778,1.,0.429803062482217));
#25880=CARTESIAN_POINT('Ctrl Pts',(1.87486989291333,-1.,0.427183828518743));
#25881=CARTESIAN_POINT('Ctrl Pts',(1.87486989291333,1.,0.427183828518743));
#25882=CARTESIAN_POINT('Ctrl Pts',(1.8693780394412,-1.,0.424678177290876));
#25883=CARTESIAN_POINT('Ctrl Pts',(1.8693780394412,1.,0.424678177290876));
#25884=CARTESIAN_POINT('Ctrl Pts',(1.86408083333863,-1.,0.422327307417885));
#25885=CARTESIAN_POINT('Ctrl Pts',(1.86408083333863,1.,0.422327307417885));
#25886=CARTESIAN_POINT('Ctrl Pts',(1.8590328109667,-1.,0.420157287975583));
#25887=CARTESIAN_POINT('Ctrl Pts',(1.8590328109667,1.,0.420157287975583));
#25888=CARTESIAN_POINT('Ctrl Pts',(1.8541763285645,-1.,0.418164129144046));
#25889=CARTESIAN_POINT('Ctrl Pts',(1.8541763285645,1.,0.418164129144046));
#25890=CARTESIAN_POINT('Ctrl Pts',(1.84929312930314,-1.,0.416300022039885));
#25891=CARTESIAN_POINT('Ctrl Pts',(1.84929312930314,1.,0.416300022039885));
#25892=CARTESIAN_POINT('Ctrl Pts',(1.84405757074218,-1.,0.414487438255542));
#25893=CARTESIAN_POINT('Ctrl Pts',(1.84405757074218,1.,0.414487438255542));
#25894=CARTESIAN_POINT('Ctrl Pts',(1.8380895347617,-1.,0.412633125322945));
#25895=CARTESIAN_POINT('Ctrl Pts',(1.8380895347617,1.,0.412633125322945));
#25896=CARTESIAN_POINT('Ctrl Pts',(1.83100408895047,-1.,0.410641256301276));
#25897=CARTESIAN_POINT('Ctrl Pts',(1.83100408895047,1.,0.410641256301276));
#25898=CARTESIAN_POINT('Ctrl Pts',(1.82247022677562,-1.,0.408428948106228));
#25899=CARTESIAN_POINT('Ctrl Pts',(1.82247022677562,1.,0.408428948106228));
#25900=CARTESIAN_POINT('Ctrl Pts',(1.81223801812013,-1.,0.405933518407176));
#25901=CARTESIAN_POINT('Ctrl Pts',(1.81223801812013,1.,0.405933518407176));
#25902=CARTESIAN_POINT('Ctrl Pts',(1.80012077173238,-1.,0.403107976163396));
#25903=CARTESIAN_POINT('Ctrl Pts',(1.80012077173238,1.,0.403107976163396));
#25904=CARTESIAN_POINT('Ctrl Pts',(1.78598826343754,-1.,0.399919403774156));
#25905=CARTESIAN_POINT('Ctrl Pts',(1.78598826343754,1.,0.399919403774156));
#25906=CARTESIAN_POINT('Ctrl Pts',(1.76975560043442,-1.,0.396346196110688));
#25907=CARTESIAN_POINT('Ctrl Pts',(1.76975560043442,1.,0.396346196110688));
#25908=CARTESIAN_POINT('Ctrl Pts',(1.75137405310193,-1.,0.392375812285396));
#25909=CARTESIAN_POINT('Ctrl Pts',(1.75137405310193,1.,0.392375812285396));
#25910=CARTESIAN_POINT('Ctrl Pts',(1.73493170972829,-1.,0.388877023502615));
#25911=CARTESIAN_POINT('Ctrl Pts',(1.73493170972829,1.,0.388877023502615));
#25912=CARTESIAN_POINT('Ctrl Pts',(1.72162022244582,-1.,0.386070790323281));
#25913=CARTESIAN_POINT('Ctrl Pts',(1.72162022244582,1.,0.386070790323281));
#25914=CARTESIAN_POINT('Ctrl Pts',(1.71231062891398,-1.,0.384119047314215));
#25915=CARTESIAN_POINT('Ctrl Pts',(1.71231062891398,1.,0.384119047314215));
#25916=CARTESIAN_POINT('Ctrl Pts',(1.7075470150345,-1.,0.383122945602004));
#25917=CARTESIAN_POINT('Ctrl Pts',(1.7075470150345,1.,0.383122945602004));
#25918=CARTESIAN_POINT('',(1.7075470150345,1.,0.383122945602004));
#25919=CARTESIAN_POINT('',(1.7075470150345,0.,0.383122945602005));
#25920=CARTESIAN_POINT('',(2.11275013067528,1.,0.613422273260091));
#25921=CARTESIAN_POINT('Ctrl Pts',(2.11275013067528,1.,0.613422273260091));
#25922=CARTESIAN_POINT('Ctrl Pts',(2.11187554260142,1.,0.61246736556225));
#25923=CARTESIAN_POINT('Ctrl Pts',(2.11012443807661,1.,0.610560911691114));
#25924=CARTESIAN_POINT('Ctrl Pts',(2.10749199615859,1.,0.607711315456826));
#25925=CARTESIAN_POINT('Ctrl Pts',(2.10397049887709,1.,0.603932030738212));
#25926=CARTESIAN_POINT('Ctrl Pts',(2.09954930865331,1.,0.599241616422144));
#25927=CARTESIAN_POINT('Ctrl Pts',(2.09510876220501,1.,0.594585006052824));
#25928=CARTESIAN_POINT('Ctrl Pts',(2.09064881812053,1.,0.58996236540319));
#25929=CARTESIAN_POINT('Ctrl Pts',(2.086169437277,1.,0.585373918990895));
#25930=CARTESIAN_POINT('Ctrl Pts',(2.08167059018138,1.,0.580819952107257));
#25931=CARTESIAN_POINT('Ctrl Pts',(2.07715226767361,1.,0.576300797416275));
#25932=CARTESIAN_POINT('Ctrl Pts',(2.07261449292757,1.,0.571816823242411));
#25933=CARTESIAN_POINT('Ctrl Pts',(2.06805732997383,1.,0.56736842118123));
#25934=CARTESIAN_POINT('Ctrl Pts',(2.06348090160697,1.,0.562955993082574));
#25935=CARTESIAN_POINT('Ctrl Pts',(2.05888537756571,1.,0.558579940185468));
#25936=CARTESIAN_POINT('Ctrl Pts',(2.05427091604482,1.,0.55424065746411));
#25937=CARTESIAN_POINT('Ctrl Pts',(2.04963761077974,1.,0.549938525150342));
#25938=CARTESIAN_POINT('Ctrl Pts',(2.0449854471456,1.,0.545673903817349));
#25939=CARTESIAN_POINT('Ctrl Pts',(2.0403142269048,1.,0.54144712061552));
#25940=CARTESIAN_POINT('Ctrl Pts',(2.03562362953993,1.,0.537258489833135));
#25941=CARTESIAN_POINT('Ctrl Pts',(2.03091336214401,1.,0.533108355132905));
#25942=CARTESIAN_POINT('Ctrl Pts',(2.02618329083289,1.,0.528997127241911));
#25943=CARTESIAN_POINT('Ctrl Pts',(2.02143356304712,1.,0.524925318333519));
#25944=CARTESIAN_POINT('Ctrl Pts',(2.01666477917305,1.,0.520893590399429));
#25945=CARTESIAN_POINT('Ctrl Pts',(2.01187773939257,1.,0.516902681728733));
#25946=CARTESIAN_POINT('Ctrl Pts',(2.00707309946955,1.,0.512953306961814));
#25947=CARTESIAN_POINT('Ctrl Pts',(2.00225107134733,1.,0.509046069886152));
#25948=CARTESIAN_POINT('Ctrl Pts',(1.99741107463567,1.,0.505181361323011));
#25949=CARTESIAN_POINT('Ctrl Pts',(1.9925514912615,1.,0.501359287727129));
#25950=CARTESIAN_POINT('Ctrl Pts',(1.98767044752929,1.,0.497579909545564));
#25951=CARTESIAN_POINT('Ctrl Pts',(1.9827665876182,1.,0.493843476541493));
#25952=CARTESIAN_POINT('Ctrl Pts',(1.97783973019229,1.,0.490150627860955));
#25953=CARTESIAN_POINT('Ctrl Pts',(1.97289186263272,1.,0.486502692907661));
#25954=CARTESIAN_POINT('Ctrl Pts',(1.96792703422358,1.,0.482901662120687));
#25955=CARTESIAN_POINT('Ctrl Pts',(1.96294933055938,1.,0.479349583074846));
#25956=CARTESIAN_POINT('Ctrl Pts',(1.95796111148175,1.,0.475848034683172));
#25957=CARTESIAN_POINT('Ctrl Pts',(1.95296148278136,1.,0.47239767226408));
#25958=CARTESIAN_POINT('Ctrl Pts',(1.94794381136524,1.,0.468997482913158));
#25959=CARTESIAN_POINT('Ctrl Pts',(1.94289794196205,1.,0.465645462026065));
#25960=CARTESIAN_POINT('Ctrl Pts',(1.93781486640834,1.,0.462340031009087));
#25961=CARTESIAN_POINT('Ctrl Pts',(1.93269066517936,1.,0.459081234547932));
#25962=CARTESIAN_POINT('Ctrl Pts',(1.92753067150461,1.,0.455872005174336));
#25963=CARTESIAN_POINT('Ctrl Pts',(1.9223538064847,1.,0.452719478359356));
#25964=CARTESIAN_POINT('Ctrl Pts',(1.91718342555717,1.,0.449632260106572));
#25965=CARTESIAN_POINT('Ctrl Pts',(1.91203699981095,1.,0.446617343485651));
#25966=CARTESIAN_POINT('Ctrl Pts',(1.90691756144906,1.,0.443677556849171));
#25967=CARTESIAN_POINT('Ctrl Pts',(1.90180124389137,1.,0.440807833704161));
#25968=CARTESIAN_POINT('Ctrl Pts',(1.89663648956549,1.,0.437995003948443));
#25969=CARTESIAN_POINT('Ctrl Pts',(1.89136993975585,1.,0.43522566096358));
#25970=CARTESIAN_POINT('Ctrl Pts',(1.88596913666828,1.,0.432493038548833));
#25971=CARTESIAN_POINT('Ctrl Pts',(1.88044229001778,1.,0.429803062482217));
#25972=CARTESIAN_POINT('Ctrl Pts',(1.87486989291333,1.,0.427183828518743));
#25973=CARTESIAN_POINT('Ctrl Pts',(1.8693780394412,1.,0.424678177290876));
#25974=CARTESIAN_POINT('Ctrl Pts',(1.86408083333863,1.,0.422327307417885));
#25975=CARTESIAN_POINT('Ctrl Pts',(1.8590328109667,1.,0.420157287975583));
#25976=CARTESIAN_POINT('Ctrl Pts',(1.8541763285645,1.,0.418164129144046));
#25977=CARTESIAN_POINT('Ctrl Pts',(1.84929312930314,1.,0.416300022039885));
#25978=CARTESIAN_POINT('Ctrl Pts',(1.84405757074218,1.,0.414487438255542));
#25979=CARTESIAN_POINT('Ctrl Pts',(1.8380895347617,1.,0.412633125322945));
#25980=CARTESIAN_POINT('Ctrl Pts',(1.83100408895047,1.,0.410641256301276));
#25981=CARTESIAN_POINT('Ctrl Pts',(1.82247022677562,1.,0.408428948106228));
#25982=CARTESIAN_POINT('Ctrl Pts',(1.81223801812013,1.,0.405933518407176));
#25983=CARTESIAN_POINT('Ctrl Pts',(1.80012077173238,1.,0.403107976163396));
#25984=CARTESIAN_POINT('Ctrl Pts',(1.78598826343754,1.,0.399919403774156));
#25985=CARTESIAN_POINT('Ctrl Pts',(1.76975560043442,1.,0.396346196110688));
#25986=CARTESIAN_POINT('Ctrl Pts',(1.75137405310193,1.,0.392375812285396));
#25987=CARTESIAN_POINT('Ctrl Pts',(1.73493170972829,1.,0.388877023502615));
#25988=CARTESIAN_POINT('Ctrl Pts',(1.72162022244582,1.,0.386070790323281));
#25989=CARTESIAN_POINT('Ctrl Pts',(1.71231062891398,1.,0.384119047314215));
#25990=CARTESIAN_POINT('Ctrl Pts',(1.7075470150345,1.,0.383122945602004));
#25991=CARTESIAN_POINT('',(2.11275013067528,0.,0.613422273260091));
#25992=CARTESIAN_POINT('Origin',(2.0698113262342,0.,0.745574324794401));
#25993=CARTESIAN_POINT('',(2.0698113262342,1.,0.745574324794401));
#25994=CARTESIAN_POINT('',(2.11275013067528,1.,0.613422273260091));
#25995=CARTESIAN_POINT('',(2.0698113262342,0.,0.745574324794401));
#25996=CARTESIAN_POINT('Ctrl Pts',(1.60662857109684,-1.,0.693717979106306));
#25997=CARTESIAN_POINT('Ctrl Pts',(1.60662857109684,1.,0.693717979106306));
#25998=CARTESIAN_POINT('Ctrl Pts',(1.61106790958151,-1.,0.695712097881194));
#25999=CARTESIAN_POINT('Ctrl Pts',(1.61106790958151,1.,0.695712097881194));
#26000=CARTESIAN_POINT('Ctrl Pts',(1.61974673472612,-1.,0.699605146405088));
#26001=CARTESIAN_POINT('Ctrl Pts',(1.61974673472612,1.,0.699605146405088));
#26002=CARTESIAN_POINT('Ctrl Pts',(1.63216541664676,-1.,0.705159151988319));
#26003=CARTESIAN_POINT('Ctrl Pts',(1.63216541664676,1.,0.705159151988319));
#26004=CARTESIAN_POINT('Ctrl Pts',(1.64752408832016,-1.,0.711993139355394));
#26005=CARTESIAN_POINT('Ctrl Pts',(1.64752408832016,1.,0.711993139355394));
#26006=CARTESIAN_POINT('Ctrl Pts',(1.6647288055568,-1.,0.719585433804282));
#26007=CARTESIAN_POINT('Ctrl Pts',(1.6647288055568,1.,0.719585433804282));
#26008=CARTESIAN_POINT('Ctrl Pts',(1.67996158455503,-1.,0.726235967997433));
#26009=CARTESIAN_POINT('Ctrl Pts',(1.67996158455503,1.,0.726235967997433));
#26010=CARTESIAN_POINT('Ctrl Pts',(1.69326921975743,-1.,0.731963238697195));
#26011=CARTESIAN_POINT('Ctrl Pts',(1.69326921975743,1.,0.731963238697195));
#26012=CARTESIAN_POINT('Ctrl Pts',(1.70473309006121,-1.,0.736799665724771));
#26013=CARTESIAN_POINT('Ctrl Pts',(1.70473309006121,1.,0.736799665724771));
#26014=CARTESIAN_POINT('Ctrl Pts',(1.71447789751927,-1.,0.740795162032088));
#26015=CARTESIAN_POINT('Ctrl Pts',(1.71447789751927,1.,0.740795162032088));
#26016=CARTESIAN_POINT('Ctrl Pts',(1.7226822991693,-1.,0.744021445433765));
#26017=CARTESIAN_POINT('Ctrl Pts',(1.7226822991693,1.,0.744021445433765));
#26018=CARTESIAN_POINT('Ctrl Pts',(1.72958533647399,-1.,0.746574710096437));
#26019=CARTESIAN_POINT('Ctrl Pts',(1.72958533647399,1.,0.746574710096437));
#26020=CARTESIAN_POINT('Ctrl Pts',(1.73550351679848,-1.,0.748582462954855));
#26021=CARTESIAN_POINT('Ctrl Pts',(1.73550351679848,1.,0.748582462954855));
#26022=CARTESIAN_POINT('Ctrl Pts',(1.74080458266705,-1.,0.750193435979541));
#26023=CARTESIAN_POINT('Ctrl Pts',(1.74080458266705,1.,0.750193435979541));
#26024=CARTESIAN_POINT('Ctrl Pts',(1.74585086852298,-1.,0.751555614163629));
#26025=CARTESIAN_POINT('Ctrl Pts',(1.74585086852298,1.,0.751555614163629));
#26026=CARTESIAN_POINT('Ctrl Pts',(1.75095139468809,-1.,0.752797683531377));
#26027=CARTESIAN_POINT('Ctrl Pts',(1.75095139468809,1.,0.752797683531377));
#26028=CARTESIAN_POINT('Ctrl Pts',(1.75631083600175,-1.,0.75400925402848));
#26029=CARTESIAN_POINT('Ctrl Pts',(1.75631083600175,1.,0.75400925402848));
#26030=CARTESIAN_POINT('Ctrl Pts',(1.7619781724032,-1.,0.755220979975262));
#26031=CARTESIAN_POINT('Ctrl Pts',(1.7619781724032,1.,0.755220979975262));
#26032=CARTESIAN_POINT('Ctrl Pts',(1.76789396003141,-1.,0.756421896028403));
#26033=CARTESIAN_POINT('Ctrl Pts',(1.76789396003141,1.,0.756421896028403));
#26034=CARTESIAN_POINT('Ctrl Pts',(1.77394167108342,-1.,0.757578264077238));
#26035=CARTESIAN_POINT('Ctrl Pts',(1.77394167108342,1.,0.757578264077238));
#26036=CARTESIAN_POINT('Ctrl Pts',(1.77999411220912,-1.,0.75865062667738));
#26037=CARTESIAN_POINT('Ctrl Pts',(1.77999411220912,1.,0.75865062667738));
#26038=CARTESIAN_POINT('Ctrl Pts',(1.78596964884526,-1.,0.759614401109868));
#26039=CARTESIAN_POINT('Ctrl Pts',(1.78596964884526,1.,0.759614401109868));
#26040=CARTESIAN_POINT('Ctrl Pts',(1.79185815610802,-1.,0.760469555880425));
#26041=CARTESIAN_POINT('Ctrl Pts',(1.79185815610802,1.,0.760469555880425));
#26042=CARTESIAN_POINT('Ctrl Pts',(1.79768986997735,-1.,0.761229695230359));
#26043=CARTESIAN_POINT('Ctrl Pts',(1.79768986997735,1.,0.761229695230359));
#26044=CARTESIAN_POINT('Ctrl Pts',(1.80351583877334,-1.,0.761915336443516));
#26045=CARTESIAN_POINT('Ctrl Pts',(1.80351583877334,1.,0.761915336443516));
#26046=CARTESIAN_POINT('Ctrl Pts',(1.80938551463989,-1.,0.762546129464036));
#26047=CARTESIAN_POINT('Ctrl Pts',(1.80938551463989,1.,0.762546129464036));
#26048=CARTESIAN_POINT('Ctrl Pts',(1.81532118405566,-1.,0.763132003836783));
#26049=CARTESIAN_POINT('Ctrl Pts',(1.81532118405566,1.,0.763132003836783));
#26050=CARTESIAN_POINT('Ctrl Pts',(1.82131873145297,-1.,0.763673465462854));
#26051=CARTESIAN_POINT('Ctrl Pts',(1.82131873145297,1.,0.763673465462854));
#26052=CARTESIAN_POINT('Ctrl Pts',(1.8273599120008,-1.,0.764165902606056));
#26053=CARTESIAN_POINT('Ctrl Pts',(1.8273599120008,1.,0.764165902606056));
#26054=CARTESIAN_POINT('Ctrl Pts',(1.8334207722714,-1.,0.764602549687846));
#26055=CARTESIAN_POINT('Ctrl Pts',(1.8334207722714,1.,0.764602549687846));
#26056=CARTESIAN_POINT('Ctrl Pts',(1.83948181064823,-1.,0.764978057881688));
#26057=CARTESIAN_POINT('Ctrl Pts',(1.83948181064823,1.,0.764978057881688));
#26058=CARTESIAN_POINT('Ctrl Pts',(1.8455369887591,-1.,0.765291664861972));
#26059=CARTESIAN_POINT('Ctrl Pts',(1.8455369887591,1.,0.765291664861972));
#26060=CARTESIAN_POINT('Ctrl Pts',(1.85158945130054,-1.,0.765545710619023));
#26061=CARTESIAN_POINT('Ctrl Pts',(1.85158945130054,1.,0.765545710619023));
#26062=CARTESIAN_POINT('Ctrl Pts',(1.85764741390391,-1.,0.765744212909305));
#26063=CARTESIAN_POINT('Ctrl Pts',(1.85764741390391,1.,0.765744212909305));
#26064=CARTESIAN_POINT('Ctrl Pts',(1.86372027063314,-1.,0.765891519092557));
#26065=CARTESIAN_POINT('Ctrl Pts',(1.86372027063314,1.,0.765891519092557));
#26066=CARTESIAN_POINT('Ctrl Pts',(1.86981398314345,-1.,0.765990708546112));
#26067=CARTESIAN_POINT('Ctrl Pts',(1.86981398314345,1.,0.765990708546112));
#26068=CARTESIAN_POINT('Ctrl Pts',(1.87592888967886,-1.,0.766042837036759));
#26069=CARTESIAN_POINT('Ctrl Pts',(1.87592888967886,1.,0.766042837036759));
#26070=CARTESIAN_POINT('Ctrl Pts',(1.88206215302561,-1.,0.766047794851869));
#26071=CARTESIAN_POINT('Ctrl Pts',(1.88206215302561,1.,0.766047794851869));
#26072=CARTESIAN_POINT('Ctrl Pts',(1.88820926433409,-1.,0.76600483706209));
#26073=CARTESIAN_POINT('Ctrl Pts',(1.88820926433409,1.,0.76600483706209));
#26074=CARTESIAN_POINT('Ctrl Pts',(1.89436577771389,-1.,0.765913193856979));
#26075=CARTESIAN_POINT('Ctrl Pts',(1.89436577771389,1.,0.765913193856979));
#26076=CARTESIAN_POINT('Ctrl Pts',(1.90052930393599,-1.,0.765772772593395));
#26077=CARTESIAN_POINT('Ctrl Pts',(1.90052930393599,1.,0.765772772593395));
#26078=CARTESIAN_POINT('Ctrl Pts',(1.90669961402362,-1.,0.765584196937937));
#26079=CARTESIAN_POINT('Ctrl Pts',(1.90669961402362,1.,0.765584196937937));
#26080=CARTESIAN_POINT('Ctrl Pts',(1.91287765805174,-1.,0.765348465884739));
#26081=CARTESIAN_POINT('Ctrl Pts',(1.91287765805174,1.,0.765348465884739));
#26082=CARTESIAN_POINT('Ctrl Pts',(1.91906491634197,-1.,0.765066729667095));
#26083=CARTESIAN_POINT('Ctrl Pts',(1.91906491634197,1.,0.765066729667095));
#26084=CARTESIAN_POINT('Ctrl Pts',(1.92526263537041,-1.,0.764740025488189));
#26085=CARTESIAN_POINT('Ctrl Pts',(1.92526263537041,1.,0.764740025488189));
#26086=CARTESIAN_POINT('Ctrl Pts',(1.93147105496367,-1.,0.76436901067389));
#26087=CARTESIAN_POINT('Ctrl Pts',(1.93147105496367,1.,0.76436901067389));
#26088=CARTESIAN_POINT('Ctrl Pts',(1.93768964875867,-1.,0.763954049121394));
#26089=CARTESIAN_POINT('Ctrl Pts',(1.93768964875867,1.,0.763954049121394));
#26090=CARTESIAN_POINT('Ctrl Pts',(1.94391746617626,-1.,0.763495333538581));
#26091=CARTESIAN_POINT('Ctrl Pts',(1.94391746617626,1.,0.763495333538581));
#26092=CARTESIAN_POINT('Ctrl Pts',(1.95015342590025,-1.,0.762992990878774));
#26093=CARTESIAN_POINT('Ctrl Pts',(1.95015342590025,1.,0.762992990878774));
#26094=CARTESIAN_POINT('Ctrl Pts',(1.95639665309893,-1.,0.762447203806264));
#26095=CARTESIAN_POINT('Ctrl Pts',(1.95639665309893,1.,0.762447203806264));
#26096=CARTESIAN_POINT('Ctrl Pts',(1.96264672744229,-1.,0.761858300014575));
#26097=CARTESIAN_POINT('Ctrl Pts',(1.96264672744229,1.,0.761858300014575));
#26098=CARTESIAN_POINT('Ctrl Pts',(1.96890351582545,-1.,0.761226690483986));
#26099=CARTESIAN_POINT('Ctrl Pts',(1.96890351582545,1.,0.761226690483986));
#26100=CARTESIAN_POINT('Ctrl Pts',(1.97516705321521,-1.,0.760552825409856));
#26101=CARTESIAN_POINT('Ctrl Pts',(1.97516705321521,1.,0.760552825409856));
#26102=CARTESIAN_POINT('Ctrl Pts',(1.98143741418156,-1.,0.759837147452135));
#26103=CARTESIAN_POINT('Ctrl Pts',(1.98143741418156,1.,0.759837147452135));
#26104=CARTESIAN_POINT('Ctrl Pts',(1.98771456680806,-1.,0.759080037802243));
#26105=CARTESIAN_POINT('Ctrl Pts',(1.98771456680806,1.,0.759080037802243));
#26106=CARTESIAN_POINT('Ctrl Pts',(1.9939983109871,-1.,0.758281796766377));
#26107=CARTESIAN_POINT('Ctrl Pts',(1.9939983109871,1.,0.758281796766377));
#26108=CARTESIAN_POINT('Ctrl Pts',(2.00028834739072,-1.,0.757442676862342));
#26109=CARTESIAN_POINT('Ctrl Pts',(2.00028834739072,1.,0.757442676862342));
#26110=CARTESIAN_POINT('Ctrl Pts',(2.00658431587682,-1.,0.756562904646496));
#26111=CARTESIAN_POINT('Ctrl Pts',(2.00658431587682,1.,0.756562904646496));
#26112=CARTESIAN_POINT('Ctrl Pts',(2.01288584328149,-1.,0.755642704958101));
#26113=CARTESIAN_POINT('Ctrl Pts',(2.01288584328149,1.,0.755642704958101));
#26114=CARTESIAN_POINT('Ctrl Pts',(2.01919259406003,-1.,0.75468233072352));
#26115=CARTESIAN_POINT('Ctrl Pts',(2.01919259406003,1.,0.75468233072352));
#26116=CARTESIAN_POINT('Ctrl Pts',(2.02550428623587,-1.,0.753682061113766));
#26117=CARTESIAN_POINT('Ctrl Pts',(2.02550428623587,1.,0.753682061113766));
#26118=CARTESIAN_POINT('Ctrl Pts',(2.03182068456467,-1.,0.752642180488104));
#26119=CARTESIAN_POINT('Ctrl Pts',(2.03182068456467,1.,0.752642180488104));
#26120=CARTESIAN_POINT('Ctrl Pts',(2.03814160092173,-1.,0.751562963361384));
#26121=CARTESIAN_POINT('Ctrl Pts',(2.03814160092173,1.,0.751562963361384));
#26122=CARTESIAN_POINT('Ctrl Pts',(2.04446689147754,-1.,0.750444657874758));
#26123=CARTESIAN_POINT('Ctrl Pts',(2.04446689147754,1.,0.750444657874758));
#26124=CARTESIAN_POINT('Ctrl Pts',(2.05079645591606,-1.,0.749287468663053));
#26125=CARTESIAN_POINT('Ctrl Pts',(2.05079645591606,1.,0.749287468663053));
#26126=CARTESIAN_POINT('Ctrl Pts',(2.05713023030263,-1.,0.748091554181101));
#26127=CARTESIAN_POINT('Ctrl Pts',(2.05713023030263,1.,0.748091554181101));
#26128=CARTESIAN_POINT('Ctrl Pts',(2.06220058927162,-1.,0.747103932785504));
#26129=CARTESIAN_POINT('Ctrl Pts',(2.06220058927162,1.,0.747103932785504));
#26130=CARTESIAN_POINT('Ctrl Pts',(2.06600523016401,-1.,0.746345871542696));
#26131=CARTESIAN_POINT('Ctrl Pts',(2.06600523016401,1.,0.746345871542696));
#26132=CARTESIAN_POINT('Ctrl Pts',(2.06854248895575,-1.,0.74583279137781));
#26133=CARTESIAN_POINT('Ctrl Pts',(2.06854248895575,1.,0.74583279137781));
#26134=CARTESIAN_POINT('Ctrl Pts',(2.0698113262342,-1.,0.745574324794401));
#26135=CARTESIAN_POINT('Ctrl Pts',(2.0698113262342,1.,0.745574324794401));
#26136=CARTESIAN_POINT('',(1.60662857109684,1.,0.693717979106306));
#26137=CARTESIAN_POINT('Ctrl Pts',(1.60662857109684,1.,0.693717979106306));
#26138=CARTESIAN_POINT('Ctrl Pts',(1.61106790958151,1.,0.695712097881194));
#26139=CARTESIAN_POINT('Ctrl Pts',(1.61974673472612,1.,0.699605146405088));
#26140=CARTESIAN_POINT('Ctrl Pts',(1.63216541664676,1.,0.705159151988319));
#26141=CARTESIAN_POINT('Ctrl Pts',(1.64752408832016,1.,0.711993139355394));
#26142=CARTESIAN_POINT('Ctrl Pts',(1.6647288055568,1.,0.719585433804282));
#26143=CARTESIAN_POINT('Ctrl Pts',(1.67996158455503,1.,0.726235967997433));
#26144=CARTESIAN_POINT('Ctrl Pts',(1.69326921975743,1.,0.731963238697195));
#26145=CARTESIAN_POINT('Ctrl Pts',(1.70473309006121,1.,0.736799665724771));
#26146=CARTESIAN_POINT('Ctrl Pts',(1.71447789751927,1.,0.740795162032088));
#26147=CARTESIAN_POINT('Ctrl Pts',(1.7226822991693,1.,0.744021445433765));
#26148=CARTESIAN_POINT('Ctrl Pts',(1.72958533647399,1.,0.746574710096437));
#26149=CARTESIAN_POINT('Ctrl Pts',(1.73550351679848,1.,0.748582462954855));
#26150=CARTESIAN_POINT('Ctrl Pts',(1.74080458266705,1.,0.750193435979541));
#26151=CARTESIAN_POINT('Ctrl Pts',(1.74585086852298,1.,0.751555614163629));
#26152=CARTESIAN_POINT('Ctrl Pts',(1.75095139468809,1.,0.752797683531377));
#26153=CARTESIAN_POINT('Ctrl Pts',(1.75631083600175,1.,0.75400925402848));
#26154=CARTESIAN_POINT('Ctrl Pts',(1.7619781724032,1.,0.755220979975262));
#26155=CARTESIAN_POINT('Ctrl Pts',(1.76789396003141,1.,0.756421896028403));
#26156=CARTESIAN_POINT('Ctrl Pts',(1.77394167108342,1.,0.757578264077238));
#26157=CARTESIAN_POINT('Ctrl Pts',(1.77999411220912,1.,0.75865062667738));
#26158=CARTESIAN_POINT('Ctrl Pts',(1.78596964884526,1.,0.759614401109868));
#26159=CARTESIAN_POINT('Ctrl Pts',(1.79185815610802,1.,0.760469555880425));
#26160=CARTESIAN_POINT('Ctrl Pts',(1.79768986997735,1.,0.761229695230359));
#26161=CARTESIAN_POINT('Ctrl Pts',(1.80351583877334,1.,0.761915336443516));
#26162=CARTESIAN_POINT('Ctrl Pts',(1.80938551463989,1.,0.762546129464036));
#26163=CARTESIAN_POINT('Ctrl Pts',(1.81532118405566,1.,0.763132003836783));
#26164=CARTESIAN_POINT('Ctrl Pts',(1.82131873145297,1.,0.763673465462854));
#26165=CARTESIAN_POINT('Ctrl Pts',(1.8273599120008,1.,0.764165902606056));
#26166=CARTESIAN_POINT('Ctrl Pts',(1.8334207722714,1.,0.764602549687846));
#26167=CARTESIAN_POINT('Ctrl Pts',(1.83948181064823,1.,0.764978057881688));
#26168=CARTESIAN_POINT('Ctrl Pts',(1.8455369887591,1.,0.765291664861972));
#26169=CARTESIAN_POINT('Ctrl Pts',(1.85158945130054,1.,0.765545710619023));
#26170=CARTESIAN_POINT('Ctrl Pts',(1.85764741390391,1.,0.765744212909305));
#26171=CARTESIAN_POINT('Ctrl Pts',(1.86372027063314,1.,0.765891519092557));
#26172=CARTESIAN_POINT('Ctrl Pts',(1.86981398314345,1.,0.765990708546112));
#26173=CARTESIAN_POINT('Ctrl Pts',(1.87592888967886,1.,0.766042837036759));
#26174=CARTESIAN_POINT('Ctrl Pts',(1.88206215302561,1.,0.766047794851869));
#26175=CARTESIAN_POINT('Ctrl Pts',(1.88820926433409,1.,0.76600483706209));
#26176=CARTESIAN_POINT('Ctrl Pts',(1.89436577771389,1.,0.765913193856979));
#26177=CARTESIAN_POINT('Ctrl Pts',(1.90052930393599,1.,0.765772772593395));
#26178=CARTESIAN_POINT('Ctrl Pts',(1.90669961402362,1.,0.765584196937937));
#26179=CARTESIAN_POINT('Ctrl Pts',(1.91287765805174,1.,0.765348465884739));
#26180=CARTESIAN_POINT('Ctrl Pts',(1.91906491634197,1.,0.765066729667095));
#26181=CARTESIAN_POINT('Ctrl Pts',(1.92526263537041,1.,0.764740025488189));
#26182=CARTESIAN_POINT('Ctrl Pts',(1.93147105496367,1.,0.76436901067389));
#26183=CARTESIAN_POINT('Ctrl Pts',(1.93768964875867,1.,0.763954049121394));
#26184=CARTESIAN_POINT('Ctrl Pts',(1.94391746617626,1.,0.763495333538581));
#26185=CARTESIAN_POINT('Ctrl Pts',(1.95015342590025,1.,0.762992990878774));
#26186=CARTESIAN_POINT('Ctrl Pts',(1.95639665309893,1.,0.762447203806264));
#26187=CARTESIAN_POINT('Ctrl Pts',(1.96264672744229,1.,0.761858300014575));
#26188=CARTESIAN_POINT('Ctrl Pts',(1.96890351582545,1.,0.761226690483986));
#26189=CARTESIAN_POINT('Ctrl Pts',(1.97516705321521,1.,0.760552825409856));
#26190=CARTESIAN_POINT('Ctrl Pts',(1.98143741418156,1.,0.759837147452135));
#26191=CARTESIAN_POINT('Ctrl Pts',(1.98771456680806,1.,0.759080037802243));
#26192=CARTESIAN_POINT('Ctrl Pts',(1.9939983109871,1.,0.758281796766377));
#26193=CARTESIAN_POINT('Ctrl Pts',(2.00028834739072,1.,0.757442676862342));
#26194=CARTESIAN_POINT('Ctrl Pts',(2.00658431587682,1.,0.756562904646496));
#26195=CARTESIAN_POINT('Ctrl Pts',(2.01288584328149,1.,0.755642704958101));
#26196=CARTESIAN_POINT('Ctrl Pts',(2.01919259406003,1.,0.75468233072352));
#26197=CARTESIAN_POINT('Ctrl Pts',(2.02550428623587,1.,0.753682061113766));
#26198=CARTESIAN_POINT('Ctrl Pts',(2.03182068456467,1.,0.752642180488104));
#26199=CARTESIAN_POINT('Ctrl Pts',(2.03814160092173,1.,0.751562963361384));
#26200=CARTESIAN_POINT('Ctrl Pts',(2.04446689147754,1.,0.750444657874758));
#26201=CARTESIAN_POINT('Ctrl Pts',(2.05079645591606,1.,0.749287468663053));
#26202=CARTESIAN_POINT('Ctrl Pts',(2.05713023030263,1.,0.748091554181101));
#26203=CARTESIAN_POINT('Ctrl Pts',(2.06220058927162,1.,0.747103932785504));
#26204=CARTESIAN_POINT('Ctrl Pts',(2.06600523016401,1.,0.746345871542696));
#26205=CARTESIAN_POINT('Ctrl Pts',(2.06854248895575,1.,0.74583279137781));
#26206=CARTESIAN_POINT('Ctrl Pts',(2.0698113262342,1.,0.745574324794401));
#26207=CARTESIAN_POINT('',(1.60662857109684,0.,0.693717979106305));
#26208=CARTESIAN_POINT('Origin',(0.,0.,0.));
#26209=CARTESIAN_POINT('',(1.5055822144029,1.,0.892032620296856));
#26210=CARTESIAN_POINT('Origin',(0.,1.,0.));
#26211=CARTESIAN_POINT('',(1.5055822144029,0.,0.892032620296855));
#26212=CARTESIAN_POINT('Ctrl Pts',(1.81978687191668,-1.,1.23627494547115));
#26213=CARTESIAN_POINT('Ctrl Pts',(1.81978687191668,1.,1.23627494547115));
#26214=CARTESIAN_POINT('Ctrl Pts',(1.81925017193666,-1.,1.23509651170476));
#26215=CARTESIAN_POINT('Ctrl Pts',(1.81925017193666,1.,1.23509651170476));
#26216=CARTESIAN_POINT('Ctrl Pts',(1.81817389921279,-1.,1.2327422452705));
#26217=CARTESIAN_POINT('Ctrl Pts',(1.81817389921279,1.,1.2327422452705));
#26218=CARTESIAN_POINT('Ctrl Pts',(1.8165508718364,-1.,1.2292186489137));
#26219=CARTESIAN_POINT('Ctrl Pts',(1.8165508718364,1.,1.2292186489137));
#26220=CARTESIAN_POINT('Ctrl Pts',(1.81436959210434,-1.,1.2245361330495));
#26221=CARTESIAN_POINT('Ctrl Pts',(1.81436959210434,1.,1.2245361330495));
#26222=CARTESIAN_POINT('Ctrl Pts',(1.81161420806656,-1.,1.21870906103557));
#26223=CARTESIAN_POINT('Ctrl Pts',(1.81161420806656,1.,1.21870906103557));
#26224=CARTESIAN_POINT('Ctrl Pts',(1.80882996917129,-1.,1.21290815708314));
#26225=CARTESIAN_POINT('Ctrl Pts',(1.80882996917129,1.,1.21290815708314));
#26226=CARTESIAN_POINT('Ctrl Pts',(1.80601678480707,-1.,1.20713356605475));
#26227=CARTESIAN_POINT('Ctrl Pts',(1.80601678480707,1.,1.20713356605475));
#26228=CARTESIAN_POINT('Ctrl Pts',(1.80317454838603,-1.,1.20138548938974));
#26229=CARTESIAN_POINT('Ctrl Pts',(1.80317454838603,1.,1.20138548938974));
#26230=CARTESIAN_POINT('Ctrl Pts',(1.80030314369879,-1.,1.19566418930242));
#26231=CARTESIAN_POINT('Ctrl Pts',(1.80030314369879,1.,1.19566418930242));
#26232=CARTESIAN_POINT('Ctrl Pts',(1.79740245923478,-1.,1.18996997934445));
#26233=CARTESIAN_POINT('Ctrl Pts',(1.79740245923478,1.,1.18996997934445));
#26234=CARTESIAN_POINT('Ctrl Pts',(1.79447240321515,-1.,1.18430321697432));
#26235=CARTESIAN_POINT('Ctrl Pts',(1.79447240321515,1.,1.18430321697432));
#26236=CARTESIAN_POINT('Ctrl Pts',(1.79151291552689,-1.,1.17866429440809));
#26237=CARTESIAN_POINT('Ctrl Pts',(1.79151291552689,1.,1.17866429440809));
#26238=CARTESIAN_POINT('Ctrl Pts',(1.78852398877616,-1.,1.17305363177328));
#26239=CARTESIAN_POINT('Ctrl Pts',(1.78852398877616,1.,1.17305363177328));
#26240=CARTESIAN_POINT('Ctrl Pts',(1.78550566040443,-1.,1.16747166312303));
#26241=CARTESIAN_POINT('Ctrl Pts',(1.78550566040443,1.,1.16747166312303));
#26242=CARTESIAN_POINT('Ctrl Pts',(1.78245795881009,-1.,1.16191881298499));
#26243=CARTESIAN_POINT('Ctrl Pts',(1.78245795881009,1.,1.16191881298499));
#26244=CARTESIAN_POINT('Ctrl Pts',(1.77938085564275,-1.,1.15639547194698));
#26245=CARTESIAN_POINT('Ctrl Pts',(1.77938085564275,1.,1.15639547194698));
#26246=CARTESIAN_POINT('Ctrl Pts',(1.7762742255701,-1.,1.15090197841515));
#26247=CARTESIAN_POINT('Ctrl Pts',(1.7762742255701,1.,1.15090197841515));
#26248=CARTESIAN_POINT('Ctrl Pts',(1.77313777896194,-1.,1.1454385822692));
#26249=CARTESIAN_POINT('Ctrl Pts',(1.77313777896194,1.,1.1454385822692));
#26250=CARTESIAN_POINT('Ctrl Pts',(1.76997111386769,-1.,1.14000548336975));
#26251=CARTESIAN_POINT('Ctrl Pts',(1.76997111386769,1.,1.14000548336975));
#26252=CARTESIAN_POINT('Ctrl Pts',(1.76677384551862,-1.,1.1346029180462));
#26253=CARTESIAN_POINT('Ctrl Pts',(1.76677384551862,1.,1.1346029180462));
#26254=CARTESIAN_POINT('Ctrl Pts',(1.7635457196617,-1.,1.12923123555075));
#26255=CARTESIAN_POINT('Ctrl Pts',(1.7635457196617,1.,1.12923123555075));
#26256=CARTESIAN_POINT('Ctrl Pts',(1.76028671825096,-1.,1.12389096855086));
#26257=CARTESIAN_POINT('Ctrl Pts',(1.76028671825096,1.,1.12389096855086));
#26258=CARTESIAN_POINT('Ctrl Pts',(1.75699720772105,-1.,1.11858293216763));
#26259=CARTESIAN_POINT('Ctrl Pts',(1.75699720772105,1.,1.11858293216763));
#26260=CARTESIAN_POINT('Ctrl Pts',(1.7536777209463,-1.,1.11330807582551));
#26261=CARTESIAN_POINT('Ctrl Pts',(1.7536777209463,1.,1.11330807582551));
#26262=CARTESIAN_POINT('Ctrl Pts',(1.7503286607592,-1.,1.10806728183007));
#26263=CARTESIAN_POINT('Ctrl Pts',(1.7503286607592,1.,1.10806728183007));
#26264=CARTESIAN_POINT('Ctrl Pts',(1.74695004214923,-1.,1.10286118991143));
#26265=CARTESIAN_POINT('Ctrl Pts',(1.74695004214923,1.,1.10286118991143));
#26266=CARTESIAN_POINT('Ctrl Pts',(1.74354119236208,-1.,1.09768999241226));
#26267=CARTESIAN_POINT('Ctrl Pts',(1.74354119236208,1.,1.09768999241226));
#26268=CARTESIAN_POINT('Ctrl Pts',(1.74010053962247,-1.,1.09255329056493));
#26269=CARTESIAN_POINT('Ctrl Pts',(1.74010053962247,1.,1.09255329056493));
#26270=CARTESIAN_POINT('Ctrl Pts',(1.73662628326091,-1.,1.08745056285427));
#26271=CARTESIAN_POINT('Ctrl Pts',(1.73662628326091,1.,1.08745056285427));
#26272=CARTESIAN_POINT('Ctrl Pts',(1.73311705663407,-1.,1.08238162784749));
#26273=CARTESIAN_POINT('Ctrl Pts',(1.73311705663407,1.,1.08238162784749));
#26274=CARTESIAN_POINT('Ctrl Pts',(1.72957248977424,-1.,1.0773470373727));
#26275=CARTESIAN_POINT('Ctrl Pts',(1.72957248977424,1.,1.0773470373727));
#26276=CARTESIAN_POINT('Ctrl Pts',(1.72599406198488,-1.,1.07234866990252));
#26277=CARTESIAN_POINT('Ctrl Pts',(1.72599406198488,1.,1.07234866990252));
#26278=CARTESIAN_POINT('Ctrl Pts',(1.72238500928453,-1.,1.06738966975462));
#26279=CARTESIAN_POINT('Ctrl Pts',(1.72238500928453,1.,1.06738966975462));
#26280=CARTESIAN_POINT('Ctrl Pts',(1.71874858456904,-1.,1.06247324680647));
#26281=CARTESIAN_POINT('Ctrl Pts',(1.71874858456904,1.,1.06247324680647));
#26282=CARTESIAN_POINT('Ctrl Pts',(1.7150865442702,-1.,1.05760163192479));
#26283=CARTESIAN_POINT('Ctrl Pts',(1.7150865442702,1.,1.05760163192479));
#26284=CARTESIAN_POINT('Ctrl Pts',(1.71139783543989,-1.,1.05277517202855));
#26285=CARTESIAN_POINT('Ctrl Pts',(1.71139783543989,1.,1.05277517202855));
#26286=CARTESIAN_POINT('Ctrl Pts',(1.70767646263649,-1.,1.04799085404995));
#26287=CARTESIAN_POINT('Ctrl Pts',(1.70767646263649,1.,1.04799085404995));
#26288=CARTESIAN_POINT('Ctrl Pts',(1.70391338707982,-1.,1.04324363334554));
#26289=CARTESIAN_POINT('Ctrl Pts',(1.70391338707982,1.,1.04324363334554));
#26290=CARTESIAN_POINT('Ctrl Pts',(1.70010052930962,-1.,1.03852922490789));
#26291=CARTESIAN_POINT('Ctrl Pts',(1.70010052930962,1.,1.03852922490789));
#26292=CARTESIAN_POINT('Ctrl Pts',(1.69623414782771,-1.,1.03384646003588));
#26293=CARTESIAN_POINT('Ctrl Pts',(1.69623414782771,1.,1.03384646003588));
#26294=CARTESIAN_POINT('Ctrl Pts',(1.69231840863458,-1.,1.02919977579147));
#26295=CARTESIAN_POINT('Ctrl Pts',(1.69231840863458,1.,1.02919977579147));
#26296=CARTESIAN_POINT('Ctrl Pts',(1.68836910178447,-1.,1.02460180535255));
#26297=CARTESIAN_POINT('Ctrl Pts',(1.68836910178447,1.,1.02460180535255));
#26298=CARTESIAN_POINT('Ctrl Pts',(1.68440578021706,-1.,1.02006795074201));
#26299=CARTESIAN_POINT('Ctrl Pts',(1.68440578021706,1.,1.02006795074201));
#26300=CARTESIAN_POINT('Ctrl Pts',(1.68044289894798,-1.,1.01561026162773));
#26301=CARTESIAN_POINT('Ctrl Pts',(1.68044289894798,1.,1.01561026162773));
#26302=CARTESIAN_POINT('Ctrl Pts',(1.67648246776464,-1.,1.01123236493511));
#26303=CARTESIAN_POINT('Ctrl Pts',(1.67648246776464,1.,1.01123236493511));
#26304=CARTESIAN_POINT('Ctrl Pts',(1.67250335383293,-1.,1.00692206696414));
#26305=CARTESIAN_POINT('Ctrl Pts',(1.67250335383293,1.,1.00692206696414));
#26306=CARTESIAN_POINT('Ctrl Pts',(1.66846059277303,-1.,1.00265091003727));
#26307=CARTESIAN_POINT('Ctrl Pts',(1.66846059277303,1.,1.00265091003727));
#26308=CARTESIAN_POINT('Ctrl Pts',(1.66430758030376,-1.,0.998389654952758));
#26309=CARTESIAN_POINT('Ctrl Pts',(1.66430758030376,1.,0.998389654952758));
#26310=CARTESIAN_POINT('Ctrl Pts',(1.66001553809947,-1.,0.994121836661306));
#26311=CARTESIAN_POINT('Ctrl Pts',(1.66001553809947,1.,0.994121836661306));
#26312=CARTESIAN_POINT('Ctrl Pts',(1.65559044289699,-1.,0.989855627854165));
#26313=CARTESIAN_POINT('Ctrl Pts',(1.65559044289699,1.,0.989855627854165));
#26314=CARTESIAN_POINT('Ctrl Pts',(1.65110016612638,-1.,0.985642622920821));
#26315=CARTESIAN_POINT('Ctrl Pts',(1.65110016612638,1.,0.985642622920821));
#26316=CARTESIAN_POINT('Ctrl Pts',(1.64665139190656,-1.,0.981562530939489));
#26317=CARTESIAN_POINT('Ctrl Pts',(1.64665139190656,1.,0.981562530939489));
#26318=CARTESIAN_POINT('Ctrl Pts',(1.64233990826687,-1.,0.977689794119417));
#26319=CARTESIAN_POINT('Ctrl Pts',(1.64233990826687,1.,0.977689794119417));
#26320=CARTESIAN_POINT('Ctrl Pts',(1.63820952658144,-1.,0.974066058287419));
#26321=CARTESIAN_POINT('Ctrl Pts',(1.63820952658144,1.,0.974066058287419));
#26322=CARTESIAN_POINT('Ctrl Pts',(1.63420665729798,-1.,0.970669715997509));
#26323=CARTESIAN_POINT('Ctrl Pts',(1.63420665729798,1.,0.970669715997509));
#26324=CARTESIAN_POINT('Ctrl Pts',(1.63013849959461,-1.,0.967387853230345));
#26325=CARTESIAN_POINT('Ctrl Pts',(1.63013849959461,1.,0.967387853230345));
#26326=CARTESIAN_POINT('Ctrl Pts',(1.62571930670187,-1.,0.964046107040536));
#26327=CARTESIAN_POINT('Ctrl Pts',(1.62571930670187,1.,0.964046107040536));
#26328=CARTESIAN_POINT('Ctrl Pts',(1.62061638140221,-1.,0.960438326101729));
#26329=CARTESIAN_POINT('Ctrl Pts',(1.62061638140221,1.,0.960438326101729));
#26330=CARTESIAN_POINT('Ctrl Pts',(1.61449324337085,-1.,0.956354422920671));
#26331=CARTESIAN_POINT('Ctrl Pts',(1.61449324337085,1.,0.956354422920671));
#26332=CARTESIAN_POINT('Ctrl Pts',(1.60706069896936,-1.,0.951613284356035));
#26333=CARTESIAN_POINT('Ctrl Pts',(1.60706069896936,1.,0.951613284356035));
#26334=CARTESIAN_POINT('Ctrl Pts',(1.59810042043673,-1.,0.946078063315257));
#26335=CARTESIAN_POINT('Ctrl Pts',(1.59810042043673,1.,0.946078063315257));
#26336=CARTESIAN_POINT('Ctrl Pts',(1.58744937487176,-1.,0.939646377893399));
#26337=CARTESIAN_POINT('Ctrl Pts',(1.58744937487176,1.,0.939646377893399));
#26338=CARTESIAN_POINT('Ctrl Pts',(1.57499388382243,-1.,0.932246680108685));
#26339=CARTESIAN_POINT('Ctrl Pts',(1.57499388382243,1.,0.932246680108685));
#26340=CARTESIAN_POINT('Ctrl Pts',(1.56065988578893,-1.,0.923832188944341));
#26341=CARTESIAN_POINT('Ctrl Pts',(1.56065988578893,1.,0.923832188944341));
#26342=CARTESIAN_POINT('Ctrl Pts',(1.54440491149498,-1.,0.914375919026456));
#26343=CARTESIAN_POINT('Ctrl Pts',(1.54440491149498,1.,0.914375919026456));
#26344=CARTESIAN_POINT('Ctrl Pts',(1.52984849887993,-1.,0.905967409625651));
#26345=CARTESIAN_POINT('Ctrl Pts',(1.52984849887993,1.,0.905967409625651));
#26346=CARTESIAN_POINT('Ctrl Pts',(1.51805569590094,-1.,0.899185047483511));
#26347=CARTESIAN_POINT('Ctrl Pts',(1.51805569590094,1.,0.899185047483511));
#26348=CARTESIAN_POINT('Ctrl Pts',(1.50980486806688,-1.,0.894452006964544));
#26349=CARTESIAN_POINT('Ctrl Pts',(1.50980486806688,1.,0.894452006964544));
#26350=CARTESIAN_POINT('Ctrl Pts',(1.5055822144029,-1.,0.892032620296856));
#26351=CARTESIAN_POINT('Ctrl Pts',(1.5055822144029,1.,0.892032620296856));
#26352=CARTESIAN_POINT('',(1.81978687191668,1.,1.23627494547115));
#26353=CARTESIAN_POINT('Ctrl Pts',(1.81978687191668,1.,1.23627494547115));
#26354=CARTESIAN_POINT('Ctrl Pts',(1.81925017193666,1.,1.23509651170476));
#26355=CARTESIAN_POINT('Ctrl Pts',(1.81817389921279,1.,1.2327422452705));
#26356=CARTESIAN_POINT('Ctrl Pts',(1.8165508718364,1.,1.2292186489137));
#26357=CARTESIAN_POINT('Ctrl Pts',(1.81436959210434,1.,1.2245361330495));
#26358=CARTESIAN_POINT('Ctrl Pts',(1.81161420806656,1.,1.21870906103557));
#26359=CARTESIAN_POINT('Ctrl Pts',(1.80882996917129,1.,1.21290815708314));
#26360=CARTESIAN_POINT('Ctrl Pts',(1.80601678480707,1.,1.20713356605475));
#26361=CARTESIAN_POINT('Ctrl Pts',(1.80317454838603,1.,1.20138548938974));
#26362=CARTESIAN_POINT('Ctrl Pts',(1.80030314369879,1.,1.19566418930242));
#26363=CARTESIAN_POINT('Ctrl Pts',(1.79740245923478,1.,1.18996997934445));
#26364=CARTESIAN_POINT('Ctrl Pts',(1.79447240321515,1.,1.18430321697432));
#26365=CARTESIAN_POINT('Ctrl Pts',(1.79151291552689,1.,1.17866429440809));
#26366=CARTESIAN_POINT('Ctrl Pts',(1.78852398877616,1.,1.17305363177328));
#26367=CARTESIAN_POINT('Ctrl Pts',(1.78550566040443,1.,1.16747166312303));
#26368=CARTESIAN_POINT('Ctrl Pts',(1.78245795881009,1.,1.16191881298499));
#26369=CARTESIAN_POINT('Ctrl Pts',(1.77938085564275,1.,1.15639547194698));
#26370=CARTESIAN_POINT('Ctrl Pts',(1.7762742255701,1.,1.15090197841515));
#26371=CARTESIAN_POINT('Ctrl Pts',(1.77313777896194,1.,1.1454385822692));
#26372=CARTESIAN_POINT('Ctrl Pts',(1.76997111386769,1.,1.14000548336975));
#26373=CARTESIAN_POINT('Ctrl Pts',(1.76677384551862,1.,1.1346029180462));
#26374=CARTESIAN_POINT('Ctrl Pts',(1.7635457196617,1.,1.12923123555075));
#26375=CARTESIAN_POINT('Ctrl Pts',(1.76028671825096,1.,1.12389096855086));
#26376=CARTESIAN_POINT('Ctrl Pts',(1.75699720772105,1.,1.11858293216763));
#26377=CARTESIAN_POINT('Ctrl Pts',(1.7536777209463,1.,1.11330807582551));
#26378=CARTESIAN_POINT('Ctrl Pts',(1.7503286607592,1.,1.10806728183007));
#26379=CARTESIAN_POINT('Ctrl Pts',(1.74695004214923,1.,1.10286118991143));
#26380=CARTESIAN_POINT('Ctrl Pts',(1.74354119236208,1.,1.09768999241226));
#26381=CARTESIAN_POINT('Ctrl Pts',(1.74010053962247,1.,1.09255329056493));
#26382=CARTESIAN_POINT('Ctrl Pts',(1.73662628326091,1.,1.08745056285427));
#26383=CARTESIAN_POINT('Ctrl Pts',(1.73311705663407,1.,1.08238162784749));
#26384=CARTESIAN_POINT('Ctrl Pts',(1.72957248977424,1.,1.0773470373727));
#26385=CARTESIAN_POINT('Ctrl Pts',(1.72599406198488,1.,1.07234866990252));
#26386=CARTESIAN_POINT('Ctrl Pts',(1.72238500928453,1.,1.06738966975462));
#26387=CARTESIAN_POINT('Ctrl Pts',(1.71874858456904,1.,1.06247324680647));
#26388=CARTESIAN_POINT('Ctrl Pts',(1.7150865442702,1.,1.05760163192479));
#26389=CARTESIAN_POINT('Ctrl Pts',(1.71139783543989,1.,1.05277517202855));
#26390=CARTESIAN_POINT('Ctrl Pts',(1.70767646263649,1.,1.04799085404995));
#26391=CARTESIAN_POINT('Ctrl Pts',(1.70391338707982,1.,1.04324363334554));
#26392=CARTESIAN_POINT('Ctrl Pts',(1.70010052930962,1.,1.03852922490789));
#26393=CARTESIAN_POINT('Ctrl Pts',(1.69623414782771,1.,1.03384646003588));
#26394=CARTESIAN_POINT('Ctrl Pts',(1.69231840863458,1.,1.02919977579147));
#26395=CARTESIAN_POINT('Ctrl Pts',(1.68836910178447,1.,1.02460180535255));
#26396=CARTESIAN_POINT('Ctrl Pts',(1.68440578021706,1.,1.02006795074201));
#26397=CARTESIAN_POINT('Ctrl Pts',(1.68044289894798,1.,1.01561026162773));
#26398=CARTESIAN_POINT('Ctrl Pts',(1.67648246776464,1.,1.01123236493511));
#26399=CARTESIAN_POINT('Ctrl Pts',(1.67250335383293,1.,1.00692206696414));
#26400=CARTESIAN_POINT('Ctrl Pts',(1.66846059277303,1.,1.00265091003727));
#26401=CARTESIAN_POINT('Ctrl Pts',(1.66430758030376,1.,0.998389654952758));
#26402=CARTESIAN_POINT('Ctrl Pts',(1.66001553809947,1.,0.994121836661306));
#26403=CARTESIAN_POINT('Ctrl Pts',(1.65559044289699,1.,0.989855627854165));
#26404=CARTESIAN_POINT('Ctrl Pts',(1.65110016612638,1.,0.985642622920821));
#26405=CARTESIAN_POINT('Ctrl Pts',(1.64665139190656,1.,0.981562530939489));
#26406=CARTESIAN_POINT('Ctrl Pts',(1.64233990826687,1.,0.977689794119417));
#26407=CARTESIAN_POINT('Ctrl Pts',(1.63820952658144,1.,0.974066058287419));
#26408=CARTESIAN_POINT('Ctrl Pts',(1.63420665729798,1.,0.970669715997509));
#26409=CARTESIAN_POINT('Ctrl Pts',(1.63013849959461,1.,0.967387853230345));
#26410=CARTESIAN_POINT('Ctrl Pts',(1.62571930670187,1.,0.964046107040536));
#26411=CARTESIAN_POINT('Ctrl Pts',(1.62061638140221,1.,0.960438326101729));
#26412=CARTESIAN_POINT('Ctrl Pts',(1.61449324337085,1.,0.956354422920671));
#26413=CARTESIAN_POINT('Ctrl Pts',(1.60706069896936,1.,0.951613284356035));
#26414=CARTESIAN_POINT('Ctrl Pts',(1.59810042043673,1.,0.946078063315257));
#26415=CARTESIAN_POINT('Ctrl Pts',(1.58744937487176,1.,0.939646377893399));
#26416=CARTESIAN_POINT('Ctrl Pts',(1.57499388382243,1.,0.932246680108685));
#26417=CARTESIAN_POINT('Ctrl Pts',(1.56065988578893,1.,0.923832188944341));
#26418=CARTESIAN_POINT('Ctrl Pts',(1.54440491149498,1.,0.914375919026456));
#26419=CARTESIAN_POINT('Ctrl Pts',(1.52984849887993,1.,0.905967409625651));
#26420=CARTESIAN_POINT('Ctrl Pts',(1.51805569590094,1.,0.899185047483511));
#26421=CARTESIAN_POINT('Ctrl Pts',(1.50980486806688,1.,0.894452006964544));
#26422=CARTESIAN_POINT('Ctrl Pts',(1.5055822144029,1.,0.892032620296856));
#26423=CARTESIAN_POINT('',(1.81978687191668,0.,1.23627494547115));
#26424=CARTESIAN_POINT('Origin',(1.73811241238545,0.,1.34869019493419));
#26425=CARTESIAN_POINT('',(1.73811241238545,1.,1.34869019493419));
#26426=CARTESIAN_POINT('',(1.81978687191668,1.,1.23627494547115));
#26427=CARTESIAN_POINT('',(1.73811241238545,0.,1.34869019493419));
#26428=CARTESIAN_POINT('Ctrl Pts',(1.31362392696032,-1.,1.15624053661742));
#26429=CARTESIAN_POINT('Ctrl Pts',(1.31362392696032,1.,1.15624053661742));
#26430=CARTESIAN_POINT('Ctrl Pts',(1.31722977216397,-1.,1.15950888730809));
#26431=CARTESIAN_POINT('Ctrl Pts',(1.31722977216397,1.,1.15950888730809));
#26432=CARTESIAN_POINT('Ctrl Pts',(1.32428080721772,-1.,1.16589330093588));
#26433=CARTESIAN_POINT('Ctrl Pts',(1.32428080721772,1.,1.16589330093588));
#26434=CARTESIAN_POINT('Ctrl Pts',(1.33437539347008,-1.,1.17501305789857));
#26435=CARTESIAN_POINT('Ctrl Pts',(1.33437539347008,1.,1.17501305789857));
#26436=CARTESIAN_POINT('Ctrl Pts',(1.34687054001093,-1.,1.18625865667441));
#26437=CARTESIAN_POINT('Ctrl Pts',(1.34687054001093,1.,1.18625865667441));
#26438=CARTESIAN_POINT('Ctrl Pts',(1.36088705043885,-1.,1.1987959077932));
#26439=CARTESIAN_POINT('Ctrl Pts',(1.36088705043885,1.,1.1987959077932));
#26440=CARTESIAN_POINT('Ctrl Pts',(1.37331915607905,-1.,1.20982812925645));
#26441=CARTESIAN_POINT('Ctrl Pts',(1.37331915607905,1.,1.20982812925645));
#26442=CARTESIAN_POINT('Ctrl Pts',(1.38420564527715,-1.,1.21938737280852));
#26443=CARTESIAN_POINT('Ctrl Pts',(1.38420564527715,1.,1.21938737280852));
#26444=CARTESIAN_POINT('Ctrl Pts',(1.39361389568796,-1.,1.22752961899387));
#26445=CARTESIAN_POINT('Ctrl Pts',(1.39361389568796,1.,1.22752961899387));
#26446=CARTESIAN_POINT('Ctrl Pts',(1.40164708206106,-1.,1.23434087290423));
#26447=CARTESIAN_POINT('Ctrl Pts',(1.40164708206106,1.,1.23434087290423));
#26448=CARTESIAN_POINT('Ctrl Pts',(1.40845295531283,-1.,1.23994455029534));
#26449=CARTESIAN_POINT('Ctrl Pts',(1.40845295531283,1.,1.23994455029534));
#26450=CARTESIAN_POINT('Ctrl Pts',(1.41422913175179,-1.,1.24450600513056));
#26451=CARTESIAN_POINT('Ctrl Pts',(1.41422913175179,1.,1.24450600513056));
#26452=CARTESIAN_POINT('Ctrl Pts',(1.41923722596025,-1.,1.24824430986571));
#26453=CARTESIAN_POINT('Ctrl Pts',(1.41923722596025,1.,1.24824430986571));
#26454=CARTESIAN_POINT('Ctrl Pts',(1.42378102115575,-1.,1.2514145557001));
#26455=CARTESIAN_POINT('Ctrl Pts',(1.42378102115575,1.,1.2514145557001));
#26456=CARTESIAN_POINT('Ctrl Pts',(1.42815938799387,-1.,1.25426945222639));
#26457=CARTESIAN_POINT('Ctrl Pts',(1.42815938799387,1.,1.25426945222639));
#26458=CARTESIAN_POINT('Ctrl Pts',(1.43262645609691,-1.,1.25702687965755));
#26459=CARTESIAN_POINT('Ctrl Pts',(1.43262645609691,1.,1.25702687965755));
#26460=CARTESIAN_POINT('Ctrl Pts',(1.43734919180847,-1.,1.25983531012005));
#26461=CARTESIAN_POINT('Ctrl Pts',(1.43734919180847,1.,1.25983531012005));
#26462=CARTESIAN_POINT('Ctrl Pts',(1.44236470511303,-1.,1.26273903323859));
#26463=CARTESIAN_POINT('Ctrl Pts',(1.44236470511303,1.,1.26273903323859));
#26464=CARTESIAN_POINT('Ctrl Pts',(1.44761985001662,-1.,1.26570925118868));
#26465=CARTESIAN_POINT('Ctrl Pts',(1.44761985001662,1.,1.26570925118868));
#26466=CARTESIAN_POINT('Ctrl Pts',(1.45301422764247,-1.,1.2686778680489));
#26467=CARTESIAN_POINT('Ctrl Pts',(1.45301422764247,1.,1.2686778680489));
#26468=CARTESIAN_POINT('Ctrl Pts',(1.45843906294697,-1.,1.27156805265289));
#26469=CARTESIAN_POINT('Ctrl Pts',(1.45843906294697,1.,1.27156805265289));
#26470=CARTESIAN_POINT('Ctrl Pts',(1.46382431332476,-1.,1.27433119897822));
#26471=CARTESIAN_POINT('Ctrl Pts',(1.46382431332476,1.,1.27433119897822));
#26472=CARTESIAN_POINT('Ctrl Pts',(1.46916035917133,-1.,1.2769641483109));
#26473=CARTESIAN_POINT('Ctrl Pts',(1.46916035917133,1.,1.2769641483109));
#26474=CARTESIAN_POINT('Ctrl Pts',(1.4744717526707,-1.,1.2794891824849));
#26475=CARTESIAN_POINT('Ctrl Pts',(1.4744717526707,1.,1.2794891824849));
#26476=CARTESIAN_POINT('Ctrl Pts',(1.47980070347095,-1.,1.28194158939517));
#26477=CARTESIAN_POINT('Ctrl Pts',(1.47980070347095,1.,1.28194158939517));
#26478=CARTESIAN_POINT('Ctrl Pts',(1.4851881711891,-1.,1.28435533880201));
#26479=CARTESIAN_POINT('Ctrl Pts',(1.4851881711891,1.,1.28435533880201));
#26480=CARTESIAN_POINT('Ctrl Pts',(1.4906522831278,-1.,1.2867467611644));
#26481=CARTESIAN_POINT('Ctrl Pts',(1.4906522831278,1.,1.2867467611644));
#26482=CARTESIAN_POINT('Ctrl Pts',(1.49618896881754,-1.,1.28911506584254));
#26483=CARTESIAN_POINT('Ctrl Pts',(1.49618896881754,1.,1.28911506584254));
#26484=CARTESIAN_POINT('Ctrl Pts',(1.50178230149776,-1.,1.29145022885181));
#26485=CARTESIAN_POINT('Ctrl Pts',(1.50178230149776,1.,1.29145022885181));
#26486=CARTESIAN_POINT('Ctrl Pts',(1.50741159078365,-1.,1.29373841372842));
#26487=CARTESIAN_POINT('Ctrl Pts',(1.50741159078365,1.,1.29373841372842));
#26488=CARTESIAN_POINT('Ctrl Pts',(1.51305994241402,-1.,1.29596850710509));
#26489=CARTESIAN_POINT('Ctrl Pts',(1.51305994241402,1.,1.29596850710509));
#26490=CARTESIAN_POINT('Ctrl Pts',(1.51872184912724,-1.,1.29813791800747));
#26491=CARTESIAN_POINT('Ctrl Pts',(1.51872184912724,1.,1.29813791800747));
#26492=CARTESIAN_POINT('Ctrl Pts',(1.52439957861062,-1.,1.30024984366328));
#26493=CARTESIAN_POINT('Ctrl Pts',(1.52439957861062,1.,1.30024984366328));
#26494=CARTESIAN_POINT('Ctrl Pts',(1.53009970283891,-1.,1.30231064395568));
#26495=CARTESIAN_POINT('Ctrl Pts',(1.53009970283891,1.,1.30231064395568));
#26496=CARTESIAN_POINT('Ctrl Pts',(1.53582981268977,-1.,1.30432735639489));
#26497=CARTESIAN_POINT('Ctrl Pts',(1.53582981268977,1.,1.30432735639489));
#26498=CARTESIAN_POINT('Ctrl Pts',(1.54159462645432,-1.,1.30630475189556));
#26499=CARTESIAN_POINT('Ctrl Pts',(1.54159462645432,1.,1.30630475189556));
#26500=CARTESIAN_POINT('Ctrl Pts',(1.54739413957185,-1.,1.30824393907473));
#26501=CARTESIAN_POINT('Ctrl Pts',(1.54739413957185,1.,1.30824393907473));
#26502=CARTESIAN_POINT('Ctrl Pts',(1.55322568759481,-1.,1.31014393684222));
#26503=CARTESIAN_POINT('Ctrl Pts',(1.55322568759481,1.,1.31014393684222));
#26504=CARTESIAN_POINT('Ctrl Pts',(1.55908521254821,-1.,1.31200264341696));
#26505=CARTESIAN_POINT('Ctrl Pts',(1.55908521254821,1.,1.31200264341696));
#26506=CARTESIAN_POINT('Ctrl Pts',(1.56496872402353,-1.,1.31381795281002));
#26507=CARTESIAN_POINT('Ctrl Pts',(1.56496872402353,1.,1.31381795281002));
#26508=CARTESIAN_POINT('Ctrl Pts',(1.57087397835723,-1.,1.31558903860016));
#26509=CARTESIAN_POINT('Ctrl Pts',(1.57087397835723,1.,1.31558903860016));
#26510=CARTESIAN_POINT('Ctrl Pts',(1.5768005650559,-1.,1.31731642317187));
#26511=CARTESIAN_POINT('Ctrl Pts',(1.5768005650559,1.,1.31731642317187));
#26512=CARTESIAN_POINT('Ctrl Pts',(1.58274907898834,-1.,1.31900135021432));
#26513=CARTESIAN_POINT('Ctrl Pts',(1.58274907898834,1.,1.31900135021432));
#26514=CARTESIAN_POINT('Ctrl Pts',(1.58872057258245,-1.,1.32064537110892));
#26515=CARTESIAN_POINT('Ctrl Pts',(1.58872057258245,1.,1.32064537110892));
#26516=CARTESIAN_POINT('Ctrl Pts',(1.59471591079403,-1.,1.32224985747682));
#26517=CARTESIAN_POINT('Ctrl Pts',(1.59471591079403,1.,1.32224985747682));
#26518=CARTESIAN_POINT('Ctrl Pts',(1.60073511858687,-1.,1.32381550858256));
#26519=CARTESIAN_POINT('Ctrl Pts',(1.60073511858687,1.,1.32381550858256));
#26520=CARTESIAN_POINT('Ctrl Pts',(1.60677758290954,-1.,1.32534250785782));
#26521=CARTESIAN_POINT('Ctrl Pts',(1.60677758290954,1.,1.32534250785782));
#26522=CARTESIAN_POINT('Ctrl Pts',(1.6128423401575,-1.,1.32683074483356));
#26523=CARTESIAN_POINT('Ctrl Pts',(1.6128423401575,1.,1.32683074483356));
#26524=CARTESIAN_POINT('Ctrl Pts',(1.61892832270724,-1.,1.32828000610449));
#26525=CARTESIAN_POINT('Ctrl Pts',(1.61892832270724,1.,1.32828000610449));
#26526=CARTESIAN_POINT('Ctrl Pts',(1.62503464209797,-1.,1.3296901950568));
#26527=CARTESIAN_POINT('Ctrl Pts',(1.62503464209797,1.,1.3296901950568));
#26528=CARTESIAN_POINT('Ctrl Pts',(1.63116079730923,-1.,1.33106149345645));
#26529=CARTESIAN_POINT('Ctrl Pts',(1.63116079730923,1.,1.33106149345645));
#26530=CARTESIAN_POINT('Ctrl Pts',(1.63730653475089,-1.,1.33239425103724));
#26531=CARTESIAN_POINT('Ctrl Pts',(1.63730653475089,1.,1.33239425103724));
#26532=CARTESIAN_POINT('Ctrl Pts',(1.6434717485603,-1.,1.33368890676572));
#26533=CARTESIAN_POINT('Ctrl Pts',(1.6434717485603,1.,1.33368890676572));
#26534=CARTESIAN_POINT('Ctrl Pts',(1.6496563728683,-1.,1.33494590467993));
#26535=CARTESIAN_POINT('Ctrl Pts',(1.6496563728683,1.,1.33494590467993));
#26536=CARTESIAN_POINT('Ctrl Pts',(1.65586025952593,-1.,1.33616559745172));
#26537=CARTESIAN_POINT('Ctrl Pts',(1.65586025952593,1.,1.33616559745172));
#26538=CARTESIAN_POINT('Ctrl Pts',(1.66208312541983,-1.,1.33734820885262));
#26539=CARTESIAN_POINT('Ctrl Pts',(1.66208312541983,1.,1.33734820885262));
#26540=CARTESIAN_POINT('Ctrl Pts',(1.66832460783989,-1.,1.33849388654388));
#26541=CARTESIAN_POINT('Ctrl Pts',(1.66832460783989,1.,1.33849388654388));
#26542=CARTESIAN_POINT('Ctrl Pts',(1.67458429426086,-1.,1.3396027347034));
#26543=CARTESIAN_POINT('Ctrl Pts',(1.67458429426086,1.,1.3396027347034));
#26544=CARTESIAN_POINT('Ctrl Pts',(1.68086176030362,-1.,1.34067485185203));
#26545=CARTESIAN_POINT('Ctrl Pts',(1.68086176030362,1.,1.34067485185203));
#26546=CARTESIAN_POINT('Ctrl Pts',(1.68715660868764,-1.,1.341710374848));
#26547=CARTESIAN_POINT('Ctrl Pts',(1.68715660868764,1.,1.341710374848));
#26548=CARTESIAN_POINT('Ctrl Pts',(1.6934684849687,-1.,1.34270948206319));
#26549=CARTESIAN_POINT('Ctrl Pts',(1.6934684849687,1.,1.34270948206319));
#26550=CARTESIAN_POINT('Ctrl Pts',(1.69979707754427,-1.,1.34367237124483));
#26551=CARTESIAN_POINT('Ctrl Pts',(1.69979707754427,1.,1.34367237124483));
#26552=CARTESIAN_POINT('Ctrl Pts',(1.70614212266738,-1.,1.34459924533831));
#26553=CARTESIAN_POINT('Ctrl Pts',(1.70614212266738,1.,1.34459924533831));
#26554=CARTESIAN_POINT('Ctrl Pts',(1.71250340686822,-1.,1.34549029589416));
#26555=CARTESIAN_POINT('Ctrl Pts',(1.71250340686822,1.,1.34549029589416));
#26556=CARTESIAN_POINT('Ctrl Pts',(1.7188807715049,-1.,1.34634568653227));
#26557=CARTESIAN_POINT('Ctrl Pts',(1.7188807715049,1.,1.34634568653227));
#26558=CARTESIAN_POINT('Ctrl Pts',(1.72527410680674,-1.,1.34716554819527));
#26559=CARTESIAN_POINT('Ctrl Pts',(1.72527410680674,1.,1.34716554819527));
#26560=CARTESIAN_POINT('Ctrl Pts',(1.7304014965394,-1.,1.34779309152035));
#26561=CARTESIAN_POINT('Ctrl Pts',(1.7304014965394,1.,1.34779309152035));
#26562=CARTESIAN_POINT('Ctrl Pts',(1.73425417885907,-1.,1.34824783112887));
#26563=CARTESIAN_POINT('Ctrl Pts',(1.73425417885907,1.,1.34824783112887));
#26564=CARTESIAN_POINT('Ctrl Pts',(1.73682580585691,-1.,1.34854391898045));
#26565=CARTESIAN_POINT('Ctrl Pts',(1.73682580585691,1.,1.34854391898045));
#26566=CARTESIAN_POINT('Ctrl Pts',(1.73811241238545,-1.,1.34869019493419));
#26567=CARTESIAN_POINT('Ctrl Pts',(1.73811241238545,1.,1.34869019493419));
#26568=CARTESIAN_POINT('',(1.31362392696032,1.,1.15624053661742));
#26569=CARTESIAN_POINT('Ctrl Pts',(1.31362392696032,1.,1.15624053661742));
#26570=CARTESIAN_POINT('Ctrl Pts',(1.31722977216397,1.,1.15950888730809));
#26571=CARTESIAN_POINT('Ctrl Pts',(1.32428080721772,1.,1.16589330093588));
#26572=CARTESIAN_POINT('Ctrl Pts',(1.33437539347008,1.,1.17501305789857));
#26573=CARTESIAN_POINT('Ctrl Pts',(1.34687054001093,1.,1.18625865667441));
#26574=CARTESIAN_POINT('Ctrl Pts',(1.36088705043885,1.,1.1987959077932));
#26575=CARTESIAN_POINT('Ctrl Pts',(1.37331915607905,1.,1.20982812925645));
#26576=CARTESIAN_POINT('Ctrl Pts',(1.38420564527715,1.,1.21938737280852));
#26577=CARTESIAN_POINT('Ctrl Pts',(1.39361389568796,1.,1.22752961899387));
#26578=CARTESIAN_POINT('Ctrl Pts',(1.40164708206106,1.,1.23434087290423));
#26579=CARTESIAN_POINT('Ctrl Pts',(1.40845295531283,1.,1.23994455029534));
#26580=CARTESIAN_POINT('Ctrl Pts',(1.41422913175179,1.,1.24450600513056));
#26581=CARTESIAN_POINT('Ctrl Pts',(1.41923722596025,1.,1.24824430986571));
#26582=CARTESIAN_POINT('Ctrl Pts',(1.42378102115575,1.,1.2514145557001));
#26583=CARTESIAN_POINT('Ctrl Pts',(1.42815938799387,1.,1.25426945222639));
#26584=CARTESIAN_POINT('Ctrl Pts',(1.43262645609691,1.,1.25702687965755));
#26585=CARTESIAN_POINT('Ctrl Pts',(1.43734919180847,1.,1.25983531012005));
#26586=CARTESIAN_POINT('Ctrl Pts',(1.44236470511303,1.,1.26273903323859));
#26587=CARTESIAN_POINT('Ctrl Pts',(1.44761985001662,1.,1.26570925118868));
#26588=CARTESIAN_POINT('Ctrl Pts',(1.45301422764247,1.,1.2686778680489));
#26589=CARTESIAN_POINT('Ctrl Pts',(1.45843906294697,1.,1.27156805265289));
#26590=CARTESIAN_POINT('Ctrl Pts',(1.46382431332476,1.,1.27433119897822));
#26591=CARTESIAN_POINT('Ctrl Pts',(1.46916035917133,1.,1.2769641483109));
#26592=CARTESIAN_POINT('Ctrl Pts',(1.4744717526707,1.,1.2794891824849));
#26593=CARTESIAN_POINT('Ctrl Pts',(1.47980070347095,1.,1.28194158939517));
#26594=CARTESIAN_POINT('Ctrl Pts',(1.4851881711891,1.,1.28435533880201));
#26595=CARTESIAN_POINT('Ctrl Pts',(1.4906522831278,1.,1.2867467611644));
#26596=CARTESIAN_POINT('Ctrl Pts',(1.49618896881754,1.,1.28911506584254));
#26597=CARTESIAN_POINT('Ctrl Pts',(1.50178230149776,1.,1.29145022885181));
#26598=CARTESIAN_POINT('Ctrl Pts',(1.50741159078365,1.,1.29373841372842));
#26599=CARTESIAN_POINT('Ctrl Pts',(1.51305994241402,1.,1.29596850710509));
#26600=CARTESIAN_POINT('Ctrl Pts',(1.51872184912724,1.,1.29813791800747));
#26601=CARTESIAN_POINT('Ctrl Pts',(1.52439957861062,1.,1.30024984366328));
#26602=CARTESIAN_POINT('Ctrl Pts',(1.53009970283891,1.,1.30231064395568));
#26603=CARTESIAN_POINT('Ctrl Pts',(1.53582981268977,1.,1.30432735639489));
#26604=CARTESIAN_POINT('Ctrl Pts',(1.54159462645432,1.,1.30630475189556));
#26605=CARTESIAN_POINT('Ctrl Pts',(1.54739413957185,1.,1.30824393907473));
#26606=CARTESIAN_POINT('Ctrl Pts',(1.55322568759481,1.,1.31014393684222));
#26607=CARTESIAN_POINT('Ctrl Pts',(1.55908521254821,1.,1.31200264341696));
#26608=CARTESIAN_POINT('Ctrl Pts',(1.56496872402353,1.,1.31381795281002));
#26609=CARTESIAN_POINT('Ctrl Pts',(1.57087397835723,1.,1.31558903860016));
#26610=CARTESIAN_POINT('Ctrl Pts',(1.5768005650559,1.,1.31731642317187));
#26611=CARTESIAN_POINT('Ctrl Pts',(1.58274907898834,1.,1.31900135021432));
#26612=CARTESIAN_POINT('Ctrl Pts',(1.58872057258245,1.,1.32064537110892));
#26613=CARTESIAN_POINT('Ctrl Pts',(1.59471591079403,1.,1.32224985747682));
#26614=CARTESIAN_POINT('Ctrl Pts',(1.60073511858687,1.,1.32381550858256));
#26615=CARTESIAN_POINT('Ctrl Pts',(1.60677758290954,1.,1.32534250785782));
#26616=CARTESIAN_POINT('Ctrl Pts',(1.6128423401575,1.,1.32683074483356));
#26617=CARTESIAN_POINT('Ctrl Pts',(1.61892832270724,1.,1.32828000610449));
#26618=CARTESIAN_POINT('Ctrl Pts',(1.62503464209797,1.,1.3296901950568));
#26619=CARTESIAN_POINT('Ctrl Pts',(1.63116079730923,1.,1.33106149345645));
#26620=CARTESIAN_POINT('Ctrl Pts',(1.63730653475089,1.,1.33239425103724));
#26621=CARTESIAN_POINT('Ctrl Pts',(1.6434717485603,1.,1.33368890676572));
#26622=CARTESIAN_POINT('Ctrl Pts',(1.6496563728683,1.,1.33494590467993));
#26623=CARTESIAN_POINT('Ctrl Pts',(1.65586025952593,1.,1.33616559745172));
#26624=CARTESIAN_POINT('Ctrl Pts',(1.66208312541983,1.,1.33734820885262));
#26625=CARTESIAN_POINT('Ctrl Pts',(1.66832460783989,1.,1.33849388654388));
#26626=CARTESIAN_POINT('Ctrl Pts',(1.67458429426086,1.,1.3396027347034));
#26627=CARTESIAN_POINT('Ctrl Pts',(1.68086176030362,1.,1.34067485185203));
#26628=CARTESIAN_POINT('Ctrl Pts',(1.68715660868764,1.,1.341710374848));
#26629=CARTESIAN_POINT('Ctrl Pts',(1.6934684849687,1.,1.34270948206319));
#26630=CARTESIAN_POINT('Ctrl Pts',(1.69979707754427,1.,1.34367237124483));
#26631=CARTESIAN_POINT('Ctrl Pts',(1.70614212266738,1.,1.34459924533831));
#26632=CARTESIAN_POINT('Ctrl Pts',(1.71250340686822,1.,1.34549029589416));
#26633=CARTESIAN_POINT('Ctrl Pts',(1.7188807715049,1.,1.34634568653227));
#26634=CARTESIAN_POINT('Ctrl Pts',(1.72527410680674,1.,1.34716554819527));
#26635=CARTESIAN_POINT('Ctrl Pts',(1.7304014965394,1.,1.34779309152035));
#26636=CARTESIAN_POINT('Ctrl Pts',(1.73425417885907,1.,1.34824783112887));
#26637=CARTESIAN_POINT('Ctrl Pts',(1.73682580585691,1.,1.34854391898045));
#26638=CARTESIAN_POINT('Ctrl Pts',(1.73811241238545,1.,1.34869019493419));
#26639=CARTESIAN_POINT('',(1.31362392696032,0.,1.15624053661742));
#26640=CARTESIAN_POINT('Origin',(0.,0.,0.));
#26641=CARTESIAN_POINT('',(1.15624053661742,1.,1.31362392696033));
#26642=CARTESIAN_POINT('Origin',(0.,1.,0.));
#26643=CARTESIAN_POINT('',(1.15624053661742,0.,1.31362392696032));
#26644=CARTESIAN_POINT('Ctrl Pts',(1.34869019493419,-1.,1.73811241238545));
#26645=CARTESIAN_POINT('Ctrl Pts',(1.34869019493419,1.,1.73811241238545));
#26646=CARTESIAN_POINT('Ctrl Pts',(1.34854391898145,-1.,1.73682580585819));
#26647=CARTESIAN_POINT('Ctrl Pts',(1.34854391898145,1.,1.73682580585819));
#26648=CARTESIAN_POINT('Ctrl Pts',(1.34824783113158,-1.,1.73425417886255));
#26649=CARTESIAN_POINT('Ctrl Pts',(1.34824783113158,1.,1.73425417886255));
#26650=CARTESIAN_POINT('Ctrl Pts',(1.3477930915247,-1.,1.73040149654497));
#26651=CARTESIAN_POINT('Ctrl Pts',(1.3477930915247,1.,1.73040149654497));
#26652=CARTESIAN_POINT('Ctrl Pts',(1.34716554820013,-1.,1.72527410681298));
#26653=CARTESIAN_POINT('Ctrl Pts',(1.34716554820013,1.,1.72527410681298));
#26654=CARTESIAN_POINT('Ctrl Pts',(1.34634568653586,-1.,1.7188807715095));
#26655=CARTESIAN_POINT('Ctrl Pts',(1.34634568653586,1.,1.7188807715095));
#26656=CARTESIAN_POINT('Ctrl Pts',(1.34549029589563,-1.,1.71250340687011));
#26657=CARTESIAN_POINT('Ctrl Pts',(1.34549029589563,1.,1.71250340687011));
#26658=CARTESIAN_POINT('Ctrl Pts',(1.34459924533783,-1.,1.70614212266676));
#26659=CARTESIAN_POINT('Ctrl Pts',(1.34459924533783,1.,1.70614212266676));
#26660=CARTESIAN_POINT('Ctrl Pts',(1.34367237124322,-1.,1.69979707754221));
#26661=CARTESIAN_POINT('Ctrl Pts',(1.34367237124322,1.,1.69979707754221));
#26662=CARTESIAN_POINT('Ctrl Pts',(1.34270948206139,-1.,1.6934684849664));
#26663=CARTESIAN_POINT('Ctrl Pts',(1.34270948206139,1.,1.6934684849664));
#26664=CARTESIAN_POINT('Ctrl Pts',(1.34171037484673,-1.,1.68715660868602));
#26665=CARTESIAN_POINT('Ctrl Pts',(1.34171037484673,1.,1.68715660868602));
#26666=CARTESIAN_POINT('Ctrl Pts',(1.3406748518516,-1.,1.68086176030308));
#26667=CARTESIAN_POINT('Ctrl Pts',(1.3406748518516,1.,1.68086176030308));
#26668=CARTESIAN_POINT('Ctrl Pts',(1.33960273470372,-1.,1.67458429426126));
#26669=CARTESIAN_POINT('Ctrl Pts',(1.33960273470372,1.,1.67458429426126));
#26670=CARTESIAN_POINT('Ctrl Pts',(1.33849388654458,-1.,1.66832460784078));
#26671=CARTESIAN_POINT('Ctrl Pts',(1.33849388654458,1.,1.66832460784078));
#26672=CARTESIAN_POINT('Ctrl Pts',(1.33734820885331,-1.,1.66208312542073));
#26673=CARTESIAN_POINT('Ctrl Pts',(1.33734820885331,1.,1.66208312542073));
#26674=CARTESIAN_POINT('Ctrl Pts',(1.33616559745217,-1.,1.65586025952651));
#26675=CARTESIAN_POINT('Ctrl Pts',(1.33616559745217,1.,1.65586025952651));
#26676=CARTESIAN_POINT('Ctrl Pts',(1.33494590468003,-1.,1.64965637286843));
#26677=CARTESIAN_POINT('Ctrl Pts',(1.33494590468003,1.,1.64965637286843));
#26678=CARTESIAN_POINT('Ctrl Pts',(1.33368890676554,-1.,1.64347174856007));
#26679=CARTESIAN_POINT('Ctrl Pts',(1.33368890676554,1.,1.64347174856007));
#26680=CARTESIAN_POINT('Ctrl Pts',(1.33239425103694,-1.,1.6373065347505));
#26681=CARTESIAN_POINT('Ctrl Pts',(1.33239425103694,1.,1.6373065347505));
#26682=CARTESIAN_POINT('Ctrl Pts',(1.33106149345618,-1.,1.63116079730887));
#26683=CARTESIAN_POINT('Ctrl Pts',(1.33106149345618,1.,1.63116079730887));
#26684=CARTESIAN_POINT('Ctrl Pts',(1.32969019505665,-1.,1.62503464209777));
#26685=CARTESIAN_POINT('Ctrl Pts',(1.32969019505665,1.,1.62503464209777));
#26686=CARTESIAN_POINT('Ctrl Pts',(1.32828000610448,-1.,1.61892832270723));
#26687=CARTESIAN_POINT('Ctrl Pts',(1.32828000610448,1.,1.61892832270723));
#26688=CARTESIAN_POINT('Ctrl Pts',(1.32683074483365,-1.,1.61284234015762));
#26689=CARTESIAN_POINT('Ctrl Pts',(1.32683074483365,1.,1.61284234015762));
#26690=CARTESIAN_POINT('Ctrl Pts',(1.32534250785794,-1.,1.6067775829097));
#26691=CARTESIAN_POINT('Ctrl Pts',(1.32534250785794,1.,1.6067775829097));
#26692=CARTESIAN_POINT('Ctrl Pts',(1.32381550858266,-1.,1.600735118587));
#26693=CARTESIAN_POINT('Ctrl Pts',(1.32381550858266,1.,1.600735118587));
#26694=CARTESIAN_POINT('Ctrl Pts',(1.32224985747686,-1.,1.59471591079408));
#26695=CARTESIAN_POINT('Ctrl Pts',(1.32224985747686,1.,1.59471591079408));
#26696=CARTESIAN_POINT('Ctrl Pts',(1.32064537110891,-1.,1.58872057258244));
#26697=CARTESIAN_POINT('Ctrl Pts',(1.32064537110891,1.,1.58872057258244));
#26698=CARTESIAN_POINT('Ctrl Pts',(1.31900135021428,-1.,1.58274907898829));
#26699=CARTESIAN_POINT('Ctrl Pts',(1.31900135021428,1.,1.58274907898829));
#26700=CARTESIAN_POINT('Ctrl Pts',(1.31731642317183,-1.,1.57680056505585));
#26701=CARTESIAN_POINT('Ctrl Pts',(1.31731642317183,1.,1.57680056505585));
#26702=CARTESIAN_POINT('Ctrl Pts',(1.31558903860015,-1.,1.57087397835721));
#26703=CARTESIAN_POINT('Ctrl Pts',(1.31558903860015,1.,1.57087397835721));
#26704=CARTESIAN_POINT('Ctrl Pts',(1.31381795281002,-1.,1.56496872402352));
#26705=CARTESIAN_POINT('Ctrl Pts',(1.31381795281002,1.,1.56496872402352));
#26706=CARTESIAN_POINT('Ctrl Pts',(1.31200264341696,-1.,1.55908521254822));
#26707=CARTESIAN_POINT('Ctrl Pts',(1.31200264341696,1.,1.55908521254822));
#26708=CARTESIAN_POINT('Ctrl Pts',(1.31014393684221,-1.,1.55322568759481));
#26709=CARTESIAN_POINT('Ctrl Pts',(1.31014393684221,1.,1.55322568759481));
#26710=CARTESIAN_POINT('Ctrl Pts',(1.30824393907471,-1.,1.54739413957183));
#26711=CARTESIAN_POINT('Ctrl Pts',(1.30824393907471,1.,1.54739413957183));
#26712=CARTESIAN_POINT('Ctrl Pts',(1.30630475189553,-1.,1.54159462645428));
#26713=CARTESIAN_POINT('Ctrl Pts',(1.30630475189553,1.,1.54159462645428));
#26714=CARTESIAN_POINT('Ctrl Pts',(1.30432735639487,-1.,1.53582981268976));
#26715=CARTESIAN_POINT('Ctrl Pts',(1.30432735639487,1.,1.53582981268976));
#26716=CARTESIAN_POINT('Ctrl Pts',(1.3023106439557,-1.,1.53009970283893));
#26717=CARTESIAN_POINT('Ctrl Pts',(1.3023106439557,1.,1.53009970283893));
#26718=CARTESIAN_POINT('Ctrl Pts',(1.30024984366334,-1.,1.5243995786107));
#26719=CARTESIAN_POINT('Ctrl Pts',(1.30024984366334,1.,1.5243995786107));
#26720=CARTESIAN_POINT('Ctrl Pts',(1.29813791800757,-1.,1.51872184912735));
#26721=CARTESIAN_POINT('Ctrl Pts',(1.29813791800757,1.,1.51872184912735));
#26722=CARTESIAN_POINT('Ctrl Pts',(1.29596850710518,-1.,1.51305994241412));
#26723=CARTESIAN_POINT('Ctrl Pts',(1.29596850710518,1.,1.51305994241412));
#26724=CARTESIAN_POINT('Ctrl Pts',(1.29373841372843,-1.,1.50741159078367));
#26725=CARTESIAN_POINT('Ctrl Pts',(1.29373841372843,1.,1.50741159078367));
#26726=CARTESIAN_POINT('Ctrl Pts',(1.29145022885171,-1.,1.50178230149764));
#26727=CARTESIAN_POINT('Ctrl Pts',(1.29145022885171,1.,1.50178230149764));
#26728=CARTESIAN_POINT('Ctrl Pts',(1.28911506584232,-1.,1.49618896881729));
#26729=CARTESIAN_POINT('Ctrl Pts',(1.28911506584232,1.,1.49618896881729));
#26730=CARTESIAN_POINT('Ctrl Pts',(1.28674676116415,-1.,1.4906522831275));
#26731=CARTESIAN_POINT('Ctrl Pts',(1.28674676116415,1.,1.4906522831275));
#26732=CARTESIAN_POINT('Ctrl Pts',(1.28435533880184,-1.,1.48518817118891));
#26733=CARTESIAN_POINT('Ctrl Pts',(1.28435533880184,1.,1.48518817118891));
#26734=CARTESIAN_POINT('Ctrl Pts',(1.28194158939522,-1.,1.47980070347102));
#26735=CARTESIAN_POINT('Ctrl Pts',(1.28194158939522,1.,1.47980070347102));
#26736=CARTESIAN_POINT('Ctrl Pts',(1.27948918248524,-1.,1.4744717526711));
#26737=CARTESIAN_POINT('Ctrl Pts',(1.27948918248524,1.,1.4744717526711));
#26738=CARTESIAN_POINT('Ctrl Pts',(1.27696414831144,-1.,1.46916035917197));
#26739=CARTESIAN_POINT('Ctrl Pts',(1.27696414831144,1.,1.46916035917197));
#26740=CARTESIAN_POINT('Ctrl Pts',(1.27433119897877,-1.,1.4638243133254));
#26741=CARTESIAN_POINT('Ctrl Pts',(1.27433119897877,1.,1.4638243133254));
#26742=CARTESIAN_POINT('Ctrl Pts',(1.27156805265312,-1.,1.45843906294725));
#26743=CARTESIAN_POINT('Ctrl Pts',(1.27156805265312,1.,1.45843906294725));
#26744=CARTESIAN_POINT('Ctrl Pts',(1.26867786804854,-1.,1.45301422764205));
#26745=CARTESIAN_POINT('Ctrl Pts',(1.26867786804854,1.,1.45301422764205));
#26746=CARTESIAN_POINT('Ctrl Pts',(1.26570925118767,-1.,1.44761985001544));
#26747=CARTESIAN_POINT('Ctrl Pts',(1.26570925118767,1.,1.44761985001544));
#26748=CARTESIAN_POINT('Ctrl Pts',(1.26273903323723,-1.,1.44236470511145));
#26749=CARTESIAN_POINT('Ctrl Pts',(1.26273903323723,1.,1.44236470511145));
#26750=CARTESIAN_POINT('Ctrl Pts',(1.25983531011894,-1.,1.43734919180719));
#26751=CARTESIAN_POINT('Ctrl Pts',(1.25983531011894,1.,1.43734919180719));
#26752=CARTESIAN_POINT('Ctrl Pts',(1.25702687965744,-1.,1.43262645609679));
#26753=CARTESIAN_POINT('Ctrl Pts',(1.25702687965744,1.,1.43262645609679));
#26754=CARTESIAN_POINT('Ctrl Pts',(1.25426945222783,-1.,1.42815938799555));
#26755=CARTESIAN_POINT('Ctrl Pts',(1.25426945222783,1.,1.42815938799555));
#26756=CARTESIAN_POINT('Ctrl Pts',(1.25141455570299,-1.,1.42378102115911));
#26757=CARTESIAN_POINT('Ctrl Pts',(1.25141455570299,1.,1.42378102115911));
#26758=CARTESIAN_POINT('Ctrl Pts',(1.24824430986911,-1.,1.41923722596421));
#26759=CARTESIAN_POINT('Ctrl Pts',(1.24824430986911,1.,1.41923722596421));
#26760=CARTESIAN_POINT('Ctrl Pts',(1.24450600513278,-1.,1.41422913175437));
#26761=CARTESIAN_POINT('Ctrl Pts',(1.24450600513278,1.,1.41422913175437));
#26762=CARTESIAN_POINT('Ctrl Pts',(1.23994455029421,-1.,1.40845295531151));
#26763=CARTESIAN_POINT('Ctrl Pts',(1.23994455029421,1.,1.40845295531151));
#26764=CARTESIAN_POINT('Ctrl Pts',(1.23434087289768,-1.,1.40164708205345));
#26765=CARTESIAN_POINT('Ctrl Pts',(1.23434087289768,1.,1.40164708205345));
#26766=CARTESIAN_POINT('Ctrl Pts',(1.22752961898063,-1.,1.39361389567257));
#26767=CARTESIAN_POINT('Ctrl Pts',(1.22752961898063,1.,1.39361389567257));
#26768=CARTESIAN_POINT('Ctrl Pts',(1.21938737278853,-1.,1.38420564525391));
#26769=CARTESIAN_POINT('Ctrl Pts',(1.21938737278853,1.,1.38420564525391));
#26770=CARTESIAN_POINT('Ctrl Pts',(1.20982812923113,-1.,1.37331915604962));
#26771=CARTESIAN_POINT('Ctrl Pts',(1.20982812923113,1.,1.37331915604962));
#26772=CARTESIAN_POINT('Ctrl Pts',(1.1987959077656,-1.,1.36088705040677));
#26773=CARTESIAN_POINT('Ctrl Pts',(1.1987959077656,1.,1.36088705040677));
#26774=CARTESIAN_POINT('Ctrl Pts',(1.18625865664915,-1.,1.34687053998157));
#26775=CARTESIAN_POINT('Ctrl Pts',(1.18625865664915,1.,1.34687053998157));
#26776=CARTESIAN_POINT('Ctrl Pts',(1.17501305787994,-1.,1.33437539344842));
#26777=CARTESIAN_POINT('Ctrl Pts',(1.17501305787994,1.,1.33437539344842));
#26778=CARTESIAN_POINT('Ctrl Pts',(1.16589330092532,-1.,1.32428080720544));
#26779=CARTESIAN_POINT('Ctrl Pts',(1.16589330092532,1.,1.32428080720544));
#26780=CARTESIAN_POINT('Ctrl Pts',(1.15950888730433,-1.,1.3172297721596));
#26781=CARTESIAN_POINT('Ctrl Pts',(1.15950888730433,1.,1.3172297721596));
#26782=CARTESIAN_POINT('Ctrl Pts',(1.15624053661742,-1.,1.31362392696033));
#26783=CARTESIAN_POINT('Ctrl Pts',(1.15624053661742,1.,1.31362392696033));
#26784=CARTESIAN_POINT('',(1.34869019493419,1.,1.73811241238545));
#26785=CARTESIAN_POINT('Ctrl Pts',(1.34869019493419,1.,1.73811241238545));
#26786=CARTESIAN_POINT('Ctrl Pts',(1.34854391898145,1.,1.73682580585819));
#26787=CARTESIAN_POINT('Ctrl Pts',(1.34824783113158,1.,1.73425417886255));
#26788=CARTESIAN_POINT('Ctrl Pts',(1.3477930915247,1.,1.73040149654497));
#26789=CARTESIAN_POINT('Ctrl Pts',(1.34716554820013,1.,1.72527410681298));
#26790=CARTESIAN_POINT('Ctrl Pts',(1.34634568653586,1.,1.7188807715095));
#26791=CARTESIAN_POINT('Ctrl Pts',(1.34549029589563,1.,1.71250340687011));
#26792=CARTESIAN_POINT('Ctrl Pts',(1.34459924533783,1.,1.70614212266676));
#26793=CARTESIAN_POINT('Ctrl Pts',(1.34367237124322,1.,1.69979707754221));
#26794=CARTESIAN_POINT('Ctrl Pts',(1.34270948206139,1.,1.6934684849664));
#26795=CARTESIAN_POINT('Ctrl Pts',(1.34171037484673,1.,1.68715660868602));
#26796=CARTESIAN_POINT('Ctrl Pts',(1.3406748518516,1.,1.68086176030308));
#26797=CARTESIAN_POINT('Ctrl Pts',(1.33960273470372,1.,1.67458429426126));
#26798=CARTESIAN_POINT('Ctrl Pts',(1.33849388654458,1.,1.66832460784078));
#26799=CARTESIAN_POINT('Ctrl Pts',(1.33734820885331,1.,1.66208312542073));
#26800=CARTESIAN_POINT('Ctrl Pts',(1.33616559745217,1.,1.65586025952651));
#26801=CARTESIAN_POINT('Ctrl Pts',(1.33494590468003,1.,1.64965637286843));
#26802=CARTESIAN_POINT('Ctrl Pts',(1.33368890676554,1.,1.64347174856007));
#26803=CARTESIAN_POINT('Ctrl Pts',(1.33239425103694,1.,1.6373065347505));
#26804=CARTESIAN_POINT('Ctrl Pts',(1.33106149345618,1.,1.63116079730887));
#26805=CARTESIAN_POINT('Ctrl Pts',(1.32969019505665,1.,1.62503464209777));
#26806=CARTESIAN_POINT('Ctrl Pts',(1.32828000610448,1.,1.61892832270723));
#26807=CARTESIAN_POINT('Ctrl Pts',(1.32683074483365,1.,1.61284234015762));
#26808=CARTESIAN_POINT('Ctrl Pts',(1.32534250785794,1.,1.6067775829097));
#26809=CARTESIAN_POINT('Ctrl Pts',(1.32381550858266,1.,1.600735118587));
#26810=CARTESIAN_POINT('Ctrl Pts',(1.32224985747686,1.,1.59471591079408));
#26811=CARTESIAN_POINT('Ctrl Pts',(1.32064537110891,1.,1.58872057258244));
#26812=CARTESIAN_POINT('Ctrl Pts',(1.31900135021428,1.,1.58274907898829));
#26813=CARTESIAN_POINT('Ctrl Pts',(1.31731642317183,1.,1.57680056505585));
#26814=CARTESIAN_POINT('Ctrl Pts',(1.31558903860015,1.,1.57087397835721));
#26815=CARTESIAN_POINT('Ctrl Pts',(1.31381795281002,1.,1.56496872402352));
#26816=CARTESIAN_POINT('Ctrl Pts',(1.31200264341696,1.,1.55908521254822));
#26817=CARTESIAN_POINT('Ctrl Pts',(1.31014393684221,1.,1.55322568759481));
#26818=CARTESIAN_POINT('Ctrl Pts',(1.30824393907471,1.,1.54739413957183));
#26819=CARTESIAN_POINT('Ctrl Pts',(1.30630475189553,1.,1.54159462645428));
#26820=CARTESIAN_POINT('Ctrl Pts',(1.30432735639487,1.,1.53582981268976));
#26821=CARTESIAN_POINT('Ctrl Pts',(1.3023106439557,1.,1.53009970283893));
#26822=CARTESIAN_POINT('Ctrl Pts',(1.30024984366334,1.,1.5243995786107));
#26823=CARTESIAN_POINT('Ctrl Pts',(1.29813791800757,1.,1.51872184912735));
#26824=CARTESIAN_POINT('Ctrl Pts',(1.29596850710518,1.,1.51305994241412));
#26825=CARTESIAN_POINT('Ctrl Pts',(1.29373841372843,1.,1.50741159078367));
#26826=CARTESIAN_POINT('Ctrl Pts',(1.29145022885171,1.,1.50178230149764));
#26827=CARTESIAN_POINT('Ctrl Pts',(1.28911506584232,1.,1.49618896881729));
#26828=CARTESIAN_POINT('Ctrl Pts',(1.28674676116415,1.,1.4906522831275));
#26829=CARTESIAN_POINT('Ctrl Pts',(1.28435533880184,1.,1.48518817118891));
#26830=CARTESIAN_POINT('Ctrl Pts',(1.28194158939522,1.,1.47980070347102));
#26831=CARTESIAN_POINT('Ctrl Pts',(1.27948918248524,1.,1.4744717526711));
#26832=CARTESIAN_POINT('Ctrl Pts',(1.27696414831144,1.,1.46916035917197));
#26833=CARTESIAN_POINT('Ctrl Pts',(1.27433119897877,1.,1.4638243133254));
#26834=CARTESIAN_POINT('Ctrl Pts',(1.27156805265312,1.,1.45843906294725));
#26835=CARTESIAN_POINT('Ctrl Pts',(1.26867786804854,1.,1.45301422764205));
#26836=CARTESIAN_POINT('Ctrl Pts',(1.26570925118767,1.,1.44761985001544));
#26837=CARTESIAN_POINT('Ctrl Pts',(1.26273903323723,1.,1.44236470511145));
#26838=CARTESIAN_POINT('Ctrl Pts',(1.25983531011894,1.,1.43734919180719));
#26839=CARTESIAN_POINT('Ctrl Pts',(1.25702687965744,1.,1.43262645609679));
#26840=CARTESIAN_POINT('Ctrl Pts',(1.25426945222783,1.,1.42815938799555));
#26841=CARTESIAN_POINT('Ctrl Pts',(1.25141455570299,1.,1.42378102115911));
#26842=CARTESIAN_POINT('Ctrl Pts',(1.24824430986911,1.,1.41923722596421));
#26843=CARTESIAN_POINT('Ctrl Pts',(1.24450600513278,1.,1.41422913175437));
#26844=CARTESIAN_POINT('Ctrl Pts',(1.23994455029421,1.,1.40845295531151));
#26845=CARTESIAN_POINT('Ctrl Pts',(1.23434087289768,1.,1.40164708205345));
#26846=CARTESIAN_POINT('Ctrl Pts',(1.22752961898063,1.,1.39361389567257));
#26847=CARTESIAN_POINT('Ctrl Pts',(1.21938737278853,1.,1.38420564525391));
#26848=CARTESIAN_POINT('Ctrl Pts',(1.20982812923113,1.,1.37331915604962));
#26849=CARTESIAN_POINT('Ctrl Pts',(1.1987959077656,1.,1.36088705040677));
#26850=CARTESIAN_POINT('Ctrl Pts',(1.18625865664915,1.,1.34687053998157));
#26851=CARTESIAN_POINT('Ctrl Pts',(1.17501305787994,1.,1.33437539344842));
#26852=CARTESIAN_POINT('Ctrl Pts',(1.16589330092532,1.,1.32428080720544));
#26853=CARTESIAN_POINT('Ctrl Pts',(1.15950888730433,1.,1.3172297721596));
#26854=CARTESIAN_POINT('Ctrl Pts',(1.15624053661742,1.,1.31362392696033));
#26855=CARTESIAN_POINT('',(1.34869019493419,0.,1.73811241238545));
#26856=CARTESIAN_POINT('Origin',(1.23627494547115,0.,1.81978687191668));
#26857=CARTESIAN_POINT('',(1.23627494547115,1.,1.81978687191668));
#26858=CARTESIAN_POINT('',(1.34869019493419,1.,1.73811241238545));
#26859=CARTESIAN_POINT('',(1.23627494547115,0.,1.81978687191668));
#26860=CARTESIAN_POINT('Ctrl Pts',(0.892032620296855,-1.,1.5055822144029));
#26861=CARTESIAN_POINT('Ctrl Pts',(0.892032620296855,1.,1.5055822144029));
#26862=CARTESIAN_POINT('Ctrl Pts',(0.894452006967538,-1.,1.50980486807181));
#26863=CARTESIAN_POINT('Ctrl Pts',(0.894452006967538,1.,1.50980486807181));
#26864=CARTESIAN_POINT('Ctrl Pts',(0.89918504749193,-1.,1.51805569591479));
#26865=CARTESIAN_POINT('Ctrl Pts',(0.89918504749193,1.,1.51805569591479));
#26866=CARTESIAN_POINT('Ctrl Pts',(0.905967409640498,-1.,1.52984849890434));
#26867=CARTESIAN_POINT('Ctrl Pts',(0.905967409640498,1.,1.52984849890434));
#26868=CARTESIAN_POINT('Ctrl Pts',(0.914375919046579,-1.,1.54440491152808));
#26869=CARTESIAN_POINT('Ctrl Pts',(0.914375919046579,1.,1.54440491152808));
#26870=CARTESIAN_POINT('Ctrl Pts',(0.923832188966322,-1.,1.56065988582509));
#26871=CARTESIAN_POINT('Ctrl Pts',(0.923832188966322,1.,1.56065988582509));
#26872=CARTESIAN_POINT('Ctrl Pts',(0.932246680128848,-1.,1.57499388385561));
#26873=CARTESIAN_POINT('Ctrl Pts',(0.932246680128848,1.,1.57499388385561));
#26874=CARTESIAN_POINT('Ctrl Pts',(0.939646377909319,-1.,1.58744937489796));
#26875=CARTESIAN_POINT('Ctrl Pts',(0.939646377909319,1.,1.58744937489796));
#26876=CARTESIAN_POINT('Ctrl Pts',(0.946078063325795,-1.,1.59810042045408));
#26877=CARTESIAN_POINT('Ctrl Pts',(0.946078063325795,1.,1.59810042045408));
#26878=CARTESIAN_POINT('Ctrl Pts',(0.951613284361247,-1.,1.60706069897794));
#26879=CARTESIAN_POINT('Ctrl Pts',(0.951613284361247,1.,1.60706069897794));
#26880=CARTESIAN_POINT('Ctrl Pts',(0.956354422921572,-1.,1.61449324337233));
#26881=CARTESIAN_POINT('Ctrl Pts',(0.956354422921572,1.,1.61449324337233));
#26882=CARTESIAN_POINT('Ctrl Pts',(0.960438326099958,-1.,1.62061638139929));
#26883=CARTESIAN_POINT('Ctrl Pts',(0.960438326099958,1.,1.62061638139929));
#26884=CARTESIAN_POINT('Ctrl Pts',(0.964046107037821,-1.,1.6257193066974));
#26885=CARTESIAN_POINT('Ctrl Pts',(0.964046107037821,1.,1.6257193066974));
#26886=CARTESIAN_POINT('Ctrl Pts',(0.967387853228041,-1.,1.63013849959083));
#26887=CARTESIAN_POINT('Ctrl Pts',(0.967387853228041,1.,1.63013849959083));
#26888=CARTESIAN_POINT('Ctrl Pts',(0.970669715996356,-1.,1.63420665729609));
#26889=CARTESIAN_POINT('Ctrl Pts',(0.970669715996356,1.,1.63420665729609));
#26890=CARTESIAN_POINT('Ctrl Pts',(0.974066058287501,-1.,1.63820952658157));
#26891=CARTESIAN_POINT('Ctrl Pts',(0.974066058287501,1.,1.63820952658157));
#26892=CARTESIAN_POINT('Ctrl Pts',(0.977689794120296,-1.,1.64233990826831));
#26893=CARTESIAN_POINT('Ctrl Pts',(0.977689794120296,1.,1.64233990826831));
#26894=CARTESIAN_POINT('Ctrl Pts',(0.981562530940574,-1.,1.64665139190834));
#26895=CARTESIAN_POINT('Ctrl Pts',(0.981562530940574,1.,1.64665139190834));
#26896=CARTESIAN_POINT('Ctrl Pts',(0.985642622921626,-1.,1.6511001661277));
#26897=CARTESIAN_POINT('Ctrl Pts',(0.985642622921626,1.,1.6511001661277));
#26898=CARTESIAN_POINT('Ctrl Pts',(0.98985562785445,-1.,1.65559044289746));
#26899=CARTESIAN_POINT('Ctrl Pts',(0.98985562785445,1.,1.65559044289746));
#26900=CARTESIAN_POINT('Ctrl Pts',(0.994121836661115,-1.,1.66001553809916));
#26901=CARTESIAN_POINT('Ctrl Pts',(0.994121836661115,1.,1.66001553809916));
#26902=CARTESIAN_POINT('Ctrl Pts',(0.998389654952317,-1.,1.66430758030304));
#26903=CARTESIAN_POINT('Ctrl Pts',(0.998389654952317,1.,1.66430758030304));
#26904=CARTESIAN_POINT('Ctrl Pts',(1.00265091003682,-1.,1.66846059277231));
#26905=CARTESIAN_POINT('Ctrl Pts',(1.00265091003682,1.,1.66846059277231));
#26906=CARTESIAN_POINT('Ctrl Pts',(1.00692206696387,-1.,1.67250335383248));
#26907=CARTESIAN_POINT('Ctrl Pts',(1.00692206696387,1.,1.67250335383248));
#26908=CARTESIAN_POINT('Ctrl Pts',(1.01123236493507,-1.,1.67648246776457));
#26909=CARTESIAN_POINT('Ctrl Pts',(1.01123236493507,1.,1.67648246776457));
#26910=CARTESIAN_POINT('Ctrl Pts',(1.01561026162786,-1.,1.6804428989482));
#26911=CARTESIAN_POINT('Ctrl Pts',(1.01561026162786,1.,1.6804428989482));
#26912=CARTESIAN_POINT('Ctrl Pts',(1.02006795074222,-1.,1.68440578021739));
#26913=CARTESIAN_POINT('Ctrl Pts',(1.02006795074222,1.,1.68440578021739));
#26914=CARTESIAN_POINT('Ctrl Pts',(1.02460180535272,-1.,1.68836910178475));
#26915=CARTESIAN_POINT('Ctrl Pts',(1.02460180535272,1.,1.68836910178475));
#26916=CARTESIAN_POINT('Ctrl Pts',(1.02919977579155,-1.,1.69231840863471));
#26917=CARTESIAN_POINT('Ctrl Pts',(1.02919977579155,1.,1.69231840863471));
#26918=CARTESIAN_POINT('Ctrl Pts',(1.03384646003587,-1.,1.69623414782769));
#26919=CARTESIAN_POINT('Ctrl Pts',(1.03384646003587,1.,1.69623414782769));
#26920=CARTESIAN_POINT('Ctrl Pts',(1.03852922490782,-1.,1.70010052930951));
#26921=CARTESIAN_POINT('Ctrl Pts',(1.03852922490782,1.,1.70010052930951));
#26922=CARTESIAN_POINT('Ctrl Pts',(1.04324363334546,-1.,1.70391338707969));
#26923=CARTESIAN_POINT('Ctrl Pts',(1.04324363334546,1.,1.70391338707969));
#26924=CARTESIAN_POINT('Ctrl Pts',(1.0479908540499,-1.,1.70767646263641));
#26925=CARTESIAN_POINT('Ctrl Pts',(1.0479908540499,1.,1.70767646263641));
#26926=CARTESIAN_POINT('Ctrl Pts',(1.05277517202853,-1.,1.71139783543986));
#26927=CARTESIAN_POINT('Ctrl Pts',(1.05277517202853,1.,1.71139783543986));
#26928=CARTESIAN_POINT('Ctrl Pts',(1.05760163192481,-1.,1.71508654427022));
#26929=CARTESIAN_POINT('Ctrl Pts',(1.05760163192481,1.,1.71508654427022));
#26930=CARTESIAN_POINT('Ctrl Pts',(1.06247324680649,-1.,1.71874858456908));
#26931=CARTESIAN_POINT('Ctrl Pts',(1.06247324680649,1.,1.71874858456908));
#26932=CARTESIAN_POINT('Ctrl Pts',(1.06738966975463,-1.,1.72238500928456));
#26933=CARTESIAN_POINT('Ctrl Pts',(1.06738966975463,1.,1.72238500928456));
#26934=CARTESIAN_POINT('Ctrl Pts',(1.07234866990252,-1.,1.72599406198489));
#26935=CARTESIAN_POINT('Ctrl Pts',(1.07234866990252,1.,1.72599406198489));
#26936=CARTESIAN_POINT('Ctrl Pts',(1.0773470373727,-1.,1.72957248977424));
#26937=CARTESIAN_POINT('Ctrl Pts',(1.0773470373727,1.,1.72957248977424));
#26938=CARTESIAN_POINT('Ctrl Pts',(1.08238162784749,-1.,1.73311705663407));
#26939=CARTESIAN_POINT('Ctrl Pts',(1.08238162784749,1.,1.73311705663407));
#26940=CARTESIAN_POINT('Ctrl Pts',(1.08745056285429,-1.,1.73662628326093));
#26941=CARTESIAN_POINT('Ctrl Pts',(1.08745056285429,1.,1.73662628326093));
#26942=CARTESIAN_POINT('Ctrl Pts',(1.09255329056496,-1.,1.74010053962252));
#26943=CARTESIAN_POINT('Ctrl Pts',(1.09255329056496,1.,1.74010053962252));
#26944=CARTESIAN_POINT('Ctrl Pts',(1.09768999241229,-1.,1.74354119236212));
#26945=CARTESIAN_POINT('Ctrl Pts',(1.09768999241229,1.,1.74354119236212));
#26946=CARTESIAN_POINT('Ctrl Pts',(1.10286118991144,-1.,1.74695004214924));
#26947=CARTESIAN_POINT('Ctrl Pts',(1.10286118991144,1.,1.74695004214924));
#26948=CARTESIAN_POINT('Ctrl Pts',(1.10806728183003,-1.,1.75032866075914));
#26949=CARTESIAN_POINT('Ctrl Pts',(1.10806728183003,1.,1.75032866075914));
#26950=CARTESIAN_POINT('Ctrl Pts',(1.11330807582542,-1.,1.75367772094617));
#26951=CARTESIAN_POINT('Ctrl Pts',(1.11330807582542,1.,1.75367772094617));
#26952=CARTESIAN_POINT('Ctrl Pts',(1.11858293216752,-1.,1.75699720772089));
#26953=CARTESIAN_POINT('Ctrl Pts',(1.11858293216752,1.,1.75699720772089));
#26954=CARTESIAN_POINT('Ctrl Pts',(1.12389096855078,-1.,1.76028671825084));
#26955=CARTESIAN_POINT('Ctrl Pts',(1.12389096855078,1.,1.76028671825084));
#26956=CARTESIAN_POINT('Ctrl Pts',(1.12923123555076,-1.,1.76354571966171));
#26957=CARTESIAN_POINT('Ctrl Pts',(1.12923123555076,1.,1.76354571966171));
#26958=CARTESIAN_POINT('Ctrl Pts',(1.13460291804634,-1.,1.76677384551883));
#26959=CARTESIAN_POINT('Ctrl Pts',(1.13460291804634,1.,1.76677384551883));
#26960=CARTESIAN_POINT('Ctrl Pts',(1.14000548337,-1.,1.76997111386806));
#26961=CARTESIAN_POINT('Ctrl Pts',(1.14000548337,1.,1.76997111386806));
#26962=CARTESIAN_POINT('Ctrl Pts',(1.14543858226948,-1.,1.77313777896234));
#26963=CARTESIAN_POINT('Ctrl Pts',(1.14543858226948,1.,1.77313777896234));
#26964=CARTESIAN_POINT('Ctrl Pts',(1.15090197841531,-1.,1.77627422557034));
#26965=CARTESIAN_POINT('Ctrl Pts',(1.15090197841531,1.,1.77627422557034));
#26966=CARTESIAN_POINT('Ctrl Pts',(1.15639547194689,-1.,1.77938085564261));
#26967=CARTESIAN_POINT('Ctrl Pts',(1.15639547194689,1.,1.77938085564261));
#26968=CARTESIAN_POINT('Ctrl Pts',(1.16191881298458,-1.,1.78245795880949));
#26969=CARTESIAN_POINT('Ctrl Pts',(1.16191881298458,1.,1.78245795880949));
#26970=CARTESIAN_POINT('Ctrl Pts',(1.16747166312239,-1.,1.78550566040349));
#26971=CARTESIAN_POINT('Ctrl Pts',(1.16747166312239,1.,1.78550566040349));
#26972=CARTESIAN_POINT('Ctrl Pts',(1.17305363177265,-1.,1.78852398877523));
#26973=CARTESIAN_POINT('Ctrl Pts',(1.17305363177265,1.,1.78852398877523));
#26974=CARTESIAN_POINT('Ctrl Pts',(1.17866429440781,-1.,1.79151291552646));
#26975=CARTESIAN_POINT('Ctrl Pts',(1.17866429440781,1.,1.79151291552646));
#26976=CARTESIAN_POINT('Ctrl Pts',(1.18430321697471,-1.,1.79447240321572));
#26977=CARTESIAN_POINT('Ctrl Pts',(1.18430321697471,1.,1.79447240321572));
#26978=CARTESIAN_POINT('Ctrl Pts',(1.1899699793456,-1.,1.79740245923649));
#26979=CARTESIAN_POINT('Ctrl Pts',(1.1899699793456,1.,1.79740245923649));
#26980=CARTESIAN_POINT('Ctrl Pts',(1.19566418930405,-1.,1.80030314370121));
#26981=CARTESIAN_POINT('Ctrl Pts',(1.19566418930405,1.,1.80030314370121));
#26982=CARTESIAN_POINT('Ctrl Pts',(1.2013854893912,-1.,1.8031745483882));
#26983=CARTESIAN_POINT('Ctrl Pts',(1.2013854893912,1.,1.8031745483882));
#26984=CARTESIAN_POINT('Ctrl Pts',(1.20713356605519,-1.,1.80601678480772));
#26985=CARTESIAN_POINT('Ctrl Pts',(1.20713356605519,1.,1.80601678480772));
#26986=CARTESIAN_POINT('Ctrl Pts',(1.2129081570818,-1.,1.80882996916931));
#26987=CARTESIAN_POINT('Ctrl Pts',(1.2129081570818,1.,1.80882996916931));
#26988=CARTESIAN_POINT('Ctrl Pts',(1.2187090610323,-1.,1.81161420806172));
#26989=CARTESIAN_POINT('Ctrl Pts',(1.2187090610323,1.,1.81161420806172));
#26990=CARTESIAN_POINT('Ctrl Pts',(1.22453613304507,-1.,1.81436959209778));
#26991=CARTESIAN_POINT('Ctrl Pts',(1.22453613304507,1.,1.81436959209778));
#26992=CARTESIAN_POINT('Ctrl Pts',(1.22921864890975,-1.,1.81655087183054));
#26993=CARTESIAN_POINT('Ctrl Pts',(1.22921864890975,1.,1.81655087183054));
#26994=CARTESIAN_POINT('Ctrl Pts',(1.23274224526804,-1.,1.81817389920914));
#26995=CARTESIAN_POINT('Ctrl Pts',(1.23274224526804,1.,1.81817389920914));
#26996=CARTESIAN_POINT('Ctrl Pts',(1.23509651170384,-1.,1.81925017193531));
#26997=CARTESIAN_POINT('Ctrl Pts',(1.23509651170384,1.,1.81925017193531));
#26998=CARTESIAN_POINT('Ctrl Pts',(1.23627494547115,-1.,1.81978687191668));
#26999=CARTESIAN_POINT('Ctrl Pts',(1.23627494547115,1.,1.81978687191668));
#27000=CARTESIAN_POINT('',(0.892032620296855,1.,1.5055822144029));
#27001=CARTESIAN_POINT('Ctrl Pts',(0.892032620296855,1.,1.5055822144029));
#27002=CARTESIAN_POINT('Ctrl Pts',(0.894452006967538,1.,1.50980486807181));
#27003=CARTESIAN_POINT('Ctrl Pts',(0.89918504749193,1.,1.51805569591479));
#27004=CARTESIAN_POINT('Ctrl Pts',(0.905967409640498,1.,1.52984849890434));
#27005=CARTESIAN_POINT('Ctrl Pts',(0.914375919046579,1.,1.54440491152808));
#27006=CARTESIAN_POINT('Ctrl Pts',(0.923832188966322,1.,1.56065988582509));
#27007=CARTESIAN_POINT('Ctrl Pts',(0.932246680128848,1.,1.57499388385561));
#27008=CARTESIAN_POINT('Ctrl Pts',(0.939646377909319,1.,1.58744937489796));
#27009=CARTESIAN_POINT('Ctrl Pts',(0.946078063325795,1.,1.59810042045408));
#27010=CARTESIAN_POINT('Ctrl Pts',(0.951613284361247,1.,1.60706069897794));
#27011=CARTESIAN_POINT('Ctrl Pts',(0.956354422921572,1.,1.61449324337233));
#27012=CARTESIAN_POINT('Ctrl Pts',(0.960438326099958,1.,1.62061638139929));
#27013=CARTESIAN_POINT('Ctrl Pts',(0.964046107037821,1.,1.6257193066974));
#27014=CARTESIAN_POINT('Ctrl Pts',(0.967387853228041,1.,1.63013849959083));
#27015=CARTESIAN_POINT('Ctrl Pts',(0.970669715996356,1.,1.63420665729609));
#27016=CARTESIAN_POINT('Ctrl Pts',(0.974066058287501,1.,1.63820952658157));
#27017=CARTESIAN_POINT('Ctrl Pts',(0.977689794120296,1.,1.64233990826831));
#27018=CARTESIAN_POINT('Ctrl Pts',(0.981562530940574,1.,1.64665139190834));
#27019=CARTESIAN_POINT('Ctrl Pts',(0.985642622921626,1.,1.6511001661277));
#27020=CARTESIAN_POINT('Ctrl Pts',(0.98985562785445,1.,1.65559044289746));
#27021=CARTESIAN_POINT('Ctrl Pts',(0.994121836661115,1.,1.66001553809916));
#27022=CARTESIAN_POINT('Ctrl Pts',(0.998389654952317,1.,1.66430758030304));
#27023=CARTESIAN_POINT('Ctrl Pts',(1.00265091003682,1.,1.66846059277231));
#27024=CARTESIAN_POINT('Ctrl Pts',(1.00692206696387,1.,1.67250335383248));
#27025=CARTESIAN_POINT('Ctrl Pts',(1.01123236493507,1.,1.67648246776457));
#27026=CARTESIAN_POINT('Ctrl Pts',(1.01561026162786,1.,1.6804428989482));
#27027=CARTESIAN_POINT('Ctrl Pts',(1.02006795074222,1.,1.68440578021739));
#27028=CARTESIAN_POINT('Ctrl Pts',(1.02460180535272,1.,1.68836910178475));
#27029=CARTESIAN_POINT('Ctrl Pts',(1.02919977579155,1.,1.69231840863471));
#27030=CARTESIAN_POINT('Ctrl Pts',(1.03384646003587,1.,1.69623414782769));
#27031=CARTESIAN_POINT('Ctrl Pts',(1.03852922490782,1.,1.70010052930951));
#27032=CARTESIAN_POINT('Ctrl Pts',(1.04324363334546,1.,1.70391338707969));
#27033=CARTESIAN_POINT('Ctrl Pts',(1.0479908540499,1.,1.70767646263641));
#27034=CARTESIAN_POINT('Ctrl Pts',(1.05277517202853,1.,1.71139783543986));
#27035=CARTESIAN_POINT('Ctrl Pts',(1.05760163192481,1.,1.71508654427022));
#27036=CARTESIAN_POINT('Ctrl Pts',(1.06247324680649,1.,1.71874858456908));
#27037=CARTESIAN_POINT('Ctrl Pts',(1.06738966975463,1.,1.72238500928456));
#27038=CARTESIAN_POINT('Ctrl Pts',(1.07234866990252,1.,1.72599406198489));
#27039=CARTESIAN_POINT('Ctrl Pts',(1.0773470373727,1.,1.72957248977424));
#27040=CARTESIAN_POINT('Ctrl Pts',(1.08238162784749,1.,1.73311705663407));
#27041=CARTESIAN_POINT('Ctrl Pts',(1.08745056285429,1.,1.73662628326093));
#27042=CARTESIAN_POINT('Ctrl Pts',(1.09255329056496,1.,1.74010053962252));
#27043=CARTESIAN_POINT('Ctrl Pts',(1.09768999241229,1.,1.74354119236212));
#27044=CARTESIAN_POINT('Ctrl Pts',(1.10286118991144,1.,1.74695004214924));
#27045=CARTESIAN_POINT('Ctrl Pts',(1.10806728183003,1.,1.75032866075914));
#27046=CARTESIAN_POINT('Ctrl Pts',(1.11330807582542,1.,1.75367772094617));
#27047=CARTESIAN_POINT('Ctrl Pts',(1.11858293216752,1.,1.75699720772089));
#27048=CARTESIAN_POINT('Ctrl Pts',(1.12389096855078,1.,1.76028671825084));
#27049=CARTESIAN_POINT('Ctrl Pts',(1.12923123555076,1.,1.76354571966171));
#27050=CARTESIAN_POINT('Ctrl Pts',(1.13460291804634,1.,1.76677384551883));
#27051=CARTESIAN_POINT('Ctrl Pts',(1.14000548337,1.,1.76997111386806));
#27052=CARTESIAN_POINT('Ctrl Pts',(1.14543858226948,1.,1.77313777896234));
#27053=CARTESIAN_POINT('Ctrl Pts',(1.15090197841531,1.,1.77627422557034));
#27054=CARTESIAN_POINT('Ctrl Pts',(1.15639547194689,1.,1.77938085564261));
#27055=CARTESIAN_POINT('Ctrl Pts',(1.16191881298458,1.,1.78245795880949));
#27056=CARTESIAN_POINT('Ctrl Pts',(1.16747166312239,1.,1.78550566040349));
#27057=CARTESIAN_POINT('Ctrl Pts',(1.17305363177265,1.,1.78852398877523));
#27058=CARTESIAN_POINT('Ctrl Pts',(1.17866429440781,1.,1.79151291552646));
#27059=CARTESIAN_POINT('Ctrl Pts',(1.18430321697471,1.,1.79447240321572));
#27060=CARTESIAN_POINT('Ctrl Pts',(1.1899699793456,1.,1.79740245923649));
#27061=CARTESIAN_POINT('Ctrl Pts',(1.19566418930405,1.,1.80030314370121));
#27062=CARTESIAN_POINT('Ctrl Pts',(1.2013854893912,1.,1.8031745483882));
#27063=CARTESIAN_POINT('Ctrl Pts',(1.20713356605519,1.,1.80601678480772));
#27064=CARTESIAN_POINT('Ctrl Pts',(1.2129081570818,1.,1.80882996916931));
#27065=CARTESIAN_POINT('Ctrl Pts',(1.2187090610323,1.,1.81161420806172));
#27066=CARTESIAN_POINT('Ctrl Pts',(1.22453613304507,1.,1.81436959209778));
#27067=CARTESIAN_POINT('Ctrl Pts',(1.22921864890975,1.,1.81655087183054));
#27068=CARTESIAN_POINT('Ctrl Pts',(1.23274224526804,1.,1.81817389920914));
#27069=CARTESIAN_POINT('Ctrl Pts',(1.23509651170384,1.,1.81925017193531));
#27070=CARTESIAN_POINT('Ctrl Pts',(1.23627494547115,1.,1.81978687191668));
#27071=CARTESIAN_POINT('',(0.892032620296854,0.,1.5055822144029));
#27072=CARTESIAN_POINT('Origin',(0.,0.,0.));
#27073=CARTESIAN_POINT('',(0.693717979106305,1.,1.60662857109684));
#27074=CARTESIAN_POINT('Origin',(0.,1.,0.));
#27075=CARTESIAN_POINT('',(0.693717979106305,0.,1.60662857109684));
#27076=CARTESIAN_POINT('Ctrl Pts',(0.7455743247944,-1.,2.0698113262342));
#27077=CARTESIAN_POINT('Ctrl Pts',(0.7455743247944,1.,2.0698113262342));
#27078=CARTESIAN_POINT('Ctrl Pts',(0.745832791378367,-1.,2.06854248895728));
#27079=CARTESIAN_POINT('Ctrl Pts',(0.745832791378367,1.,2.06854248895728));
#27080=CARTESIAN_POINT('Ctrl Pts',(0.7463458715442,-1.,2.06600523016815));
#27081=CARTESIAN_POINT('Ctrl Pts',(0.7463458715442,1.,2.06600523016815));
#27082=CARTESIAN_POINT('Ctrl Pts',(0.747103932787919,-1.,2.06220058927826));
#27083=CARTESIAN_POINT('Ctrl Pts',(0.747103932787919,1.,2.06220058927826));
#27084=CARTESIAN_POINT('Ctrl Pts',(0.748091554183802,-1.,2.05713023031007));
#27085=CARTESIAN_POINT('Ctrl Pts',(0.748091554183802,1.,2.05713023031007));
#27086=CARTESIAN_POINT('Ctrl Pts',(0.749287468665046,-1.,2.05079645592154));
#27087=CARTESIAN_POINT('Ctrl Pts',(0.749287468665046,1.,2.05079645592154));
#27088=CARTESIAN_POINT('Ctrl Pts',(0.750444657875575,-1.,2.04446689147979));
#27089=CARTESIAN_POINT('Ctrl Pts',(0.750444657875575,1.,2.04446689147979));
#27090=CARTESIAN_POINT('Ctrl Pts',(0.751562963361115,-1.,2.03814160092099));
#27091=CARTESIAN_POINT('Ctrl Pts',(0.751562963361115,1.,2.03814160092099));
#27092=CARTESIAN_POINT('Ctrl Pts',(0.75264218048721,-1.,2.03182068456221));
#27093=CARTESIAN_POINT('Ctrl Pts',(0.75264218048721,1.,2.03182068456221));
#27094=CARTESIAN_POINT('Ctrl Pts',(0.753682061112768,-1.,2.02550428623313));
#27095=CARTESIAN_POINT('Ctrl Pts',(0.753682061112768,1.,2.02550428623313));
#27096=CARTESIAN_POINT('Ctrl Pts',(0.754682330722816,-1.,2.01919259405809));
#27097=CARTESIAN_POINT('Ctrl Pts',(0.754682330722816,1.,2.01919259405809));
#27098=CARTESIAN_POINT('Ctrl Pts',(0.755642704957865,-1.,2.01288584328084));
#27099=CARTESIAN_POINT('Ctrl Pts',(0.755642704957865,1.,2.01288584328084));
#27100=CARTESIAN_POINT('Ctrl Pts',(0.75656290464667,-1.,2.0065843158773));
#27101=CARTESIAN_POINT('Ctrl Pts',(0.75656290464667,1.,2.0065843158773));
#27102=CARTESIAN_POINT('Ctrl Pts',(0.757442676862724,-1.,2.00028834739178));
#27103=CARTESIAN_POINT('Ctrl Pts',(0.757442676862724,1.,2.00028834739178));
#27104=CARTESIAN_POINT('Ctrl Pts',(0.758281796766761,-1.,1.99399831098817));
#27105=CARTESIAN_POINT('Ctrl Pts',(0.758281796766761,1.,1.99399831098817));
#27106=CARTESIAN_POINT('Ctrl Pts',(0.759080037802488,-1.,1.98771456680874));
#27107=CARTESIAN_POINT('Ctrl Pts',(0.759080037802488,1.,1.98771456680874));
#27108=CARTESIAN_POINT('Ctrl Pts',(0.75983714745219,-1.,1.98143741418172));
#27109=CARTESIAN_POINT('Ctrl Pts',(0.75983714745219,1.,1.98143741418172));
#27110=CARTESIAN_POINT('Ctrl Pts',(0.760552825409757,-1.,1.97516705321494));
#27111=CARTESIAN_POINT('Ctrl Pts',(0.760552825409757,1.,1.97516705321494));
#27112=CARTESIAN_POINT('Ctrl Pts',(0.76122669048382,-1.,1.96890351582499));
#27113=CARTESIAN_POINT('Ctrl Pts',(0.76122669048382,1.,1.96890351582499));
#27114=CARTESIAN_POINT('Ctrl Pts',(0.761858300014423,-1.,1.96264672744186));
#27115=CARTESIAN_POINT('Ctrl Pts',(0.761858300014423,1.,1.96264672744186));
#27116=CARTESIAN_POINT('Ctrl Pts',(0.762447203806178,-1.,1.95639665309869));
#27117=CARTESIAN_POINT('Ctrl Pts',(0.762447203806178,1.,1.95639665309869));
#27118=CARTESIAN_POINT('Ctrl Pts',(0.762992990878769,-1.,1.95015342590024));
#27119=CARTESIAN_POINT('Ctrl Pts',(0.762992990878769,1.,1.95015342590024));
#27120=CARTESIAN_POINT('Ctrl Pts',(0.763495333538629,-1.,1.9439174661764));
#27121=CARTESIAN_POINT('Ctrl Pts',(0.763495333538629,1.,1.9439174661764));
#27122=CARTESIAN_POINT('Ctrl Pts',(0.763954049121458,-1.,1.93768964875886));
#27123=CARTESIAN_POINT('Ctrl Pts',(0.763954049121458,1.,1.93768964875886));
#27124=CARTESIAN_POINT('Ctrl Pts',(0.76436901067394,-1.,1.93147105496382));
#27125=CARTESIAN_POINT('Ctrl Pts',(0.76436901067394,1.,1.93147105496382));
#27126=CARTESIAN_POINT('Ctrl Pts',(0.764740025488211,-1.,1.92526263537048));
#27127=CARTESIAN_POINT('Ctrl Pts',(0.764740025488211,1.,1.92526263537048));
#27128=CARTESIAN_POINT('Ctrl Pts',(0.765066729667088,-1.,1.91906491634196));
#27129=CARTESIAN_POINT('Ctrl Pts',(0.765066729667088,1.,1.91906491634196));
#27130=CARTESIAN_POINT('Ctrl Pts',(0.765348465884722,-1.,1.91287765805169));
#27131=CARTESIAN_POINT('Ctrl Pts',(0.765348465884722,1.,1.91287765805169));
#27132=CARTESIAN_POINT('Ctrl Pts',(0.765584196937919,-1.,1.90669961402356));
#27133=CARTESIAN_POINT('Ctrl Pts',(0.765584196937919,1.,1.90669961402356));
#27134=CARTESIAN_POINT('Ctrl Pts',(0.765772772593386,-1.,1.90052930393596));
#27135=CARTESIAN_POINT('Ctrl Pts',(0.765772772593386,1.,1.90052930393596));
#27136=CARTESIAN_POINT('Ctrl Pts',(0.765913193856978,-1.,1.89436577771388));
#27137=CARTESIAN_POINT('Ctrl Pts',(0.765913193856978,1.,1.89436577771388));
#27138=CARTESIAN_POINT('Ctrl Pts',(0.766004837062091,-1.,1.88820926433409));
#27139=CARTESIAN_POINT('Ctrl Pts',(0.766004837062091,1.,1.88820926433409));
#27140=CARTESIAN_POINT('Ctrl Pts',(0.766047794851864,-1.,1.88206215302561));
#27141=CARTESIAN_POINT('Ctrl Pts',(0.766047794851864,1.,1.88206215302561));
#27142=CARTESIAN_POINT('Ctrl Pts',(0.766042837036744,-1.,1.87592888967883));
#27143=CARTESIAN_POINT('Ctrl Pts',(0.766042837036744,1.,1.87592888967883));
#27144=CARTESIAN_POINT('Ctrl Pts',(0.765990708546091,-1.,1.86981398314341));
#27145=CARTESIAN_POINT('Ctrl Pts',(0.765990708546091,1.,1.86981398314341));
#27146=CARTESIAN_POINT('Ctrl Pts',(0.765891519092547,-1.,1.86372027063312));
#27147=CARTESIAN_POINT('Ctrl Pts',(0.765891519092547,1.,1.86372027063312));
#27148=CARTESIAN_POINT('Ctrl Pts',(0.765744212909318,-1.,1.85764741390394));
#27149=CARTESIAN_POINT('Ctrl Pts',(0.765744212909318,1.,1.85764741390394));
#27150=CARTESIAN_POINT('Ctrl Pts',(0.765545710619062,-1.,1.85158945130063));
#27151=CARTESIAN_POINT('Ctrl Pts',(0.765545710619062,1.,1.85158945130063));
#27152=CARTESIAN_POINT('Ctrl Pts',(0.765291664862029,-1.,1.84553698875924));
#27153=CARTESIAN_POINT('Ctrl Pts',(0.765291664862029,1.,1.84553698875924));
#27154=CARTESIAN_POINT('Ctrl Pts',(0.764978057881737,-1.,1.83948181064835));
#27155=CARTESIAN_POINT('Ctrl Pts',(0.764978057881737,1.,1.83948181064835));
#27156=CARTESIAN_POINT('Ctrl Pts',(0.764602549687853,-1.,1.83342077227142));
#27157=CARTESIAN_POINT('Ctrl Pts',(0.764602549687853,1.,1.83342077227142));
#27158=CARTESIAN_POINT('Ctrl Pts',(0.764165902605995,-1.,1.82735991200065));
#27159=CARTESIAN_POINT('Ctrl Pts',(0.764165902605995,1.,1.82735991200065));
#27160=CARTESIAN_POINT('Ctrl Pts',(0.763673465462726,-1.,1.82131873145266));
#27161=CARTESIAN_POINT('Ctrl Pts',(0.763673465462726,1.,1.82131873145266));
#27162=CARTESIAN_POINT('Ctrl Pts',(0.763132003836634,-1.,1.8153211840553));
#27163=CARTESIAN_POINT('Ctrl Pts',(0.763132003836634,1.,1.8153211840553));
#27164=CARTESIAN_POINT('Ctrl Pts',(0.762546129463938,-1.,1.80938551463965));
#27165=CARTESIAN_POINT('Ctrl Pts',(0.762546129463938,1.,1.80938551463965));
#27166=CARTESIAN_POINT('Ctrl Pts',(0.761915336443547,-1.,1.80351583877342));
#27167=CARTESIAN_POINT('Ctrl Pts',(0.761915336443547,1.,1.80351583877342));
#27168=CARTESIAN_POINT('Ctrl Pts',(0.761229695230558,-1.,1.79768986997783));
#27169=CARTESIAN_POINT('Ctrl Pts',(0.761229695230558,1.,1.79768986997783));
#27170=CARTESIAN_POINT('Ctrl Pts',(0.760469555880749,-1.,1.7918581561088));
#27171=CARTESIAN_POINT('Ctrl Pts',(0.760469555880749,1.,1.7918581561088));
#27172=CARTESIAN_POINT('Ctrl Pts',(0.759614401110189,-1.,1.78596964884604));
#27173=CARTESIAN_POINT('Ctrl Pts',(0.759614401110189,1.,1.78596964884604));
#27174=CARTESIAN_POINT('Ctrl Pts',(0.758650626677518,-1.,1.77999411220945));
#27175=CARTESIAN_POINT('Ctrl Pts',(0.758650626677518,1.,1.77999411220945));
#27176=CARTESIAN_POINT('Ctrl Pts',(0.757578264077028,-1.,1.77394167108292));
#27177=CARTESIAN_POINT('Ctrl Pts',(0.757578264077028,1.,1.77394167108292));
#27178=CARTESIAN_POINT('Ctrl Pts',(0.75642189602781,-1.,1.76789396002998));
#27179=CARTESIAN_POINT('Ctrl Pts',(0.75642189602781,1.,1.76789396002998));
#27180=CARTESIAN_POINT('Ctrl Pts',(0.755220979974461,-1.,1.76197817240128));
#27181=CARTESIAN_POINT('Ctrl Pts',(0.755220979974461,1.,1.76197817240128));
#27182=CARTESIAN_POINT('Ctrl Pts',(0.754009254027828,-1.,1.75631083600019));
#27183=CARTESIAN_POINT('Ctrl Pts',(0.754009254027828,1.,1.75631083600019));
#27184=CARTESIAN_POINT('Ctrl Pts',(0.752797683531314,-1.,1.75095139468794));
#27185=CARTESIAN_POINT('Ctrl Pts',(0.752797683531314,1.,1.75095139468794));
#27186=CARTESIAN_POINT('Ctrl Pts',(0.751555614164482,-1.,1.74585086852502));
#27187=CARTESIAN_POINT('Ctrl Pts',(0.751555614164482,1.,1.74585086852502));
#27188=CARTESIAN_POINT('Ctrl Pts',(0.750193435981249,-1.,1.74080458267114));
#27189=CARTESIAN_POINT('Ctrl Pts',(0.750193435981249,1.,1.74080458267114));
#27190=CARTESIAN_POINT('Ctrl Pts',(0.74858246295687,-1.,1.7355035168033));
#27191=CARTESIAN_POINT('Ctrl Pts',(0.74858246295687,1.,1.7355035168033));
#27192=CARTESIAN_POINT('Ctrl Pts',(0.746574710097752,-1.,1.72958533647714));
#27193=CARTESIAN_POINT('Ctrl Pts',(0.746574710097752,1.,1.72958533647714));
#27194=CARTESIAN_POINT('Ctrl Pts',(0.744021445433093,-1.,1.72268229916769));
#27195=CARTESIAN_POINT('Ctrl Pts',(0.744021445433093,1.,1.72268229916769));
#27196=CARTESIAN_POINT('Ctrl Pts',(0.74079516202821,-1.,1.71447789751001));
#27197=CARTESIAN_POINT('Ctrl Pts',(0.74079516202821,1.,1.71447789751001));
#27198=CARTESIAN_POINT('Ctrl Pts',(0.736799665716932,-1.,1.70473309004249));
#27199=CARTESIAN_POINT('Ctrl Pts',(0.736799665716932,1.,1.70473309004249));
#27200=CARTESIAN_POINT('Ctrl Pts',(0.731963238685357,-1.,1.69326921972915));
#27201=CARTESIAN_POINT('Ctrl Pts',(0.731963238685357,1.,1.69326921972915));
#27202=CARTESIAN_POINT('Ctrl Pts',(0.726235967982445,-1.,1.67996158451922));
#27203=CARTESIAN_POINT('Ctrl Pts',(0.726235967982445,1.,1.67996158451922));
#27204=CARTESIAN_POINT('Ctrl Pts',(0.719585433787949,-1.,1.66472880551777));
#27205=CARTESIAN_POINT('Ctrl Pts',(0.719585433787949,1.,1.66472880551777));
#27206=CARTESIAN_POINT('Ctrl Pts',(0.711993139340447,-1.,1.64752408828442));
#27207=CARTESIAN_POINT('Ctrl Pts',(0.711993139340447,1.,1.64752408828442));
#27208=CARTESIAN_POINT('Ctrl Pts',(0.705159151977294,-1.,1.6321654166204));
#27209=CARTESIAN_POINT('Ctrl Pts',(0.705159151977294,1.,1.6321654166204));
#27210=CARTESIAN_POINT('Ctrl Pts',(0.699605146398836,-1.,1.61974673471117));
#27211=CARTESIAN_POINT('Ctrl Pts',(0.699605146398836,1.,1.61974673471117));
#27212=CARTESIAN_POINT('Ctrl Pts',(0.69571209787897,-1.,1.61106790957619));
#27213=CARTESIAN_POINT('Ctrl Pts',(0.69571209787897,1.,1.61106790957619));
#27214=CARTESIAN_POINT('Ctrl Pts',(0.693717979106305,-1.,1.60662857109684));
#27215=CARTESIAN_POINT('Ctrl Pts',(0.693717979106305,1.,1.60662857109684));
#27216=CARTESIAN_POINT('',(0.7455743247944,1.,2.0698113262342));
#27217=CARTESIAN_POINT('Ctrl Pts',(0.7455743247944,1.,2.0698113262342));
#27218=CARTESIAN_POINT('Ctrl Pts',(0.745832791378367,1.,2.06854248895728));
#27219=CARTESIAN_POINT('Ctrl Pts',(0.7463458715442,1.,2.06600523016815));
#27220=CARTESIAN_POINT('Ctrl Pts',(0.747103932787919,1.,2.06220058927826));
#27221=CARTESIAN_POINT('Ctrl Pts',(0.748091554183802,1.,2.05713023031007));
#27222=CARTESIAN_POINT('Ctrl Pts',(0.749287468665046,1.,2.05079645592154));
#27223=CARTESIAN_POINT('Ctrl Pts',(0.750444657875575,1.,2.04446689147979));
#27224=CARTESIAN_POINT('Ctrl Pts',(0.751562963361115,1.,2.03814160092099));
#27225=CARTESIAN_POINT('Ctrl Pts',(0.75264218048721,1.,2.03182068456221));
#27226=CARTESIAN_POINT('Ctrl Pts',(0.753682061112768,1.,2.02550428623313));
#27227=CARTESIAN_POINT('Ctrl Pts',(0.754682330722816,1.,2.01919259405809));
#27228=CARTESIAN_POINT('Ctrl Pts',(0.755642704957865,1.,2.01288584328084));
#27229=CARTESIAN_POINT('Ctrl Pts',(0.75656290464667,1.,2.0065843158773));
#27230=CARTESIAN_POINT('Ctrl Pts',(0.757442676862724,1.,2.00028834739178));
#27231=CARTESIAN_POINT('Ctrl Pts',(0.758281796766761,1.,1.99399831098817));
#27232=CARTESIAN_POINT('Ctrl Pts',(0.759080037802488,1.,1.98771456680874));
#27233=CARTESIAN_POINT('Ctrl Pts',(0.75983714745219,1.,1.98143741418172));
#27234=CARTESIAN_POINT('Ctrl Pts',(0.760552825409757,1.,1.97516705321494));
#27235=CARTESIAN_POINT('Ctrl Pts',(0.76122669048382,1.,1.96890351582499));
#27236=CARTESIAN_POINT('Ctrl Pts',(0.761858300014423,1.,1.96264672744186));
#27237=CARTESIAN_POINT('Ctrl Pts',(0.762447203806178,1.,1.95639665309869));
#27238=CARTESIAN_POINT('Ctrl Pts',(0.762992990878769,1.,1.95015342590024));
#27239=CARTESIAN_POINT('Ctrl Pts',(0.763495333538629,1.,1.9439174661764));
#27240=CARTESIAN_POINT('Ctrl Pts',(0.763954049121458,1.,1.93768964875886));
#27241=CARTESIAN_POINT('Ctrl Pts',(0.76436901067394,1.,1.93147105496382));
#27242=CARTESIAN_POINT('Ctrl Pts',(0.764740025488211,1.,1.92526263537048));
#27243=CARTESIAN_POINT('Ctrl Pts',(0.765066729667088,1.,1.91906491634196));
#27244=CARTESIAN_POINT('Ctrl Pts',(0.765348465884722,1.,1.91287765805169));
#27245=CARTESIAN_POINT('Ctrl Pts',(0.765584196937919,1.,1.90669961402356));
#27246=CARTESIAN_POINT('Ctrl Pts',(0.765772772593386,1.,1.90052930393596));
#27247=CARTESIAN_POINT('Ctrl Pts',(0.765913193856978,1.,1.89436577771388));
#27248=CARTESIAN_POINT('Ctrl Pts',(0.766004837062091,1.,1.88820926433409));
#27249=CARTESIAN_POINT('Ctrl Pts',(0.766047794851864,1.,1.88206215302561));
#27250=CARTESIAN_POINT('Ctrl Pts',(0.766042837036744,1.,1.87592888967883));
#27251=CARTESIAN_POINT('Ctrl Pts',(0.765990708546091,1.,1.86981398314341));
#27252=CARTESIAN_POINT('Ctrl Pts',(0.765891519092547,1.,1.86372027063312));
#27253=CARTESIAN_POINT('Ctrl Pts',(0.765744212909318,1.,1.85764741390394));
#27254=CARTESIAN_POINT('Ctrl Pts',(0.765545710619062,1.,1.85158945130063));
#27255=CARTESIAN_POINT('Ctrl Pts',(0.765291664862029,1.,1.84553698875924));
#27256=CARTESIAN_POINT('Ctrl Pts',(0.764978057881737,1.,1.83948181064835));
#27257=CARTESIAN_POINT('Ctrl Pts',(0.764602549687853,1.,1.83342077227142));
#27258=CARTESIAN_POINT('Ctrl Pts',(0.764165902605995,1.,1.82735991200065));
#27259=CARTESIAN_POINT('Ctrl Pts',(0.763673465462726,1.,1.82131873145266));
#27260=CARTESIAN_POINT('Ctrl Pts',(0.763132003836634,1.,1.8153211840553));
#27261=CARTESIAN_POINT('Ctrl Pts',(0.762546129463938,1.,1.80938551463965));
#27262=CARTESIAN_POINT('Ctrl Pts',(0.761915336443547,1.,1.80351583877342));
#27263=CARTESIAN_POINT('Ctrl Pts',(0.761229695230558,1.,1.79768986997783));
#27264=CARTESIAN_POINT('Ctrl Pts',(0.760469555880749,1.,1.7918581561088));
#27265=CARTESIAN_POINT('Ctrl Pts',(0.759614401110189,1.,1.78596964884604));
#27266=CARTESIAN_POINT('Ctrl Pts',(0.758650626677518,1.,1.77999411220945));
#27267=CARTESIAN_POINT('Ctrl Pts',(0.757578264077028,1.,1.77394167108292));
#27268=CARTESIAN_POINT('Ctrl Pts',(0.75642189602781,1.,1.76789396002998));
#27269=CARTESIAN_POINT('Ctrl Pts',(0.755220979974461,1.,1.76197817240128));
#27270=CARTESIAN_POINT('Ctrl Pts',(0.754009254027828,1.,1.75631083600019));
#27271=CARTESIAN_POINT('Ctrl Pts',(0.752797683531314,1.,1.75095139468794));
#27272=CARTESIAN_POINT('Ctrl Pts',(0.751555614164482,1.,1.74585086852502));
#27273=CARTESIAN_POINT('Ctrl Pts',(0.750193435981249,1.,1.74080458267114));
#27274=CARTESIAN_POINT('Ctrl Pts',(0.74858246295687,1.,1.7355035168033));
#27275=CARTESIAN_POINT('Ctrl Pts',(0.746574710097752,1.,1.72958533647714));
#27276=CARTESIAN_POINT('Ctrl Pts',(0.744021445433093,1.,1.72268229916769));
#27277=CARTESIAN_POINT('Ctrl Pts',(0.74079516202821,1.,1.71447789751001));
#27278=CARTESIAN_POINT('Ctrl Pts',(0.736799665716932,1.,1.70473309004249));
#27279=CARTESIAN_POINT('Ctrl Pts',(0.731963238685357,1.,1.69326921972915));
#27280=CARTESIAN_POINT('Ctrl Pts',(0.726235967982445,1.,1.67996158451922));
#27281=CARTESIAN_POINT('Ctrl Pts',(0.719585433787949,1.,1.66472880551777));
#27282=CARTESIAN_POINT('Ctrl Pts',(0.711993139340447,1.,1.64752408828442));
#27283=CARTESIAN_POINT('Ctrl Pts',(0.705159151977294,1.,1.6321654166204));
#27284=CARTESIAN_POINT('Ctrl Pts',(0.699605146398836,1.,1.61974673471117));
#27285=CARTESIAN_POINT('Ctrl Pts',(0.69571209787897,1.,1.61106790957619));
#27286=CARTESIAN_POINT('Ctrl Pts',(0.693717979106305,1.,1.60662857109684));
#27287=CARTESIAN_POINT('',(0.7455743247944,0.,2.0698113262342));
#27288=CARTESIAN_POINT('Origin',(0.61342227326009,0.,2.11275013067528));
#27289=CARTESIAN_POINT('',(0.61342227326009,1.,2.11275013067528));
#27290=CARTESIAN_POINT('',(0.7455743247944,1.,2.0698113262342));
#27291=CARTESIAN_POINT('',(0.61342227326009,0.,2.11275013067528));
#27292=CARTESIAN_POINT('Ctrl Pts',(0.383122945602004,-1.,1.7075470150345));
#27293=CARTESIAN_POINT('Ctrl Pts',(0.383122945602004,1.,1.7075470150345));
#27294=CARTESIAN_POINT('Ctrl Pts',(0.384119047315541,-1.,1.71231062891958));
#27295=CARTESIAN_POINT('Ctrl Pts',(0.384119047315541,1.,1.71231062891958));
#27296=CARTESIAN_POINT('Ctrl Pts',(0.38607079032701,-1.,1.72162022246158));
#27297=CARTESIAN_POINT('Ctrl Pts',(0.38607079032701,1.,1.72162022246158));
#27298=CARTESIAN_POINT('Ctrl Pts',(0.388877023509191,-1.,1.7349317097561));
#27299=CARTESIAN_POINT('Ctrl Pts',(0.388877023509191,1.,1.7349317097561));
#27300=CARTESIAN_POINT('Ctrl Pts',(0.392375812294307,-1.,1.75137405313962));
#27301=CARTESIAN_POINT('Ctrl Pts',(0.392375812294307,1.,1.75137405313962));
#27302=CARTESIAN_POINT('Ctrl Pts',(0.39634619612042,-1.,1.7697556004756));
#27303=CARTESIAN_POINT('Ctrl Pts',(0.39634619612042,1.,1.7697556004756));
#27304=CARTESIAN_POINT('Ctrl Pts',(0.39991940378308,-1.,1.78598826347533));
#27305=CARTESIAN_POINT('Ctrl Pts',(0.39991940378308,1.,1.78598826347533));
#27306=CARTESIAN_POINT('Ctrl Pts',(0.403107976170441,-1.,1.80012077176221));
#27307=CARTESIAN_POINT('Ctrl Pts',(0.403107976170441,1.,1.80012077176221));
#27308=CARTESIAN_POINT('Ctrl Pts',(0.405933518411838,-1.,1.81223801813988));
#27309=CARTESIAN_POINT('Ctrl Pts',(0.405933518411838,1.,1.81223801813988));
#27310=CARTESIAN_POINT('Ctrl Pts',(0.408428948108533,-1.,1.8224702267854));
#27311=CARTESIAN_POINT('Ctrl Pts',(0.408428948108533,1.,1.8224702267854));
#27312=CARTESIAN_POINT('Ctrl Pts',(0.410641256301674,-1.,1.83100408895216));
#27313=CARTESIAN_POINT('Ctrl Pts',(0.410641256301674,1.,1.83100408895216));
#27314=CARTESIAN_POINT('Ctrl Pts',(0.412633125322161,-1.,1.83808953475839));
#27315=CARTESIAN_POINT('Ctrl Pts',(0.412633125322161,1.,1.83808953475839));
#27316=CARTESIAN_POINT('Ctrl Pts',(0.41448743825434,-1.,1.8440575707371));
#27317=CARTESIAN_POINT('Ctrl Pts',(0.41448743825434,1.,1.8440575707371));
#27318=CARTESIAN_POINT('Ctrl Pts',(0.416300022038864,-1.,1.84929312929882));
#27319=CARTESIAN_POINT('Ctrl Pts',(0.416300022038864,1.,1.84929312929882));
#27320=CARTESIAN_POINT('Ctrl Pts',(0.418164129143534,-1.,1.85417632856234));
#27321=CARTESIAN_POINT('Ctrl Pts',(0.418164129143534,1.,1.85417632856234));
#27322=CARTESIAN_POINT('Ctrl Pts',(0.420157287975619,-1.,1.85903281096686));
#27323=CARTESIAN_POINT('Ctrl Pts',(0.420157287975619,1.,1.85903281096686));
#27324=CARTESIAN_POINT('Ctrl Pts',(0.422327307418275,-1.,1.86408083334028));
#27325=CARTESIAN_POINT('Ctrl Pts',(0.422327307418275,1.,1.86408083334028));
#27326=CARTESIAN_POINT('Ctrl Pts',(0.424678177291358,-1.,1.86937803944323));
#27327=CARTESIAN_POINT('Ctrl Pts',(0.424678177291358,1.,1.86937803944323));
#27328=CARTESIAN_POINT('Ctrl Pts',(0.427183828519102,-1.,1.87486989291484));
#27329=CARTESIAN_POINT('Ctrl Pts',(0.427183828519102,1.,1.87486989291484));
#27330=CARTESIAN_POINT('Ctrl Pts',(0.429803062482344,-1.,1.88044229001832));
#27331=CARTESIAN_POINT('Ctrl Pts',(0.429803062482344,1.,1.88044229001832));
#27332=CARTESIAN_POINT('Ctrl Pts',(0.432493038548748,-1.,1.88596913666793));
#27333=CARTESIAN_POINT('Ctrl Pts',(0.432493038548748,1.,1.88596913666793));
#27334=CARTESIAN_POINT('Ctrl Pts',(0.435225660963383,-1.,1.89136993975504));
#27335=CARTESIAN_POINT('Ctrl Pts',(0.435225660963383,1.,1.89136993975504));
#27336=CARTESIAN_POINT('Ctrl Pts',(0.437995003948244,-1.,1.89663648956466));
#27337=CARTESIAN_POINT('Ctrl Pts',(0.437995003948244,1.,1.89663648956466));
#27338=CARTESIAN_POINT('Ctrl Pts',(0.440807833704038,-1.,1.90180124389086));
#27339=CARTESIAN_POINT('Ctrl Pts',(0.440807833704038,1.,1.90180124389086));
#27340=CARTESIAN_POINT('Ctrl Pts',(0.44367755684915,-1.,1.90691756144898));
#27341=CARTESIAN_POINT('Ctrl Pts',(0.44367755684915,1.,1.90691756144898));
#27342=CARTESIAN_POINT('Ctrl Pts',(0.446617343485711,-1.,1.9120369998112));
#27343=CARTESIAN_POINT('Ctrl Pts',(0.446617343485711,1.,1.9120369998112));
#27344=CARTESIAN_POINT('Ctrl Pts',(0.449632260106662,-1.,1.91718342555755));
#27345=CARTESIAN_POINT('Ctrl Pts',(0.449632260106662,1.,1.91718342555755));
#27346=CARTESIAN_POINT('Ctrl Pts',(0.452719478359432,-1.,1.92235380648502));
#27347=CARTESIAN_POINT('Ctrl Pts',(0.452719478359432,1.,1.92235380648502));
#27348=CARTESIAN_POINT('Ctrl Pts',(0.45587200517437,-1.,1.92753067150476));
#27349=CARTESIAN_POINT('Ctrl Pts',(0.45587200517437,1.,1.92753067150476));
#27350=CARTESIAN_POINT('Ctrl Pts',(0.459081234547926,-1.,1.93269066517934));
#27351=CARTESIAN_POINT('Ctrl Pts',(0.459081234547926,1.,1.93269066517934));
#27352=CARTESIAN_POINT('Ctrl Pts',(0.462340031009056,-1.,1.93781486640821));
#27353=CARTESIAN_POINT('Ctrl Pts',(0.462340031009056,1.,1.93781486640821));
#27354=CARTESIAN_POINT('Ctrl Pts',(0.46564546202603,-1.,1.9428979419619));
#27355=CARTESIAN_POINT('Ctrl Pts',(0.46564546202603,1.,1.9428979419619));
#27356=CARTESIAN_POINT('Ctrl Pts',(0.468997482913135,-1.,1.94794381136514));
#27357=CARTESIAN_POINT('Ctrl Pts',(0.468997482913135,1.,1.94794381136514));
#27358=CARTESIAN_POINT('Ctrl Pts',(0.472397672264072,-1.,1.95296148278133));
#27359=CARTESIAN_POINT('Ctrl Pts',(0.472397672264072,1.,1.95296148278133));
#27360=CARTESIAN_POINT('Ctrl Pts',(0.475848034683176,-1.,1.95796111148177));
#27361=CARTESIAN_POINT('Ctrl Pts',(0.475848034683176,1.,1.95796111148177));
#27362=CARTESIAN_POINT('Ctrl Pts',(0.479349583074855,-1.,1.96294933055943));
#27363=CARTESIAN_POINT('Ctrl Pts',(0.479349583074855,1.,1.96294933055943));
#27364=CARTESIAN_POINT('Ctrl Pts',(0.48290166212069,-1.,1.96792703422362));
#27365=CARTESIAN_POINT('Ctrl Pts',(0.48290166212069,1.,1.96792703422362));
#27366=CARTESIAN_POINT('Ctrl Pts',(0.486502692907658,-1.,1.97289186263272));
#27367=CARTESIAN_POINT('Ctrl Pts',(0.486502692907658,1.,1.97289186263272));
#27368=CARTESIAN_POINT('Ctrl Pts',(0.490150627860952,-1.,1.97783973019229));
#27369=CARTESIAN_POINT('Ctrl Pts',(0.490150627860952,1.,1.97783973019229));
#27370=CARTESIAN_POINT('Ctrl Pts',(0.493843476541494,-1.,1.98276658761821));
#27371=CARTESIAN_POINT('Ctrl Pts',(0.493843476541494,1.,1.98276658761821));
#27372=CARTESIAN_POINT('Ctrl Pts',(0.497579909545574,-1.,1.98767044752932));
#27373=CARTESIAN_POINT('Ctrl Pts',(0.497579909545574,1.,1.98767044752932));
#27374=CARTESIAN_POINT('Ctrl Pts',(0.501359287727146,-1.,1.99255149126155));
#27375=CARTESIAN_POINT('Ctrl Pts',(0.501359287727146,1.,1.99255149126155));
#27376=CARTESIAN_POINT('Ctrl Pts',(0.505181361323026,-1.,1.99741107463572));
#27377=CARTESIAN_POINT('Ctrl Pts',(0.505181361323026,1.,1.99741107463572));
#27378=CARTESIAN_POINT('Ctrl Pts',(0.509046069886157,-1.,2.00225107134734));
#27379=CARTESIAN_POINT('Ctrl Pts',(0.509046069886157,1.,2.00225107134734));
#27380=CARTESIAN_POINT('Ctrl Pts',(0.512953306961792,-1.,2.00707309946949));
#27381=CARTESIAN_POINT('Ctrl Pts',(0.512953306961792,1.,2.00707309946949));
#27382=CARTESIAN_POINT('Ctrl Pts',(0.516902681728687,-1.,2.01187773939242));
#27383=CARTESIAN_POINT('Ctrl Pts',(0.516902681728687,1.,2.01187773939242));
#27384=CARTESIAN_POINT('Ctrl Pts',(0.52089359039937,-1.,2.01666477917286));
#27385=CARTESIAN_POINT('Ctrl Pts',(0.52089359039937,1.,2.01666477917286));
#27386=CARTESIAN_POINT('Ctrl Pts',(0.524925318333476,-1.,2.02143356304698));
#27387=CARTESIAN_POINT('Ctrl Pts',(0.524925318333476,1.,2.02143356304698));
#27388=CARTESIAN_POINT('Ctrl Pts',(0.528997127241914,-1.,2.0261832908329));
#27389=CARTESIAN_POINT('Ctrl Pts',(0.528997127241914,1.,2.0261832908329));
#27390=CARTESIAN_POINT('Ctrl Pts',(0.533108355132976,-1.,2.03091336214426));
#27391=CARTESIAN_POINT('Ctrl Pts',(0.533108355132976,1.,2.03091336214426));
#27392=CARTESIAN_POINT('Ctrl Pts',(0.537258489833262,-1.,2.03562362954037));
#27393=CARTESIAN_POINT('Ctrl Pts',(0.537258489833262,1.,2.03562362954037));
#27394=CARTESIAN_POINT('Ctrl Pts',(0.541447120615659,-1.,2.04031422690527));
#27395=CARTESIAN_POINT('Ctrl Pts',(0.541447120615659,1.,2.04031422690527));
#27396=CARTESIAN_POINT('Ctrl Pts',(0.54567390381743,-1.,2.04498544714588));
#27397=CARTESIAN_POINT('Ctrl Pts',(0.54567390381743,1.,2.04498544714588));
#27398=CARTESIAN_POINT('Ctrl Pts',(0.549938525150295,-1.,2.04963761077958));
#27399=CARTESIAN_POINT('Ctrl Pts',(0.549938525150295,1.,2.04963761077958));
#27400=CARTESIAN_POINT('Ctrl Pts',(0.554240657463906,-1.,2.05427091604413));
#27401=CARTESIAN_POINT('Ctrl Pts',(0.554240657463906,1.,2.05427091604413));
#27402=CARTESIAN_POINT('Ctrl Pts',(0.558579940185151,-1.,2.05888537756462));
#27403=CARTESIAN_POINT('Ctrl Pts',(0.558579940185151,1.,2.05888537756462));
#27404=CARTESIAN_POINT('Ctrl Pts',(0.562955993082261,-1.,2.06348090160589));
#27405=CARTESIAN_POINT('Ctrl Pts',(0.562955993082261,1.,2.06348090160589));
#27406=CARTESIAN_POINT('Ctrl Pts',(0.567368421181087,-1.,2.06805732997334));
#27407=CARTESIAN_POINT('Ctrl Pts',(0.567368421181087,1.,2.06805732997334));
#27408=CARTESIAN_POINT('Ctrl Pts',(0.571816823242602,-1.,2.07261449292824));
#27409=CARTESIAN_POINT('Ctrl Pts',(0.571816823242602,1.,2.07261449292824));
#27410=CARTESIAN_POINT('Ctrl Pts',(0.576300797416844,-1.,2.07715226767559));
#27411=CARTESIAN_POINT('Ctrl Pts',(0.576300797416844,1.,2.07715226767559));
#27412=CARTESIAN_POINT('Ctrl Pts',(0.580819952108063,-1.,2.08167059018418));
#27413=CARTESIAN_POINT('Ctrl Pts',(0.580819952108063,1.,2.08167059018418));
#27414=CARTESIAN_POINT('Ctrl Pts',(0.585373918991617,-1.,2.08616943727951));
#27415=CARTESIAN_POINT('Ctrl Pts',(0.585373918991617,1.,2.08616943727951));
#27416=CARTESIAN_POINT('Ctrl Pts',(0.589962365403406,-1.,2.09064881812129));
#27417=CARTESIAN_POINT('Ctrl Pts',(0.589962365403406,1.,2.09064881812129));
#27418=CARTESIAN_POINT('Ctrl Pts',(0.594585006052162,-1.,2.0951087622027));
#27419=CARTESIAN_POINT('Ctrl Pts',(0.594585006052162,1.,2.0951087622027));
#27420=CARTESIAN_POINT('Ctrl Pts',(0.599241616420533,-1.,2.0995493086477));
#27421=CARTESIAN_POINT('Ctrl Pts',(0.599241616420533,1.,2.0995493086477));
#27422=CARTESIAN_POINT('Ctrl Pts',(0.60393203073603,-1.,2.10397049886949));
#27423=CARTESIAN_POINT('Ctrl Pts',(0.60393203073603,1.,2.10397049886949));
#27424=CARTESIAN_POINT('Ctrl Pts',(0.607711315454876,-1.,2.1074919961518));
#27425=CARTESIAN_POINT('Ctrl Pts',(0.607711315454876,1.,2.1074919961518));
#27426=CARTESIAN_POINT('Ctrl Pts',(0.610560911689898,-1.,2.11012443807238));
#27427=CARTESIAN_POINT('Ctrl Pts',(0.610560911689898,1.,2.11012443807238));
#27428=CARTESIAN_POINT('Ctrl Pts',(0.6124673655618,-1.,2.11187554259986));
#27429=CARTESIAN_POINT('Ctrl Pts',(0.6124673655618,1.,2.11187554259986));
#27430=CARTESIAN_POINT('Ctrl Pts',(0.61342227326009,-1.,2.11275013067528));
#27431=CARTESIAN_POINT('Ctrl Pts',(0.61342227326009,1.,2.11275013067528));
#27432=CARTESIAN_POINT('',(0.383122945602004,1.,1.7075470150345));
#27433=CARTESIAN_POINT('Ctrl Pts',(0.383122945602004,1.,1.7075470150345));
#27434=CARTESIAN_POINT('Ctrl Pts',(0.384119047315541,1.,1.71231062891958));
#27435=CARTESIAN_POINT('Ctrl Pts',(0.38607079032701,1.,1.72162022246158));
#27436=CARTESIAN_POINT('Ctrl Pts',(0.388877023509191,1.,1.7349317097561));
#27437=CARTESIAN_POINT('Ctrl Pts',(0.392375812294307,1.,1.75137405313962));
#27438=CARTESIAN_POINT('Ctrl Pts',(0.39634619612042,1.,1.7697556004756));
#27439=CARTESIAN_POINT('Ctrl Pts',(0.39991940378308,1.,1.78598826347533));
#27440=CARTESIAN_POINT('Ctrl Pts',(0.403107976170441,1.,1.80012077176221));
#27441=CARTESIAN_POINT('Ctrl Pts',(0.405933518411838,1.,1.81223801813988));
#27442=CARTESIAN_POINT('Ctrl Pts',(0.408428948108533,1.,1.8224702267854));
#27443=CARTESIAN_POINT('Ctrl Pts',(0.410641256301674,1.,1.83100408895216));
#27444=CARTESIAN_POINT('Ctrl Pts',(0.412633125322161,1.,1.83808953475839));
#27445=CARTESIAN_POINT('Ctrl Pts',(0.41448743825434,1.,1.8440575707371));
#27446=CARTESIAN_POINT('Ctrl Pts',(0.416300022038864,1.,1.84929312929882));
#27447=CARTESIAN_POINT('Ctrl Pts',(0.418164129143534,1.,1.85417632856234));
#27448=CARTESIAN_POINT('Ctrl Pts',(0.420157287975619,1.,1.85903281096686));
#27449=CARTESIAN_POINT('Ctrl Pts',(0.422327307418275,1.,1.86408083334028));
#27450=CARTESIAN_POINT('Ctrl Pts',(0.424678177291358,1.,1.86937803944323));
#27451=CARTESIAN_POINT('Ctrl Pts',(0.427183828519102,1.,1.87486989291484));
#27452=CARTESIAN_POINT('Ctrl Pts',(0.429803062482344,1.,1.88044229001832));
#27453=CARTESIAN_POINT('Ctrl Pts',(0.432493038548748,1.,1.88596913666793));
#27454=CARTESIAN_POINT('Ctrl Pts',(0.435225660963383,1.,1.89136993975504));
#27455=CARTESIAN_POINT('Ctrl Pts',(0.437995003948244,1.,1.89663648956466));
#27456=CARTESIAN_POINT('Ctrl Pts',(0.440807833704038,1.,1.90180124389086));
#27457=CARTESIAN_POINT('Ctrl Pts',(0.44367755684915,1.,1.90691756144898));
#27458=CARTESIAN_POINT('Ctrl Pts',(0.446617343485711,1.,1.9120369998112));
#27459=CARTESIAN_POINT('Ctrl Pts',(0.449632260106662,1.,1.91718342555755));
#27460=CARTESIAN_POINT('Ctrl Pts',(0.452719478359432,1.,1.92235380648502));
#27461=CARTESIAN_POINT('Ctrl Pts',(0.45587200517437,1.,1.92753067150476));
#27462=CARTESIAN_POINT('Ctrl Pts',(0.459081234547926,1.,1.93269066517934));
#27463=CARTESIAN_POINT('Ctrl Pts',(0.462340031009056,1.,1.93781486640821));
#27464=CARTESIAN_POINT('Ctrl Pts',(0.46564546202603,1.,1.9428979419619));
#27465=CARTESIAN_POINT('Ctrl Pts',(0.468997482913135,1.,1.94794381136514));
#27466=CARTESIAN_POINT('Ctrl Pts',(0.472397672264072,1.,1.95296148278133));
#27467=CARTESIAN_POINT('Ctrl Pts',(0.475848034683176,1.,1.95796111148177));
#27468=CARTESIAN_POINT('Ctrl Pts',(0.479349583074855,1.,1.96294933055943));
#27469=CARTESIAN_POINT('Ctrl Pts',(0.48290166212069,1.,1.96792703422362));
#27470=CARTESIAN_POINT('Ctrl Pts',(0.486502692907658,1.,1.97289186263272));
#27471=CARTESIAN_POINT('Ctrl Pts',(0.490150627860952,1.,1.97783973019229));
#27472=CARTESIAN_POINT('Ctrl Pts',(0.493843476541494,1.,1.98276658761821));
#27473=CARTESIAN_POINT('Ctrl Pts',(0.497579909545574,1.,1.98767044752932));
#27474=CARTESIAN_POINT('Ctrl Pts',(0.501359287727146,1.,1.99255149126155));
#27475=CARTESIAN_POINT('Ctrl Pts',(0.505181361323026,1.,1.99741107463572));
#27476=CARTESIAN_POINT('Ctrl Pts',(0.509046069886157,1.,2.00225107134734));
#27477=CARTESIAN_POINT('Ctrl Pts',(0.512953306961792,1.,2.00707309946949));
#27478=CARTESIAN_POINT('Ctrl Pts',(0.516902681728687,1.,2.01187773939242));
#27479=CARTESIAN_POINT('Ctrl Pts',(0.52089359039937,1.,2.01666477917286));
#27480=CARTESIAN_POINT('Ctrl Pts',(0.524925318333476,1.,2.02143356304698));
#27481=CARTESIAN_POINT('Ctrl Pts',(0.528997127241914,1.,2.0261832908329));
#27482=CARTESIAN_POINT('Ctrl Pts',(0.533108355132976,1.,2.03091336214426));
#27483=CARTESIAN_POINT('Ctrl Pts',(0.537258489833262,1.,2.03562362954037));
#27484=CARTESIAN_POINT('Ctrl Pts',(0.541447120615659,1.,2.04031422690527));
#27485=CARTESIAN_POINT('Ctrl Pts',(0.54567390381743,1.,2.04498544714588));
#27486=CARTESIAN_POINT('Ctrl Pts',(0.549938525150295,1.,2.04963761077958));
#27487=CARTESIAN_POINT('Ctrl Pts',(0.554240657463906,1.,2.05427091604413));
#27488=CARTESIAN_POINT('Ctrl Pts',(0.558579940185151,1.,2.05888537756462));
#27489=CARTESIAN_POINT('Ctrl Pts',(0.562955993082261,1.,2.06348090160589));
#27490=CARTESIAN_POINT('Ctrl Pts',(0.567368421181087,1.,2.06805732997334));
#27491=CARTESIAN_POINT('Ctrl Pts',(0.571816823242602,1.,2.07261449292824));
#27492=CARTESIAN_POINT('Ctrl Pts',(0.576300797416844,1.,2.07715226767559));
#27493=CARTESIAN_POINT('Ctrl Pts',(0.580819952108063,1.,2.08167059018418));
#27494=CARTESIAN_POINT('Ctrl Pts',(0.585373918991617,1.,2.08616943727951));
#27495=CARTESIAN_POINT('Ctrl Pts',(0.589962365403406,1.,2.09064881812129));
#27496=CARTESIAN_POINT('Ctrl Pts',(0.594585006052162,1.,2.0951087622027));
#27497=CARTESIAN_POINT('Ctrl Pts',(0.599241616420533,1.,2.0995493086477));
#27498=CARTESIAN_POINT('Ctrl Pts',(0.60393203073603,1.,2.10397049886949));
#27499=CARTESIAN_POINT('Ctrl Pts',(0.607711315454876,1.,2.1074919961518));
#27500=CARTESIAN_POINT('Ctrl Pts',(0.610560911689898,1.,2.11012443807238));
#27501=CARTESIAN_POINT('Ctrl Pts',(0.6124673655618,1.,2.11187554259986));
#27502=CARTESIAN_POINT('Ctrl Pts',(0.61342227326009,1.,2.11275013067528));
#27503=CARTESIAN_POINT('',(0.383122945602003,0.,1.7075470150345));
#27504=CARTESIAN_POINT('Origin',(0.,0.,0.));
#27505=CARTESIAN_POINT('',(0.163289472382896,1.,1.74236521665491));
#27506=CARTESIAN_POINT('Origin',(0.,1.,0.));
#27507=CARTESIAN_POINT('',(0.163289472382896,0.,1.74236521665491));
#27508=CARTESIAN_POINT('Ctrl Pts',(0.0694764450219578,-1.,2.19890268624765));
#27509=CARTESIAN_POINT('Ctrl Pts',(0.0694764450219578,1.,2.19890268624765));
#27510=CARTESIAN_POINT('Ctrl Pts',(0.0701143536325487,-1.,2.19777582085423));
#27511=CARTESIAN_POINT('Ctrl Pts',(0.0701143536325487,1.,2.19777582085423));
#27512=CARTESIAN_POINT('Ctrl Pts',(0.0713863779526151,-1.,2.19552129484002));
#27513=CARTESIAN_POINT('Ctrl Pts',(0.0713863779526151,1.,2.19552129484002));
#27514=CARTESIAN_POINT('Ctrl Pts',(0.0732830357306722,-1.,2.19213712013662));
#27515=CARTESIAN_POINT('Ctrl Pts',(0.0732830357306722,1.,2.19213712013662));
#27516=CARTESIAN_POINT('Ctrl Pts',(0.0757891465836145,-1.,2.1876201139953));
#27517=CARTESIAN_POINT('Ctrl Pts',(0.0757891465836145,1.,2.1876201139953));
#27518=CARTESIAN_POINT('Ctrl Pts',(0.078883772768524,-1.,2.18196589448887));
#27519=CARTESIAN_POINT('Ctrl Pts',(0.078883772768524,1.,2.18196589448887));
#27520=CARTESIAN_POINT('Ctrl Pts',(0.0819402680872763,-1.,2.176303712113));
#27521=CARTESIAN_POINT('Ctrl Pts',(0.0819402680872763,1.,2.176303712113));
#27522=CARTESIAN_POINT('Ctrl Pts',(0.084958462083537,-1.,2.17063357870952));
#27523=CARTESIAN_POINT('Ctrl Pts',(0.084958462083537,1.,2.17063357870952));
#27524=CARTESIAN_POINT('Ctrl Pts',(0.087938129138692,-1.,2.16495552645014));
#27525=CARTESIAN_POINT('Ctrl Pts',(0.087938129138692,1.,2.16495552645014));
#27526=CARTESIAN_POINT('Ctrl Pts',(0.0908789888107263,-1.,2.15926961544516));
#27527=CARTESIAN_POINT('Ctrl Pts',(0.0908789888107263,1.,2.15926961544516));
#27528=CARTESIAN_POINT('Ctrl Pts',(0.0937807218867641,-1.,2.1535759397817));
#27529=CARTESIAN_POINT('Ctrl Pts',(0.0937807218867641,1.,2.1535759397817));
#27530=CARTESIAN_POINT('Ctrl Pts',(0.0966429852305456,-1.,2.14787463531795));
#27531=CARTESIAN_POINT('Ctrl Pts',(0.0966429852305456,1.,2.14787463531795));
#27532=CARTESIAN_POINT('Ctrl Pts',(0.0994654261990913,-1.,2.14216588396025));
#27533=CARTESIAN_POINT('Ctrl Pts',(0.0994654261990913,1.,2.14216588396025));
#27534=CARTESIAN_POINT('Ctrl Pts',(0.1022477005561,-1.,2.13644992667165));
#27535=CARTESIAN_POINT('Ctrl Pts',(0.1022477005561,1.,2.13644992667165));
#27536=CARTESIAN_POINT('Ctrl Pts',(0.104989479152739,-1.,2.13072704887293));
#27537=CARTESIAN_POINT('Ctrl Pts',(0.104989479152739,1.,2.13072704887293));
#27538=CARTESIAN_POINT('Ctrl Pts',(0.10769043523109,-1.,2.12499752307));
#27539=CARTESIAN_POINT('Ctrl Pts',(0.10769043523109,1.,2.12499752307));
#27540=CARTESIAN_POINT('Ctrl Pts',(0.110350236135025,-1.,2.11926155590865));
#27541=CARTESIAN_POINT('Ctrl Pts',(0.110350236135025,1.,2.11926155590865));
#27542=CARTESIAN_POINT('Ctrl Pts',(0.112968534419737,-1.,2.11351924490306));
#27543=CARTESIAN_POINT('Ctrl Pts',(0.112968534419737,1.,2.11351924490306));
#27544=CARTESIAN_POINT('Ctrl Pts',(0.115544957687926,-1.,2.10777050261309));
#27545=CARTESIAN_POINT('Ctrl Pts',(0.115544957687926,1.,2.10777050261309));
#27546=CARTESIAN_POINT('Ctrl Pts',(0.118079107988355,-1.,2.102015121329));
#27547=CARTESIAN_POINT('Ctrl Pts',(0.118079107988355,1.,2.102015121329));
#27548=CARTESIAN_POINT('Ctrl Pts',(0.120570567965122,-1.,2.0962529286773));
#27549=CARTESIAN_POINT('Ctrl Pts',(0.120570567965122,1.,2.0962529286773));
#27550=CARTESIAN_POINT('Ctrl Pts',(0.123018905621083,-1.,2.09048392424825));
#27551=CARTESIAN_POINT('Ctrl Pts',(0.123018905621083,1.,2.09048392424825));
#27552=CARTESIAN_POINT('Ctrl Pts',(0.125423679412061,-1.,2.08470840653643));
#27553=CARTESIAN_POINT('Ctrl Pts',(0.125423679412061,1.,2.08470840653643));
#27554=CARTESIAN_POINT('Ctrl Pts',(0.12778444527612,-1.,2.07892715110987));
#27555=CARTESIAN_POINT('Ctrl Pts',(0.12778444527612,1.,2.07892715110987));
#27556=CARTESIAN_POINT('Ctrl Pts',(0.130100748328403,-1.,2.07314114713063));
#27557=CARTESIAN_POINT('Ctrl Pts',(0.130100748328403,1.,2.07314114713063));
#27558=CARTESIAN_POINT('Ctrl Pts',(0.13237211154771,-1.,2.06735123910326));
#27559=CARTESIAN_POINT('Ctrl Pts',(0.13237211154771,1.,2.06735123910326));
#27560=CARTESIAN_POINT('Ctrl Pts',(0.134598026192106,-1.,2.06155781517842));
#27561=CARTESIAN_POINT('Ctrl Pts',(0.134598026192106,1.,2.06155781517842));
#27562=CARTESIAN_POINT('Ctrl Pts',(0.136777941218043,-1.,2.05576044414264));
#27563=CARTESIAN_POINT('Ctrl Pts',(0.136777941218043,1.,2.05576044414264));
#27564=CARTESIAN_POINT('Ctrl Pts',(0.138911255368966,-1.,2.04995762001328));
#27565=CARTESIAN_POINT('Ctrl Pts',(0.138911255368966,1.,2.04995762001328));
#27566=CARTESIAN_POINT('Ctrl Pts',(0.140997332152546,-1.,2.04414757947916));
#27567=CARTESIAN_POINT('Ctrl Pts',(0.140997332152546,1.,2.04414757947916));
#27568=CARTESIAN_POINT('Ctrl Pts',(0.143035515058208,-1.,2.03832911025912));
#27569=CARTESIAN_POINT('Ctrl Pts',(0.143035515058208,1.,2.03832911025912));
#27570=CARTESIAN_POINT('Ctrl Pts',(0.145025140186057,-1.,2.03250223739942));
#27571=CARTESIAN_POINT('Ctrl Pts',(0.145025140186057,1.,2.03250223739942));
#27572=CARTESIAN_POINT('Ctrl Pts',(0.146965557332583,-1.,2.02666926182017));
#27573=CARTESIAN_POINT('Ctrl Pts',(0.146965557332583,1.,2.02666926182017));
#27574=CARTESIAN_POINT('Ctrl Pts',(0.148856124775337,-1.,2.02083464969894));
#27575=CARTESIAN_POINT('Ctrl Pts',(0.148856124775337,1.,2.02083464969894));
#27576=CARTESIAN_POINT('Ctrl Pts',(0.150696157673078,-1.,2.01500291940238));
#27577=CARTESIAN_POINT('Ctrl Pts',(0.150696157673078,1.,2.01500291940238));
#27578=CARTESIAN_POINT('Ctrl Pts',(0.152484883621449,-1.,2.00917680318424));
#27579=CARTESIAN_POINT('Ctrl Pts',(0.152484883621449,1.,2.00917680318424));
#27580=CARTESIAN_POINT('Ctrl Pts',(0.154221403049722,-1.,2.00335565310543));
#27581=CARTESIAN_POINT('Ctrl Pts',(0.154221403049722,1.,2.00335565310543));
#27582=CARTESIAN_POINT('Ctrl Pts',(0.155904629548783,-1.,1.99753284771497));
#27583=CARTESIAN_POINT('Ctrl Pts',(0.155904629548783,1.,1.99753284771497));
#27584=CARTESIAN_POINT('Ctrl Pts',(0.157533331459227,-1.,1.99169810931908));
#27585=CARTESIAN_POINT('Ctrl Pts',(0.157533331459227,1.,1.99169810931908));
#27586=CARTESIAN_POINT('Ctrl Pts',(0.159106226437299,-1.,1.98584238283292));
#27587=CARTESIAN_POINT('Ctrl Pts',(0.159106226437299,1.,1.98584238283292));
#27588=CARTESIAN_POINT('Ctrl Pts',(0.160622060784611,-1.,1.97996195437559));
#27589=CARTESIAN_POINT('Ctrl Pts',(0.160622060784611,1.,1.97996195437559));
#27590=CARTESIAN_POINT('Ctrl Pts',(0.162079693556288,-1.,1.97406280235188));
#27591=CARTESIAN_POINT('Ctrl Pts',(0.162079693556288,1.,1.97406280235188));
#27592=CARTESIAN_POINT('Ctrl Pts',(0.163478185457734,-1.,1.96816512677967));
#27593=CARTESIAN_POINT('Ctrl Pts',(0.163478185457734,1.,1.96816512677967));
#27594=CARTESIAN_POINT('Ctrl Pts',(0.164816568920269,-1.,1.96229379940136));
#27595=CARTESIAN_POINT('Ctrl Pts',(0.164816568920269,1.,1.96229379940136));
#27596=CARTESIAN_POINT('Ctrl Pts',(0.166093592002812,-1.,1.9564675971873));
#27597=CARTESIAN_POINT('Ctrl Pts',(0.166093592002812,1.,1.9564675971873));
#27598=CARTESIAN_POINT('Ctrl Pts',(0.167307501784475,-1.,1.95069027794294));
#27599=CARTESIAN_POINT('Ctrl Pts',(0.167307501784475,1.,1.95069027794294));
#27600=CARTESIAN_POINT('Ctrl Pts',(0.168455741607556,-1.,1.94493757756931));
#27601=CARTESIAN_POINT('Ctrl Pts',(0.168455741607556,1.,1.94493757756931));
#27602=CARTESIAN_POINT('Ctrl Pts',(0.16953490481749,-1.,1.93915639211581));
#27603=CARTESIAN_POINT('Ctrl Pts',(0.16953490481749,1.,1.93915639211581));
#27604=CARTESIAN_POINT('Ctrl Pts',(0.170541253116201,-1.,1.93329183155539));
#27605=CARTESIAN_POINT('Ctrl Pts',(0.170541253116201,1.,1.93329183155539));
#27606=CARTESIAN_POINT('Ctrl Pts',(0.171471191532988,-1.,1.92731093582036));
#27607=CARTESIAN_POINT('Ctrl Pts',(0.171471191532988,1.,1.92731093582036));
#27608=CARTESIAN_POINT('Ctrl Pts',(0.172321621259513,-1.,1.9212233439798));
#27609=CARTESIAN_POINT('Ctrl Pts',(0.172321621259513,1.,1.9212233439798));
#27610=CARTESIAN_POINT('Ctrl Pts',(0.173090695383496,-1.,1.91511429159527));
#27611=CARTESIAN_POINT('Ctrl Pts',(0.173090695383496,1.,1.91511429159527));
#27612=CARTESIAN_POINT('Ctrl Pts',(0.173776635257816,-1.,1.90911693975267));
#27613=CARTESIAN_POINT('Ctrl Pts',(0.173776635257816,1.,1.90911693975267));
#27614=CARTESIAN_POINT('Ctrl Pts',(0.174375518661085,-1.,1.90335253862834));
#27615=CARTESIAN_POINT('Ctrl Pts',(0.174375518661085,1.,1.90335253862834));
#27616=CARTESIAN_POINT('Ctrl Pts',(0.174879405091263,-1.,1.89788101117132));
#27617=CARTESIAN_POINT('Ctrl Pts',(0.174879405091263,1.,1.89788101117132));
#27618=CARTESIAN_POINT('Ctrl Pts',(0.175274276190844,-1.,1.892646301985));
#27619=CARTESIAN_POINT('Ctrl Pts',(0.175274276190844,1.,1.892646301985));
#27620=CARTESIAN_POINT('Ctrl Pts',(0.175538155840648,-1.,1.88742606273259));
#27621=CARTESIAN_POINT('Ctrl Pts',(0.175538155840648,1.,1.88742606273259));
#27622=CARTESIAN_POINT('Ctrl Pts',(0.175644148889698,-1.,1.88188663145367));
#27623=CARTESIAN_POINT('Ctrl Pts',(0.175644148889698,1.,1.88188663145367));
#27624=CARTESIAN_POINT('Ctrl Pts',(0.175563480746485,-1.,1.87563767773588));
#27625=CARTESIAN_POINT('Ctrl Pts',(0.175563480746485,1.,1.87563767773588));
#27626=CARTESIAN_POINT('Ctrl Pts',(0.175268337590757,-1.,1.86828349694799));
#27627=CARTESIAN_POINT('Ctrl Pts',(0.175268337590757,1.,1.86828349694799));
#27628=CARTESIAN_POINT('Ctrl Pts',(0.17473525927603,-1.,1.85948367088837));
#27629=CARTESIAN_POINT('Ctrl Pts',(0.17473525927603,1.,1.85948367088837));
#27630=CARTESIAN_POINT('Ctrl Pts',(0.173946627587731,-1.,1.8489811319852));
#27631=CARTESIAN_POINT('Ctrl Pts',(0.173946627587731,1.,1.8489811319852));
#27632=CARTESIAN_POINT('Ctrl Pts',(0.1728894428919,-1.,1.83658380527692));
#27633=CARTESIAN_POINT('Ctrl Pts',(0.1728894428919,1.,1.83658380527692));
#27634=CARTESIAN_POINT('Ctrl Pts',(0.171554770204119,-1.,1.82215766811545));
#27635=CARTESIAN_POINT('Ctrl Pts',(0.171554770204119,1.,1.82215766811545));
#27636=CARTESIAN_POINT('Ctrl Pts',(0.169936923904608,-1.,1.80561530629706));
#27637=CARTESIAN_POINT('Ctrl Pts',(0.169936923904608,1.,1.80561530629706));
#27638=CARTESIAN_POINT('Ctrl Pts',(0.168032772805197,-1.,1.7869064998507));
#27639=CARTESIAN_POINT('Ctrl Pts',(0.168032772805197,1.,1.7869064998507));
#27640=CARTESIAN_POINT('Ctrl Pts',(0.1662793551464,-1.,1.77018771684844));
#27641=CARTESIAN_POINT('Ctrl Pts',(0.1662793551464,1.,1.77018771684844));
#27642=CARTESIAN_POINT('Ctrl Pts',(0.164834765707158,-1.,1.75666056638427));
#27643=CARTESIAN_POINT('Ctrl Pts',(0.164834765707158,1.,1.75666056638427));
#27644=CARTESIAN_POINT('Ctrl Pts',(0.163814161002002,-1.,1.7472034950333));
#27645=CARTESIAN_POINT('Ctrl Pts',(0.163814161002002,1.,1.7472034950333));
#27646=CARTESIAN_POINT('Ctrl Pts',(0.163289472382896,-1.,1.74236521665491));
#27647=CARTESIAN_POINT('Ctrl Pts',(0.163289472382896,1.,1.74236521665491));
#27648=CARTESIAN_POINT('',(0.0694764450219578,1.,2.19890268624765));
#27649=CARTESIAN_POINT('Ctrl Pts',(0.0694764450219578,1.,2.19890268624765));
#27650=CARTESIAN_POINT('Ctrl Pts',(0.0701143536325487,1.,2.19777582085423));
#27651=CARTESIAN_POINT('Ctrl Pts',(0.0713863779526151,1.,2.19552129484002));
#27652=CARTESIAN_POINT('Ctrl Pts',(0.0732830357306722,1.,2.19213712013662));
#27653=CARTESIAN_POINT('Ctrl Pts',(0.0757891465836145,1.,2.1876201139953));
#27654=CARTESIAN_POINT('Ctrl Pts',(0.078883772768524,1.,2.18196589448887));
#27655=CARTESIAN_POINT('Ctrl Pts',(0.0819402680872763,1.,2.176303712113));
#27656=CARTESIAN_POINT('Ctrl Pts',(0.084958462083537,1.,2.17063357870952));
#27657=CARTESIAN_POINT('Ctrl Pts',(0.087938129138692,1.,2.16495552645014));
#27658=CARTESIAN_POINT('Ctrl Pts',(0.0908789888107263,1.,2.15926961544516));
#27659=CARTESIAN_POINT('Ctrl Pts',(0.0937807218867641,1.,2.1535759397817));
#27660=CARTESIAN_POINT('Ctrl Pts',(0.0966429852305456,1.,2.14787463531795));
#27661=CARTESIAN_POINT('Ctrl Pts',(0.0994654261990913,1.,2.14216588396025));
#27662=CARTESIAN_POINT('Ctrl Pts',(0.1022477005561,1.,2.13644992667165));
#27663=CARTESIAN_POINT('Ctrl Pts',(0.104989479152739,1.,2.13072704887293));
#27664=CARTESIAN_POINT('Ctrl Pts',(0.10769043523109,1.,2.12499752307));
#27665=CARTESIAN_POINT('Ctrl Pts',(0.110350236135025,1.,2.11926155590865));
#27666=CARTESIAN_POINT('Ctrl Pts',(0.112968534419737,1.,2.11351924490306));
#27667=CARTESIAN_POINT('Ctrl Pts',(0.115544957687926,1.,2.10777050261309));
#27668=CARTESIAN_POINT('Ctrl Pts',(0.118079107988355,1.,2.102015121329));
#27669=CARTESIAN_POINT('Ctrl Pts',(0.120570567965122,1.,2.0962529286773));
#27670=CARTESIAN_POINT('Ctrl Pts',(0.123018905621083,1.,2.09048392424825));
#27671=CARTESIAN_POINT('Ctrl Pts',(0.125423679412061,1.,2.08470840653643));
#27672=CARTESIAN_POINT('Ctrl Pts',(0.12778444527612,1.,2.07892715110987));
#27673=CARTESIAN_POINT('Ctrl Pts',(0.130100748328403,1.,2.07314114713063));
#27674=CARTESIAN_POINT('Ctrl Pts',(0.13237211154771,1.,2.06735123910326));
#27675=CARTESIAN_POINT('Ctrl Pts',(0.134598026192106,1.,2.06155781517842));
#27676=CARTESIAN_POINT('Ctrl Pts',(0.136777941218043,1.,2.05576044414264));
#27677=CARTESIAN_POINT('Ctrl Pts',(0.138911255368966,1.,2.04995762001328));
#27678=CARTESIAN_POINT('Ctrl Pts',(0.140997332152546,1.,2.04414757947916));
#27679=CARTESIAN_POINT('Ctrl Pts',(0.143035515058208,1.,2.03832911025912));
#27680=CARTESIAN_POINT('Ctrl Pts',(0.145025140186057,1.,2.03250223739942));
#27681=CARTESIAN_POINT('Ctrl Pts',(0.146965557332583,1.,2.02666926182017));
#27682=CARTESIAN_POINT('Ctrl Pts',(0.148856124775337,1.,2.02083464969894));
#27683=CARTESIAN_POINT('Ctrl Pts',(0.150696157673078,1.,2.01500291940238));
#27684=CARTESIAN_POINT('Ctrl Pts',(0.152484883621449,1.,2.00917680318424));
#27685=CARTESIAN_POINT('Ctrl Pts',(0.154221403049722,1.,2.00335565310543));
#27686=CARTESIAN_POINT('Ctrl Pts',(0.155904629548783,1.,1.99753284771497));
#27687=CARTESIAN_POINT('Ctrl Pts',(0.157533331459227,1.,1.99169810931908));
#27688=CARTESIAN_POINT('Ctrl Pts',(0.159106226437299,1.,1.98584238283292));
#27689=CARTESIAN_POINT('Ctrl Pts',(0.160622060784611,1.,1.97996195437559));
#27690=CARTESIAN_POINT('Ctrl Pts',(0.162079693556288,1.,1.97406280235188));
#27691=CARTESIAN_POINT('Ctrl Pts',(0.163478185457734,1.,1.96816512677967));
#27692=CARTESIAN_POINT('Ctrl Pts',(0.164816568920269,1.,1.96229379940136));
#27693=CARTESIAN_POINT('Ctrl Pts',(0.166093592002812,1.,1.9564675971873));
#27694=CARTESIAN_POINT('Ctrl Pts',(0.167307501784475,1.,1.95069027794294));
#27695=CARTESIAN_POINT('Ctrl Pts',(0.168455741607556,1.,1.94493757756931));
#27696=CARTESIAN_POINT('Ctrl Pts',(0.16953490481749,1.,1.93915639211581));
#27697=CARTESIAN_POINT('Ctrl Pts',(0.170541253116201,1.,1.93329183155539));
#27698=CARTESIAN_POINT('Ctrl Pts',(0.171471191532988,1.,1.92731093582036));
#27699=CARTESIAN_POINT('Ctrl Pts',(0.172321621259513,1.,1.9212233439798));
#27700=CARTESIAN_POINT('Ctrl Pts',(0.173090695383496,1.,1.91511429159527));
#27701=CARTESIAN_POINT('Ctrl Pts',(0.173776635257816,1.,1.90911693975267));
#27702=CARTESIAN_POINT('Ctrl Pts',(0.174375518661085,1.,1.90335253862834));
#27703=CARTESIAN_POINT('Ctrl Pts',(0.174879405091263,1.,1.89788101117132));
#27704=CARTESIAN_POINT('Ctrl Pts',(0.175274276190844,1.,1.892646301985));
#27705=CARTESIAN_POINT('Ctrl Pts',(0.175538155840648,1.,1.88742606273259));
#27706=CARTESIAN_POINT('Ctrl Pts',(0.175644148889698,1.,1.88188663145367));
#27707=CARTESIAN_POINT('Ctrl Pts',(0.175563480746485,1.,1.87563767773588));
#27708=CARTESIAN_POINT('Ctrl Pts',(0.175268337590757,1.,1.86828349694799));
#27709=CARTESIAN_POINT('Ctrl Pts',(0.17473525927603,1.,1.85948367088837));
#27710=CARTESIAN_POINT('Ctrl Pts',(0.173946627587731,1.,1.8489811319852));
#27711=CARTESIAN_POINT('Ctrl Pts',(0.1728894428919,1.,1.83658380527692));
#27712=CARTESIAN_POINT('Ctrl Pts',(0.171554770204119,1.,1.82215766811545));
#27713=CARTESIAN_POINT('Ctrl Pts',(0.169936923904608,1.,1.80561530629706));
#27714=CARTESIAN_POINT('Ctrl Pts',(0.168032772805197,1.,1.7869064998507));
#27715=CARTESIAN_POINT('Ctrl Pts',(0.1662793551464,1.,1.77018771684844));
#27716=CARTESIAN_POINT('Ctrl Pts',(0.164834765707158,1.,1.75666056638427));
#27717=CARTESIAN_POINT('Ctrl Pts',(0.163814161002002,1.,1.7472034950333));
#27718=CARTESIAN_POINT('Ctrl Pts',(0.163289472382896,1.,1.74236521665491));
#27719=CARTESIAN_POINT('',(0.0694764450219578,0.,2.19890268624765));
#27720=CARTESIAN_POINT('Origin',(-0.0694764450219586,0.,2.19890268624765));
#27721=CARTESIAN_POINT('',(-0.0694764450219586,1.,2.19890268624765));
#27722=CARTESIAN_POINT('',(0.0694764450219578,1.,2.19890268624765));
#27723=CARTESIAN_POINT('',(-0.0694764450219586,0.,2.19890268624765));
#27724=CARTESIAN_POINT('Ctrl Pts',(-0.163289472382896,-1.,1.74236521665491));
#27725=CARTESIAN_POINT('Ctrl Pts',(-0.163289472382896,1.,1.74236521665491));
#27726=CARTESIAN_POINT('Ctrl Pts',(-0.163814161002474,-1.,1.74720349503904));
#27727=CARTESIAN_POINT('Ctrl Pts',(-0.163814161002474,1.,1.74720349503904));
#27728=CARTESIAN_POINT('Ctrl Pts',(-0.164834765708484,-1.,1.75666056640041));
#27729=CARTESIAN_POINT('Ctrl Pts',(-0.164834765708484,1.,1.75666056640041));
#27730=CARTESIAN_POINT('Ctrl Pts',(-0.166279355148738,-1.,1.77018771687692));
#27731=CARTESIAN_POINT('Ctrl Pts',(-0.166279355148738,1.,1.77018771687692));
#27732=CARTESIAN_POINT('Ctrl Pts',(-0.16803277280837,-1.,1.78690649988931));
#27733=CARTESIAN_POINT('Ctrl Pts',(-0.16803277280837,1.,1.78690649988931));
#27734=CARTESIAN_POINT('Ctrl Pts',(-0.169936923908078,-1.,1.80561530633924));
#27735=CARTESIAN_POINT('Ctrl Pts',(-0.169936923908078,1.,1.80561530633924));
#27736=CARTESIAN_POINT('Ctrl Pts',(-0.171554770207306,-1.,1.82215766815414));
#27737=CARTESIAN_POINT('Ctrl Pts',(-0.171554770207306,1.,1.82215766815414));
#27738=CARTESIAN_POINT('Ctrl Pts',(-0.17288944289442,-1.,1.83658380530747));
#27739=CARTESIAN_POINT('Ctrl Pts',(-0.17288944289442,1.,1.83658380530747));
#27740=CARTESIAN_POINT('Ctrl Pts',(-0.173946627589401,-1.,1.84898113200543));
#27741=CARTESIAN_POINT('Ctrl Pts',(-0.173946627589401,1.,1.84898113200543));
#27742=CARTESIAN_POINT('Ctrl Pts',(-0.174735259276856,-1.,1.85948367089838));
#27743=CARTESIAN_POINT('Ctrl Pts',(-0.174735259276856,1.,1.85948367089838));
#27744=CARTESIAN_POINT('Ctrl Pts',(-0.175268337590901,-1.,1.86828349694972));
#27745=CARTESIAN_POINT('Ctrl Pts',(-0.175268337590901,1.,1.86828349694972));
#27746=CARTESIAN_POINT('Ctrl Pts',(-0.175563480746206,-1.,1.87563767773249));
#27747=CARTESIAN_POINT('Ctrl Pts',(-0.175563480746206,1.,1.87563767773249));
#27748=CARTESIAN_POINT('Ctrl Pts',(-0.175644148889271,-1.,1.88188663144846));
#27749=CARTESIAN_POINT('Ctrl Pts',(-0.175644148889271,1.,1.88188663144846));
#27750=CARTESIAN_POINT('Ctrl Pts',(-0.175538155840286,-1.,1.88742606272818));
#27751=CARTESIAN_POINT('Ctrl Pts',(-0.175538155840286,1.,1.88742606272818));
#27752=CARTESIAN_POINT('Ctrl Pts',(-0.175274276190664,-1.,1.89264630198279));
#27753=CARTESIAN_POINT('Ctrl Pts',(-0.175274276190664,1.,1.89264630198279));
#27754=CARTESIAN_POINT('Ctrl Pts',(-0.174879405091277,-1.,1.89788101117148));
#27755=CARTESIAN_POINT('Ctrl Pts',(-0.174879405091277,1.,1.89788101117148));
#27756=CARTESIAN_POINT('Ctrl Pts',(-0.174375518661222,-1.,1.90335253863003));
#27757=CARTESIAN_POINT('Ctrl Pts',(-0.174375518661222,1.,1.90335253863003));
#27758=CARTESIAN_POINT('Ctrl Pts',(-0.173776635257984,-1.,1.90911693975475));
#27759=CARTESIAN_POINT('Ctrl Pts',(-0.173776635257984,1.,1.90911693975475));
#27760=CARTESIAN_POINT('Ctrl Pts',(-0.173090695383619,-1.,1.91511429159681));
#27761=CARTESIAN_POINT('Ctrl Pts',(-0.173090695383619,1.,1.91511429159681));
#27762=CARTESIAN_POINT('Ctrl Pts',(-0.172321621259557,-1.,1.92122334398034));
#27763=CARTESIAN_POINT('Ctrl Pts',(-0.172321621259557,1.,1.92122334398034));
#27764=CARTESIAN_POINT('Ctrl Pts',(-0.17147119153296,-1.,1.92731093582));
#27765=CARTESIAN_POINT('Ctrl Pts',(-0.17147119153296,1.,1.92731093582));
#27766=CARTESIAN_POINT('Ctrl Pts',(-0.170541253116136,-1.,1.93329183155455));
#27767=CARTESIAN_POINT('Ctrl Pts',(-0.170541253116136,1.,1.93329183155455));
#27768=CARTESIAN_POINT('Ctrl Pts',(-0.169534904817425,-1.,1.93915639211497));
#27769=CARTESIAN_POINT('Ctrl Pts',(-0.169534904817425,1.,1.93915639211497));
#27770=CARTESIAN_POINT('Ctrl Pts',(-0.168455741607516,-1.,1.94493757756879));
#27771=CARTESIAN_POINT('Ctrl Pts',(-0.168455741607516,1.,1.94493757756879));
#27772=CARTESIAN_POINT('Ctrl Pts',(-0.167307501784469,-1.,1.95069027794286));
#27773=CARTESIAN_POINT('Ctrl Pts',(-0.167307501784469,1.,1.95069027794286));
#27774=CARTESIAN_POINT('Ctrl Pts',(-0.166093592002833,-1.,1.95646759718755));
#27775=CARTESIAN_POINT('Ctrl Pts',(-0.166093592002833,1.,1.95646759718755));
#27776=CARTESIAN_POINT('Ctrl Pts',(-0.1648165689203,-1.,1.96229379940174));
#27777=CARTESIAN_POINT('Ctrl Pts',(-0.1648165689203,1.,1.96229379940174));
#27778=CARTESIAN_POINT('Ctrl Pts',(-0.16347818545776,-1.,1.96816512678));
#27779=CARTESIAN_POINT('Ctrl Pts',(-0.16347818545776,1.,1.96816512678));
#27780=CARTESIAN_POINT('Ctrl Pts',(-0.162079693556302,-1.,1.97406280235204));
#27781=CARTESIAN_POINT('Ctrl Pts',(-0.162079693556302,1.,1.97406280235204));
#27782=CARTESIAN_POINT('Ctrl Pts',(-0.16062206078461,-1.,1.97996195437557));
#27783=CARTESIAN_POINT('Ctrl Pts',(-0.16062206078461,1.,1.97996195437557));
#27784=CARTESIAN_POINT('Ctrl Pts',(-0.159106226437289,-1.,1.98584238283279));
#27785=CARTESIAN_POINT('Ctrl Pts',(-0.159106226437289,1.,1.98584238283279));
#27786=CARTESIAN_POINT('Ctrl Pts',(-0.157533331459215,-1.,1.99169810931893));
#27787=CARTESIAN_POINT('Ctrl Pts',(-0.157533331459215,1.,1.99169810931893));
#27788=CARTESIAN_POINT('Ctrl Pts',(-0.155904629548775,-1.,1.99753284771487));
#27789=CARTESIAN_POINT('Ctrl Pts',(-0.155904629548775,1.,1.99753284771487));
#27790=CARTESIAN_POINT('Ctrl Pts',(-0.154221403049719,-1.,2.00335565310539));
#27791=CARTESIAN_POINT('Ctrl Pts',(-0.154221403049719,1.,2.00335565310539));
#27792=CARTESIAN_POINT('Ctrl Pts',(-0.152484883621452,-1.,2.00917680318426));
#27793=CARTESIAN_POINT('Ctrl Pts',(-0.152484883621452,1.,2.00917680318426));
#27794=CARTESIAN_POINT('Ctrl Pts',(-0.150696157673084,-1.,2.01500291940243));
#27795=CARTESIAN_POINT('Ctrl Pts',(-0.150696157673084,1.,2.01500291940243));
#27796=CARTESIAN_POINT('Ctrl Pts',(-0.148856124775343,-1.,2.02083464969897));
#27797=CARTESIAN_POINT('Ctrl Pts',(-0.148856124775343,1.,2.02083464969897));
#27798=CARTESIAN_POINT('Ctrl Pts',(-0.146965557332586,-1.,2.02666926182017));
#27799=CARTESIAN_POINT('Ctrl Pts',(-0.146965557332586,1.,2.02666926182017));
#27800=CARTESIAN_POINT('Ctrl Pts',(-0.145025140186058,-1.,2.03250223739941));
#27801=CARTESIAN_POINT('Ctrl Pts',(-0.145025140186058,1.,2.03250223739941));
#27802=CARTESIAN_POINT('Ctrl Pts',(-0.143035515058208,-1.,2.03832911025913));
#27803=CARTESIAN_POINT('Ctrl Pts',(-0.143035515058208,1.,2.03832911025913));
#27804=CARTESIAN_POINT('Ctrl Pts',(-0.140997332152546,-1.,2.04414757947919));
#27805=CARTESIAN_POINT('Ctrl Pts',(-0.140997332152546,1.,2.04414757947919));
#27806=CARTESIAN_POINT('Ctrl Pts',(-0.138911255368966,-1.,2.04995762001333));
#27807=CARTESIAN_POINT('Ctrl Pts',(-0.138911255368966,1.,2.04995762001333));
#27808=CARTESIAN_POINT('Ctrl Pts',(-0.136777941218044,-1.,2.0557604441427));
#27809=CARTESIAN_POINT('Ctrl Pts',(-0.136777941218044,1.,2.0557604441427));
#27810=CARTESIAN_POINT('Ctrl Pts',(-0.134598026192107,-1.,2.06155781517844));
#27811=CARTESIAN_POINT('Ctrl Pts',(-0.134598026192107,1.,2.06155781517844));
#27812=CARTESIAN_POINT('Ctrl Pts',(-0.13237211154771,-1.,2.06735123910319));
#27813=CARTESIAN_POINT('Ctrl Pts',(-0.13237211154771,1.,2.06735123910319));
#27814=CARTESIAN_POINT('Ctrl Pts',(-0.130100748328401,-1.,2.07314114713047));
#27815=CARTESIAN_POINT('Ctrl Pts',(-0.130100748328401,1.,2.07314114713047));
#27816=CARTESIAN_POINT('Ctrl Pts',(-0.127784445276116,-1.,2.07892715110967));
#27817=CARTESIAN_POINT('Ctrl Pts',(-0.127784445276116,1.,2.07892715110967));
#27818=CARTESIAN_POINT('Ctrl Pts',(-0.125423679412058,-1.,2.08470840653628));
#27819=CARTESIAN_POINT('Ctrl Pts',(-0.125423679412058,1.,2.08470840653628));
#27820=CARTESIAN_POINT('Ctrl Pts',(-0.123018905621083,-1.,2.09048392424826));
#27821=CARTESIAN_POINT('Ctrl Pts',(-0.123018905621083,1.,2.09048392424826));
#27822=CARTESIAN_POINT('Ctrl Pts',(-0.120570567965129,-1.,2.09625292867756));
#27823=CARTESIAN_POINT('Ctrl Pts',(-0.120570567965129,1.,2.09625292867756));
#27824=CARTESIAN_POINT('Ctrl Pts',(-0.118079107988368,-1.,2.10201512132945));
#27825=CARTESIAN_POINT('Ctrl Pts',(-0.118079107988368,1.,2.10201512132945));
#27826=CARTESIAN_POINT('Ctrl Pts',(-0.115544957687941,-1.,2.10777050261359));
#27827=CARTESIAN_POINT('Ctrl Pts',(-0.115544957687941,1.,2.10777050261359));
#27828=CARTESIAN_POINT('Ctrl Pts',(-0.112968534419746,-1.,2.11351924490335));
#27829=CARTESIAN_POINT('Ctrl Pts',(-0.112968534419746,1.,2.11351924490335));
#27830=CARTESIAN_POINT('Ctrl Pts',(-0.11035023613502,-1.,2.11926155590849));
#27831=CARTESIAN_POINT('Ctrl Pts',(-0.11035023613502,1.,2.11926155590849));
#27832=CARTESIAN_POINT('Ctrl Pts',(-0.107690435231068,-1.,2.12499752306927));
#27833=CARTESIAN_POINT('Ctrl Pts',(-0.107690435231068,1.,2.12499752306927));
#27834=CARTESIAN_POINT('Ctrl Pts',(-0.104989479152703,-1.,2.1307270488718));
#27835=CARTESIAN_POINT('Ctrl Pts',(-0.104989479152703,1.,2.1307270488718));
#27836=CARTESIAN_POINT('Ctrl Pts',(-0.102247700556064,-1.,2.13644992667052));
#27837=CARTESIAN_POINT('Ctrl Pts',(-0.102247700556064,1.,2.13644992667052));
#27838=CARTESIAN_POINT('Ctrl Pts',(-0.0994654261990745,-1.,2.14216588395974));
#27839=CARTESIAN_POINT('Ctrl Pts',(-0.0994654261990745,1.,2.14216588395974));
#27840=CARTESIAN_POINT('Ctrl Pts',(-0.0966429852305691,-1.,2.14787463531864));
#27841=CARTESIAN_POINT('Ctrl Pts',(-0.0966429852305691,1.,2.14787463531864));
#27842=CARTESIAN_POINT('Ctrl Pts',(-0.0937807218868348,-1.,2.15357593978377));
#27843=CARTESIAN_POINT('Ctrl Pts',(-0.0937807218868348,1.,2.15357593978377));
#27844=CARTESIAN_POINT('Ctrl Pts',(-0.0908789888108269,-1.,2.15926961544808));
#27845=CARTESIAN_POINT('Ctrl Pts',(-0.0908789888108269,1.,2.15926961544808));
#27846=CARTESIAN_POINT('Ctrl Pts',(-0.0879381291387825,-1.,2.16495552645275));
#27847=CARTESIAN_POINT('Ctrl Pts',(-0.0879381291387825,1.,2.16495552645275));
#27848=CARTESIAN_POINT('Ctrl Pts',(-0.0849584620835646,-1.,2.17063357871031));
#27849=CARTESIAN_POINT('Ctrl Pts',(-0.0849584620835646,1.,2.17063357871031));
#27850=CARTESIAN_POINT('Ctrl Pts',(-0.0819402680871942,-1.,2.1763037121106));
#27851=CARTESIAN_POINT('Ctrl Pts',(-0.0819402680871942,1.,2.1763037121106));
#27852=CARTESIAN_POINT('Ctrl Pts',(-0.078883772768323,-1.,2.18196589448304));
#27853=CARTESIAN_POINT('Ctrl Pts',(-0.078883772768323,1.,2.18196589448304));
#27854=CARTESIAN_POINT('Ctrl Pts',(-0.0757891465833414,-1.,2.1876201139874));
#27855=CARTESIAN_POINT('Ctrl Pts',(-0.0757891465833414,1.,2.1876201139874));
#27856=CARTESIAN_POINT('Ctrl Pts',(-0.0732830357304279,-1.,2.19213712012956));
#27857=CARTESIAN_POINT('Ctrl Pts',(-0.0732830357304279,1.,2.19213712012956));
#27858=CARTESIAN_POINT('Ctrl Pts',(-0.071386377952463,-1.,2.19552129483562));
#27859=CARTESIAN_POINT('Ctrl Pts',(-0.071386377952463,1.,2.19552129483562));
#27860=CARTESIAN_POINT('Ctrl Pts',(-0.0701143536324929,-1.,2.19777582085261));
#27861=CARTESIAN_POINT('Ctrl Pts',(-0.0701143536324929,1.,2.19777582085261));
#27862=CARTESIAN_POINT('Ctrl Pts',(-0.0694764450219586,-1.,2.19890268624765));
#27863=CARTESIAN_POINT('Ctrl Pts',(-0.0694764450219586,1.,2.19890268624765));
#27864=CARTESIAN_POINT('',(-0.163289472382896,1.,1.74236521665491));
#27865=CARTESIAN_POINT('Ctrl Pts',(-0.163289472382896,1.,1.74236521665491));
#27866=CARTESIAN_POINT('Ctrl Pts',(-0.163814161002474,1.,1.74720349503904));
#27867=CARTESIAN_POINT('Ctrl Pts',(-0.164834765708484,1.,1.75666056640041));
#27868=CARTESIAN_POINT('Ctrl Pts',(-0.166279355148738,1.,1.77018771687692));
#27869=CARTESIAN_POINT('Ctrl Pts',(-0.16803277280837,1.,1.78690649988931));
#27870=CARTESIAN_POINT('Ctrl Pts',(-0.169936923908078,1.,1.80561530633924));
#27871=CARTESIAN_POINT('Ctrl Pts',(-0.171554770207306,1.,1.82215766815414));
#27872=CARTESIAN_POINT('Ctrl Pts',(-0.17288944289442,1.,1.83658380530747));
#27873=CARTESIAN_POINT('Ctrl Pts',(-0.173946627589401,1.,1.84898113200543));
#27874=CARTESIAN_POINT('Ctrl Pts',(-0.174735259276856,1.,1.85948367089838));
#27875=CARTESIAN_POINT('Ctrl Pts',(-0.175268337590901,1.,1.86828349694972));
#27876=CARTESIAN_POINT('Ctrl Pts',(-0.175563480746206,1.,1.87563767773249));
#27877=CARTESIAN_POINT('Ctrl Pts',(-0.175644148889271,1.,1.88188663144846));
#27878=CARTESIAN_POINT('Ctrl Pts',(-0.175538155840286,1.,1.88742606272818));
#27879=CARTESIAN_POINT('Ctrl Pts',(-0.175274276190664,1.,1.89264630198279));
#27880=CARTESIAN_POINT('Ctrl Pts',(-0.174879405091277,1.,1.89788101117148));
#27881=CARTESIAN_POINT('Ctrl Pts',(-0.174375518661222,1.,1.90335253863003));
#27882=CARTESIAN_POINT('Ctrl Pts',(-0.173776635257984,1.,1.90911693975475));
#27883=CARTESIAN_POINT('Ctrl Pts',(-0.173090695383619,1.,1.91511429159681));
#27884=CARTESIAN_POINT('Ctrl Pts',(-0.172321621259557,1.,1.92122334398034));
#27885=CARTESIAN_POINT('Ctrl Pts',(-0.17147119153296,1.,1.92731093582));
#27886=CARTESIAN_POINT('Ctrl Pts',(-0.170541253116136,1.,1.93329183155455));
#27887=CARTESIAN_POINT('Ctrl Pts',(-0.169534904817425,1.,1.93915639211497));
#27888=CARTESIAN_POINT('Ctrl Pts',(-0.168455741607516,1.,1.94493757756879));
#27889=CARTESIAN_POINT('Ctrl Pts',(-0.167307501784469,1.,1.95069027794286));
#27890=CARTESIAN_POINT('Ctrl Pts',(-0.166093592002833,1.,1.95646759718755));
#27891=CARTESIAN_POINT('Ctrl Pts',(-0.1648165689203,1.,1.96229379940174));
#27892=CARTESIAN_POINT('Ctrl Pts',(-0.16347818545776,1.,1.96816512678));
#27893=CARTESIAN_POINT('Ctrl Pts',(-0.162079693556302,1.,1.97406280235204));
#27894=CARTESIAN_POINT('Ctrl Pts',(-0.16062206078461,1.,1.97996195437557));
#27895=CARTESIAN_POINT('Ctrl Pts',(-0.159106226437289,1.,1.98584238283279));
#27896=CARTESIAN_POINT('Ctrl Pts',(-0.157533331459215,1.,1.99169810931893));
#27897=CARTESIAN_POINT('Ctrl Pts',(-0.155904629548775,1.,1.99753284771487));
#27898=CARTESIAN_POINT('Ctrl Pts',(-0.154221403049719,1.,2.00335565310539));
#27899=CARTESIAN_POINT('Ctrl Pts',(-0.152484883621452,1.,2.00917680318426));
#27900=CARTESIAN_POINT('Ctrl Pts',(-0.150696157673084,1.,2.01500291940243));
#27901=CARTESIAN_POINT('Ctrl Pts',(-0.148856124775343,1.,2.02083464969897));
#27902=CARTESIAN_POINT('Ctrl Pts',(-0.146965557332586,1.,2.02666926182017));
#27903=CARTESIAN_POINT('Ctrl Pts',(-0.145025140186058,1.,2.03250223739941));
#27904=CARTESIAN_POINT('Ctrl Pts',(-0.143035515058208,1.,2.03832911025913));
#27905=CARTESIAN_POINT('Ctrl Pts',(-0.140997332152546,1.,2.04414757947919));
#27906=CARTESIAN_POINT('Ctrl Pts',(-0.138911255368966,1.,2.04995762001333));
#27907=CARTESIAN_POINT('Ctrl Pts',(-0.136777941218044,1.,2.0557604441427));
#27908=CARTESIAN_POINT('Ctrl Pts',(-0.134598026192107,1.,2.06155781517844));
#27909=CARTESIAN_POINT('Ctrl Pts',(-0.13237211154771,1.,2.06735123910319));
#27910=CARTESIAN_POINT('Ctrl Pts',(-0.130100748328401,1.,2.07314114713047));
#27911=CARTESIAN_POINT('Ctrl Pts',(-0.127784445276116,1.,2.07892715110967));
#27912=CARTESIAN_POINT('Ctrl Pts',(-0.125423679412058,1.,2.08470840653628));
#27913=CARTESIAN_POINT('Ctrl Pts',(-0.123018905621083,1.,2.09048392424826));
#27914=CARTESIAN_POINT('Ctrl Pts',(-0.120570567965129,1.,2.09625292867756));
#27915=CARTESIAN_POINT('Ctrl Pts',(-0.118079107988368,1.,2.10201512132945));
#27916=CARTESIAN_POINT('Ctrl Pts',(-0.115544957687941,1.,2.10777050261359));
#27917=CARTESIAN_POINT('Ctrl Pts',(-0.112968534419746,1.,2.11351924490335));
#27918=CARTESIAN_POINT('Ctrl Pts',(-0.11035023613502,1.,2.11926155590849));
#27919=CARTESIAN_POINT('Ctrl Pts',(-0.107690435231068,1.,2.12499752306927));
#27920=CARTESIAN_POINT('Ctrl Pts',(-0.104989479152703,1.,2.1307270488718));
#27921=CARTESIAN_POINT('Ctrl Pts',(-0.102247700556064,1.,2.13644992667052));
#27922=CARTESIAN_POINT('Ctrl Pts',(-0.0994654261990745,1.,2.14216588395974));
#27923=CARTESIAN_POINT('Ctrl Pts',(-0.0966429852305691,1.,2.14787463531864));
#27924=CARTESIAN_POINT('Ctrl Pts',(-0.0937807218868348,1.,2.15357593978377));
#27925=CARTESIAN_POINT('Ctrl Pts',(-0.0908789888108269,1.,2.15926961544808));
#27926=CARTESIAN_POINT('Ctrl Pts',(-0.0879381291387825,1.,2.16495552645275));
#27927=CARTESIAN_POINT('Ctrl Pts',(-0.0849584620835646,1.,2.17063357871031));
#27928=CARTESIAN_POINT('Ctrl Pts',(-0.0819402680871942,1.,2.1763037121106));
#27929=CARTESIAN_POINT('Ctrl Pts',(-0.078883772768323,1.,2.18196589448304));
#27930=CARTESIAN_POINT('Ctrl Pts',(-0.0757891465833414,1.,2.1876201139874));
#27931=CARTESIAN_POINT('Ctrl Pts',(-0.0732830357304279,1.,2.19213712012956));
#27932=CARTESIAN_POINT('Ctrl Pts',(-0.071386377952463,1.,2.19552129483562));
#27933=CARTESIAN_POINT('Ctrl Pts',(-0.0701143536324929,1.,2.19777582085261));
#27934=CARTESIAN_POINT('Ctrl Pts',(-0.0694764450219586,1.,2.19890268624765));
#27935=CARTESIAN_POINT('',(-0.163289472382897,0.,1.74236521665491));
#27936=CARTESIAN_POINT('Origin',(0.,0.,0.));
#27937=CARTESIAN_POINT('',(-0.383122945602004,1.,1.7075470150345));
#27938=CARTESIAN_POINT('Origin',(0.,1.,0.));
#27939=CARTESIAN_POINT('',(-0.383122945602004,0.,1.7075470150345));
#27940=CARTESIAN_POINT('Ctrl Pts',(-0.61342227326009,-1.,2.11275013067528));
#27941=CARTESIAN_POINT('Ctrl Pts',(-0.61342227326009,1.,2.11275013067528));
#27942=CARTESIAN_POINT('Ctrl Pts',(-0.61246736556225,-1.,2.11187554260142));
#27943=CARTESIAN_POINT('Ctrl Pts',(-0.61246736556225,1.,2.11187554260142));
#27944=CARTESIAN_POINT('Ctrl Pts',(-0.610560911691113,-1.,2.11012443807661));
#27945=CARTESIAN_POINT('Ctrl Pts',(-0.610560911691113,1.,2.11012443807661));
#27946=CARTESIAN_POINT('Ctrl Pts',(-0.607711315456826,-1.,2.10749199615859));
#27947=CARTESIAN_POINT('Ctrl Pts',(-0.607711315456826,1.,2.10749199615859));
#27948=CARTESIAN_POINT('Ctrl Pts',(-0.603932030738212,-1.,2.10397049887709));
#27949=CARTESIAN_POINT('Ctrl Pts',(-0.603932030738212,1.,2.10397049887709));
#27950=CARTESIAN_POINT('Ctrl Pts',(-0.599241616422144,-1.,2.09954930865331));
#27951=CARTESIAN_POINT('Ctrl Pts',(-0.599241616422144,1.,2.09954930865331));
#27952=CARTESIAN_POINT('Ctrl Pts',(-0.594585006052824,-1.,2.09510876220501));
#27953=CARTESIAN_POINT('Ctrl Pts',(-0.594585006052824,1.,2.09510876220501));
#27954=CARTESIAN_POINT('Ctrl Pts',(-0.589962365403189,-1.,2.09064881812053));
#27955=CARTESIAN_POINT('Ctrl Pts',(-0.589962365403189,1.,2.09064881812053));
#27956=CARTESIAN_POINT('Ctrl Pts',(-0.585373918990895,-1.,2.086169437277));
#27957=CARTESIAN_POINT('Ctrl Pts',(-0.585373918990895,1.,2.086169437277));
#27958=CARTESIAN_POINT('Ctrl Pts',(-0.580819952107257,-1.,2.08167059018138));
#27959=CARTESIAN_POINT('Ctrl Pts',(-0.580819952107257,1.,2.08167059018138));
#27960=CARTESIAN_POINT('Ctrl Pts',(-0.576300797416275,-1.,2.07715226767361));
#27961=CARTESIAN_POINT('Ctrl Pts',(-0.576300797416275,1.,2.07715226767361));
#27962=CARTESIAN_POINT('Ctrl Pts',(-0.571816823242411,-1.,2.07261449292757));
#27963=CARTESIAN_POINT('Ctrl Pts',(-0.571816823242411,1.,2.07261449292757));
#27964=CARTESIAN_POINT('Ctrl Pts',(-0.567368421181229,-1.,2.06805732997383));
#27965=CARTESIAN_POINT('Ctrl Pts',(-0.567368421181229,1.,2.06805732997383));
#27966=CARTESIAN_POINT('Ctrl Pts',(-0.562955993082574,-1.,2.06348090160697));
#27967=CARTESIAN_POINT('Ctrl Pts',(-0.562955993082574,1.,2.06348090160697));
#27968=CARTESIAN_POINT('Ctrl Pts',(-0.558579940185467,-1.,2.05888537756571));
#27969=CARTESIAN_POINT('Ctrl Pts',(-0.558579940185467,1.,2.05888537756571));
#27970=CARTESIAN_POINT('Ctrl Pts',(-0.55424065746411,-1.,2.05427091604482));
#27971=CARTESIAN_POINT('Ctrl Pts',(-0.55424065746411,1.,2.05427091604482));
#27972=CARTESIAN_POINT('Ctrl Pts',(-0.549938525150342,-1.,2.04963761077974));
#27973=CARTESIAN_POINT('Ctrl Pts',(-0.549938525150342,1.,2.04963761077974));
#27974=CARTESIAN_POINT('Ctrl Pts',(-0.545673903817348,-1.,2.0449854471456));
#27975=CARTESIAN_POINT('Ctrl Pts',(-0.545673903817348,1.,2.0449854471456));
#27976=CARTESIAN_POINT('Ctrl Pts',(-0.54144712061552,-1.,2.0403142269048));
#27977=CARTESIAN_POINT('Ctrl Pts',(-0.54144712061552,1.,2.0403142269048));
#27978=CARTESIAN_POINT('Ctrl Pts',(-0.537258489833134,-1.,2.03562362953993));
#27979=CARTESIAN_POINT('Ctrl Pts',(-0.537258489833134,1.,2.03562362953993));
#27980=CARTESIAN_POINT('Ctrl Pts',(-0.533108355132905,-1.,2.03091336214401));
#27981=CARTESIAN_POINT('Ctrl Pts',(-0.533108355132905,1.,2.03091336214401));
#27982=CARTESIAN_POINT('Ctrl Pts',(-0.528997127241911,-1.,2.02618329083289));
#27983=CARTESIAN_POINT('Ctrl Pts',(-0.528997127241911,1.,2.02618329083289));
#27984=CARTESIAN_POINT('Ctrl Pts',(-0.524925318333518,-1.,2.02143356304712));
#27985=CARTESIAN_POINT('Ctrl Pts',(-0.524925318333518,1.,2.02143356304712));
#27986=CARTESIAN_POINT('Ctrl Pts',(-0.520893590399428,-1.,2.01666477917305));
#27987=CARTESIAN_POINT('Ctrl Pts',(-0.520893590399428,1.,2.01666477917305));
#27988=CARTESIAN_POINT('Ctrl Pts',(-0.516902681728733,-1.,2.01187773939257));
#27989=CARTESIAN_POINT('Ctrl Pts',(-0.516902681728733,1.,2.01187773939257));
#27990=CARTESIAN_POINT('Ctrl Pts',(-0.512953306961814,-1.,2.00707309946955));
#27991=CARTESIAN_POINT('Ctrl Pts',(-0.512953306961814,1.,2.00707309946955));
#27992=CARTESIAN_POINT('Ctrl Pts',(-0.509046069886152,-1.,2.00225107134733));
#27993=CARTESIAN_POINT('Ctrl Pts',(-0.509046069886152,1.,2.00225107134733));
#27994=CARTESIAN_POINT('Ctrl Pts',(-0.505181361323011,-1.,1.99741107463567));
#27995=CARTESIAN_POINT('Ctrl Pts',(-0.505181361323011,1.,1.99741107463567));
#27996=CARTESIAN_POINT('Ctrl Pts',(-0.501359287727129,-1.,1.9925514912615));
#27997=CARTESIAN_POINT('Ctrl Pts',(-0.501359287727129,1.,1.9925514912615));
#27998=CARTESIAN_POINT('Ctrl Pts',(-0.497579909545564,-1.,1.98767044752929));
#27999=CARTESIAN_POINT('Ctrl Pts',(-0.497579909545564,1.,1.98767044752929));
#28000=CARTESIAN_POINT('Ctrl Pts',(-0.493843476541492,-1.,1.9827665876182));
#28001=CARTESIAN_POINT('Ctrl Pts',(-0.493843476541492,1.,1.9827665876182));
#28002=CARTESIAN_POINT('Ctrl Pts',(-0.490150627860955,-1.,1.97783973019229));
#28003=CARTESIAN_POINT('Ctrl Pts',(-0.490150627860955,1.,1.97783973019229));
#28004=CARTESIAN_POINT('Ctrl Pts',(-0.486502692907661,-1.,1.97289186263272));
#28005=CARTESIAN_POINT('Ctrl Pts',(-0.486502692907661,1.,1.97289186263272));
#28006=CARTESIAN_POINT('Ctrl Pts',(-0.482901662120687,-1.,1.96792703422358));
#28007=CARTESIAN_POINT('Ctrl Pts',(-0.482901662120687,1.,1.96792703422358));
#28008=CARTESIAN_POINT('Ctrl Pts',(-0.479349583074846,-1.,1.96294933055938));
#28009=CARTESIAN_POINT('Ctrl Pts',(-0.479349583074846,1.,1.96294933055938));
#28010=CARTESIAN_POINT('Ctrl Pts',(-0.475848034683172,-1.,1.95796111148175));
#28011=CARTESIAN_POINT('Ctrl Pts',(-0.475848034683172,1.,1.95796111148175));
#28012=CARTESIAN_POINT('Ctrl Pts',(-0.47239767226408,-1.,1.95296148278136));
#28013=CARTESIAN_POINT('Ctrl Pts',(-0.47239767226408,1.,1.95296148278136));
#28014=CARTESIAN_POINT('Ctrl Pts',(-0.468997482913158,-1.,1.94794381136524));
#28015=CARTESIAN_POINT('Ctrl Pts',(-0.468997482913158,1.,1.94794381136524));
#28016=CARTESIAN_POINT('Ctrl Pts',(-0.465645462026065,-1.,1.94289794196205));
#28017=CARTESIAN_POINT('Ctrl Pts',(-0.465645462026065,1.,1.94289794196205));
#28018=CARTESIAN_POINT('Ctrl Pts',(-0.462340031009087,-1.,1.93781486640834));
#28019=CARTESIAN_POINT('Ctrl Pts',(-0.462340031009087,1.,1.93781486640834));
#28020=CARTESIAN_POINT('Ctrl Pts',(-0.459081234547931,-1.,1.93269066517936));
#28021=CARTESIAN_POINT('Ctrl Pts',(-0.459081234547931,1.,1.93269066517936));
#28022=CARTESIAN_POINT('Ctrl Pts',(-0.455872005174335,-1.,1.92753067150461));
#28023=CARTESIAN_POINT('Ctrl Pts',(-0.455872005174335,1.,1.92753067150461));
#28024=CARTESIAN_POINT('Ctrl Pts',(-0.452719478359356,-1.,1.9223538064847));
#28025=CARTESIAN_POINT('Ctrl Pts',(-0.452719478359356,1.,1.9223538064847));
#28026=CARTESIAN_POINT('Ctrl Pts',(-0.449632260106572,-1.,1.91718342555717));
#28027=CARTESIAN_POINT('Ctrl Pts',(-0.449632260106572,1.,1.91718342555717));
#28028=CARTESIAN_POINT('Ctrl Pts',(-0.446617343485651,-1.,1.91203699981095));
#28029=CARTESIAN_POINT('Ctrl Pts',(-0.446617343485651,1.,1.91203699981095));
#28030=CARTESIAN_POINT('Ctrl Pts',(-0.44367755684917,-1.,1.90691756144906));
#28031=CARTESIAN_POINT('Ctrl Pts',(-0.44367755684917,1.,1.90691756144906));
#28032=CARTESIAN_POINT('Ctrl Pts',(-0.440807833704161,-1.,1.90180124389137));
#28033=CARTESIAN_POINT('Ctrl Pts',(-0.440807833704161,1.,1.90180124389137));
#28034=CARTESIAN_POINT('Ctrl Pts',(-0.437995003948443,-1.,1.89663648956549));
#28035=CARTESIAN_POINT('Ctrl Pts',(-0.437995003948443,1.,1.89663648956549));
#28036=CARTESIAN_POINT('Ctrl Pts',(-0.43522566096358,-1.,1.89136993975585));
#28037=CARTESIAN_POINT('Ctrl Pts',(-0.43522566096358,1.,1.89136993975585));
#28038=CARTESIAN_POINT('Ctrl Pts',(-0.432493038548833,-1.,1.88596913666828));
#28039=CARTESIAN_POINT('Ctrl Pts',(-0.432493038548833,1.,1.88596913666828));
#28040=CARTESIAN_POINT('Ctrl Pts',(-0.429803062482217,-1.,1.88044229001778));
#28041=CARTESIAN_POINT('Ctrl Pts',(-0.429803062482217,1.,1.88044229001778));
#28042=CARTESIAN_POINT('Ctrl Pts',(-0.427183828518743,-1.,1.87486989291333));
#28043=CARTESIAN_POINT('Ctrl Pts',(-0.427183828518743,1.,1.87486989291333));
#28044=CARTESIAN_POINT('Ctrl Pts',(-0.424678177290876,-1.,1.8693780394412));
#28045=CARTESIAN_POINT('Ctrl Pts',(-0.424678177290876,1.,1.8693780394412));
#28046=CARTESIAN_POINT('Ctrl Pts',(-0.422327307417885,-1.,1.86408083333863));
#28047=CARTESIAN_POINT('Ctrl Pts',(-0.422327307417885,1.,1.86408083333863));
#28048=CARTESIAN_POINT('Ctrl Pts',(-0.420157287975583,-1.,1.8590328109667));
#28049=CARTESIAN_POINT('Ctrl Pts',(-0.420157287975583,1.,1.8590328109667));
#28050=CARTESIAN_POINT('Ctrl Pts',(-0.418164129144045,-1.,1.8541763285645));
#28051=CARTESIAN_POINT('Ctrl Pts',(-0.418164129144045,1.,1.8541763285645));
#28052=CARTESIAN_POINT('Ctrl Pts',(-0.416300022039885,-1.,1.84929312930314));
#28053=CARTESIAN_POINT('Ctrl Pts',(-0.416300022039885,1.,1.84929312930314));
#28054=CARTESIAN_POINT('Ctrl Pts',(-0.414487438255542,-1.,1.84405757074218));
#28055=CARTESIAN_POINT('Ctrl Pts',(-0.414487438255542,1.,1.84405757074218));
#28056=CARTESIAN_POINT('Ctrl Pts',(-0.412633125322945,-1.,1.8380895347617));
#28057=CARTESIAN_POINT('Ctrl Pts',(-0.412633125322945,1.,1.8380895347617));
#28058=CARTESIAN_POINT('Ctrl Pts',(-0.410641256301276,-1.,1.83100408895047));
#28059=CARTESIAN_POINT('Ctrl Pts',(-0.410641256301276,1.,1.83100408895047));
#28060=CARTESIAN_POINT('Ctrl Pts',(-0.408428948106227,-1.,1.82247022677562));
#28061=CARTESIAN_POINT('Ctrl Pts',(-0.408428948106227,1.,1.82247022677562));
#28062=CARTESIAN_POINT('Ctrl Pts',(-0.405933518407175,-1.,1.81223801812013));
#28063=CARTESIAN_POINT('Ctrl Pts',(-0.405933518407175,1.,1.81223801812013));
#28064=CARTESIAN_POINT('Ctrl Pts',(-0.403107976163396,-1.,1.80012077173238));
#28065=CARTESIAN_POINT('Ctrl Pts',(-0.403107976163396,1.,1.80012077173238));
#28066=CARTESIAN_POINT('Ctrl Pts',(-0.399919403774155,-1.,1.78598826343754));
#28067=CARTESIAN_POINT('Ctrl Pts',(-0.399919403774155,1.,1.78598826343754));
#28068=CARTESIAN_POINT('Ctrl Pts',(-0.396346196110688,-1.,1.76975560043442));
#28069=CARTESIAN_POINT('Ctrl Pts',(-0.396346196110688,1.,1.76975560043442));
#28070=CARTESIAN_POINT('Ctrl Pts',(-0.392375812285395,-1.,1.75137405310193));
#28071=CARTESIAN_POINT('Ctrl Pts',(-0.392375812285395,1.,1.75137405310193));
#28072=CARTESIAN_POINT('Ctrl Pts',(-0.388877023502615,-1.,1.73493170972829));
#28073=CARTESIAN_POINT('Ctrl Pts',(-0.388877023502615,1.,1.73493170972829));
#28074=CARTESIAN_POINT('Ctrl Pts',(-0.386070790323281,-1.,1.72162022244582));
#28075=CARTESIAN_POINT('Ctrl Pts',(-0.386070790323281,1.,1.72162022244582));
#28076=CARTESIAN_POINT('Ctrl Pts',(-0.384119047314215,-1.,1.71231062891398));
#28077=CARTESIAN_POINT('Ctrl Pts',(-0.384119047314215,1.,1.71231062891398));
#28078=CARTESIAN_POINT('Ctrl Pts',(-0.383122945602004,-1.,1.7075470150345));
#28079=CARTESIAN_POINT('Ctrl Pts',(-0.383122945602004,1.,1.7075470150345));
#28080=CARTESIAN_POINT('',(-0.61342227326009,1.,2.11275013067528));
#28081=CARTESIAN_POINT('Ctrl Pts',(-0.61342227326009,1.,2.11275013067528));
#28082=CARTESIAN_POINT('Ctrl Pts',(-0.61246736556225,1.,2.11187554260142));
#28083=CARTESIAN_POINT('Ctrl Pts',(-0.610560911691113,1.,2.11012443807661));
#28084=CARTESIAN_POINT('Ctrl Pts',(-0.607711315456826,1.,2.10749199615859));
#28085=CARTESIAN_POINT('Ctrl Pts',(-0.603932030738212,1.,2.10397049887709));
#28086=CARTESIAN_POINT('Ctrl Pts',(-0.599241616422144,1.,2.09954930865331));
#28087=CARTESIAN_POINT('Ctrl Pts',(-0.594585006052824,1.,2.09510876220501));
#28088=CARTESIAN_POINT('Ctrl Pts',(-0.589962365403189,1.,2.09064881812053));
#28089=CARTESIAN_POINT('Ctrl Pts',(-0.585373918990895,1.,2.086169437277));
#28090=CARTESIAN_POINT('Ctrl Pts',(-0.580819952107257,1.,2.08167059018138));
#28091=CARTESIAN_POINT('Ctrl Pts',(-0.576300797416275,1.,2.07715226767361));
#28092=CARTESIAN_POINT('Ctrl Pts',(-0.571816823242411,1.,2.07261449292757));
#28093=CARTESIAN_POINT('Ctrl Pts',(-0.567368421181229,1.,2.06805732997383));
#28094=CARTESIAN_POINT('Ctrl Pts',(-0.562955993082574,1.,2.06348090160697));
#28095=CARTESIAN_POINT('Ctrl Pts',(-0.558579940185467,1.,2.05888537756571));
#28096=CARTESIAN_POINT('Ctrl Pts',(-0.55424065746411,1.,2.05427091604482));
#28097=CARTESIAN_POINT('Ctrl Pts',(-0.549938525150342,1.,2.04963761077974));
#28098=CARTESIAN_POINT('Ctrl Pts',(-0.545673903817348,1.,2.0449854471456));
#28099=CARTESIAN_POINT('Ctrl Pts',(-0.54144712061552,1.,2.0403142269048));
#28100=CARTESIAN_POINT('Ctrl Pts',(-0.537258489833134,1.,2.03562362953993));
#28101=CARTESIAN_POINT('Ctrl Pts',(-0.533108355132905,1.,2.03091336214401));
#28102=CARTESIAN_POINT('Ctrl Pts',(-0.528997127241911,1.,2.02618329083289));
#28103=CARTESIAN_POINT('Ctrl Pts',(-0.524925318333518,1.,2.02143356304712));
#28104=CARTESIAN_POINT('Ctrl Pts',(-0.520893590399428,1.,2.01666477917305));
#28105=CARTESIAN_POINT('Ctrl Pts',(-0.516902681728733,1.,2.01187773939257));
#28106=CARTESIAN_POINT('Ctrl Pts',(-0.512953306961814,1.,2.00707309946955));
#28107=CARTESIAN_POINT('Ctrl Pts',(-0.509046069886152,1.,2.00225107134733));
#28108=CARTESIAN_POINT('Ctrl Pts',(-0.505181361323011,1.,1.99741107463567));
#28109=CARTESIAN_POINT('Ctrl Pts',(-0.501359287727129,1.,1.9925514912615));
#28110=CARTESIAN_POINT('Ctrl Pts',(-0.497579909545564,1.,1.98767044752929));
#28111=CARTESIAN_POINT('Ctrl Pts',(-0.493843476541492,1.,1.9827665876182));
#28112=CARTESIAN_POINT('Ctrl Pts',(-0.490150627860955,1.,1.97783973019229));
#28113=CARTESIAN_POINT('Ctrl Pts',(-0.486502692907661,1.,1.97289186263272));
#28114=CARTESIAN_POINT('Ctrl Pts',(-0.482901662120687,1.,1.96792703422358));
#28115=CARTESIAN_POINT('Ctrl Pts',(-0.479349583074846,1.,1.96294933055938));
#28116=CARTESIAN_POINT('Ctrl Pts',(-0.475848034683172,1.,1.95796111148175));
#28117=CARTESIAN_POINT('Ctrl Pts',(-0.47239767226408,1.,1.95296148278136));
#28118=CARTESIAN_POINT('Ctrl Pts',(-0.468997482913158,1.,1.94794381136524));
#28119=CARTESIAN_POINT('Ctrl Pts',(-0.465645462026065,1.,1.94289794196205));
#28120=CARTESIAN_POINT('Ctrl Pts',(-0.462340031009087,1.,1.93781486640834));
#28121=CARTESIAN_POINT('Ctrl Pts',(-0.459081234547931,1.,1.93269066517936));
#28122=CARTESIAN_POINT('Ctrl Pts',(-0.455872005174335,1.,1.92753067150461));
#28123=CARTESIAN_POINT('Ctrl Pts',(-0.452719478359356,1.,1.9223538064847));
#28124=CARTESIAN_POINT('Ctrl Pts',(-0.449632260106572,1.,1.91718342555717));
#28125=CARTESIAN_POINT('Ctrl Pts',(-0.446617343485651,1.,1.91203699981095));
#28126=CARTESIAN_POINT('Ctrl Pts',(-0.44367755684917,1.,1.90691756144906));
#28127=CARTESIAN_POINT('Ctrl Pts',(-0.440807833704161,1.,1.90180124389137));
#28128=CARTESIAN_POINT('Ctrl Pts',(-0.437995003948443,1.,1.89663648956549));
#28129=CARTESIAN_POINT('Ctrl Pts',(-0.43522566096358,1.,1.89136993975585));
#28130=CARTESIAN_POINT('Ctrl Pts',(-0.432493038548833,1.,1.88596913666828));
#28131=CARTESIAN_POINT('Ctrl Pts',(-0.429803062482217,1.,1.88044229001778));
#28132=CARTESIAN_POINT('Ctrl Pts',(-0.427183828518743,1.,1.87486989291333));
#28133=CARTESIAN_POINT('Ctrl Pts',(-0.424678177290876,1.,1.8693780394412));
#28134=CARTESIAN_POINT('Ctrl Pts',(-0.422327307417885,1.,1.86408083333863));
#28135=CARTESIAN_POINT('Ctrl Pts',(-0.420157287975583,1.,1.8590328109667));
#28136=CARTESIAN_POINT('Ctrl Pts',(-0.418164129144045,1.,1.8541763285645));
#28137=CARTESIAN_POINT('Ctrl Pts',(-0.416300022039885,1.,1.84929312930314));
#28138=CARTESIAN_POINT('Ctrl Pts',(-0.414487438255542,1.,1.84405757074218));
#28139=CARTESIAN_POINT('Ctrl Pts',(-0.412633125322945,1.,1.8380895347617));
#28140=CARTESIAN_POINT('Ctrl Pts',(-0.410641256301276,1.,1.83100408895047));
#28141=CARTESIAN_POINT('Ctrl Pts',(-0.408428948106227,1.,1.82247022677562));
#28142=CARTESIAN_POINT('Ctrl Pts',(-0.405933518407175,1.,1.81223801812013));
#28143=CARTESIAN_POINT('Ctrl Pts',(-0.403107976163396,1.,1.80012077173238));
#28144=CARTESIAN_POINT('Ctrl Pts',(-0.399919403774155,1.,1.78598826343754));
#28145=CARTESIAN_POINT('Ctrl Pts',(-0.396346196110688,1.,1.76975560043442));
#28146=CARTESIAN_POINT('Ctrl Pts',(-0.392375812285395,1.,1.75137405310193));
#28147=CARTESIAN_POINT('Ctrl Pts',(-0.388877023502615,1.,1.73493170972829));
#28148=CARTESIAN_POINT('Ctrl Pts',(-0.386070790323281,1.,1.72162022244582));
#28149=CARTESIAN_POINT('Ctrl Pts',(-0.384119047314215,1.,1.71231062891398));
#28150=CARTESIAN_POINT('Ctrl Pts',(-0.383122945602004,1.,1.7075470150345));
#28151=CARTESIAN_POINT('',(-0.61342227326009,0.,2.11275013067528));
#28152=CARTESIAN_POINT('Origin',(-0.745574324794401,0.,2.0698113262342));
#28153=CARTESIAN_POINT('',(-0.745574324794401,1.,2.0698113262342));
#28154=CARTESIAN_POINT('',(-0.61342227326009,1.,2.11275013067528));
#28155=CARTESIAN_POINT('',(-0.745574324794401,0.,2.0698113262342));
#28156=CARTESIAN_POINT('Ctrl Pts',(-0.693717979106306,-1.,1.60662857109684));
#28157=CARTESIAN_POINT('Ctrl Pts',(-0.693717979106306,1.,1.60662857109684));
#28158=CARTESIAN_POINT('Ctrl Pts',(-0.695712097881194,-1.,1.61106790958151));
#28159=CARTESIAN_POINT('Ctrl Pts',(-0.695712097881194,1.,1.61106790958151));
#28160=CARTESIAN_POINT('Ctrl Pts',(-0.699605146405088,-1.,1.61974673472612));
#28161=CARTESIAN_POINT('Ctrl Pts',(-0.699605146405088,1.,1.61974673472612));
#28162=CARTESIAN_POINT('Ctrl Pts',(-0.705159151988319,-1.,1.63216541664676));
#28163=CARTESIAN_POINT('Ctrl Pts',(-0.705159151988319,1.,1.63216541664676));
#28164=CARTESIAN_POINT('Ctrl Pts',(-0.711993139355394,-1.,1.64752408832016));
#28165=CARTESIAN_POINT('Ctrl Pts',(-0.711993139355394,1.,1.64752408832016));
#28166=CARTESIAN_POINT('Ctrl Pts',(-0.719585433804282,-1.,1.6647288055568));
#28167=CARTESIAN_POINT('Ctrl Pts',(-0.719585433804282,1.,1.6647288055568));
#28168=CARTESIAN_POINT('Ctrl Pts',(-0.726235967997433,-1.,1.67996158455503));
#28169=CARTESIAN_POINT('Ctrl Pts',(-0.726235967997433,1.,1.67996158455503));
#28170=CARTESIAN_POINT('Ctrl Pts',(-0.731963238697195,-1.,1.69326921975743));
#28171=CARTESIAN_POINT('Ctrl Pts',(-0.731963238697195,1.,1.69326921975743));
#28172=CARTESIAN_POINT('Ctrl Pts',(-0.736799665724771,-1.,1.70473309006121));
#28173=CARTESIAN_POINT('Ctrl Pts',(-0.736799665724771,1.,1.70473309006121));
#28174=CARTESIAN_POINT('Ctrl Pts',(-0.740795162032088,-1.,1.71447789751927));
#28175=CARTESIAN_POINT('Ctrl Pts',(-0.740795162032088,1.,1.71447789751927));
#28176=CARTESIAN_POINT('Ctrl Pts',(-0.744021445433764,-1.,1.7226822991693));
#28177=CARTESIAN_POINT('Ctrl Pts',(-0.744021445433764,1.,1.7226822991693));
#28178=CARTESIAN_POINT('Ctrl Pts',(-0.746574710096436,-1.,1.72958533647399));
#28179=CARTESIAN_POINT('Ctrl Pts',(-0.746574710096436,1.,1.72958533647399));
#28180=CARTESIAN_POINT('Ctrl Pts',(-0.748582462954855,-1.,1.73550351679848));
#28181=CARTESIAN_POINT('Ctrl Pts',(-0.748582462954855,1.,1.73550351679848));
#28182=CARTESIAN_POINT('Ctrl Pts',(-0.75019343597954,-1.,1.74080458266705));
#28183=CARTESIAN_POINT('Ctrl Pts',(-0.75019343597954,1.,1.74080458266705));
#28184=CARTESIAN_POINT('Ctrl Pts',(-0.751555614163629,-1.,1.74585086852298));
#28185=CARTESIAN_POINT('Ctrl Pts',(-0.751555614163629,1.,1.74585086852298));
#28186=CARTESIAN_POINT('Ctrl Pts',(-0.752797683531377,-1.,1.75095139468809));
#28187=CARTESIAN_POINT('Ctrl Pts',(-0.752797683531377,1.,1.75095139468809));
#28188=CARTESIAN_POINT('Ctrl Pts',(-0.75400925402848,-1.,1.75631083600175));
#28189=CARTESIAN_POINT('Ctrl Pts',(-0.75400925402848,1.,1.75631083600175));
#28190=CARTESIAN_POINT('Ctrl Pts',(-0.755220979975262,-1.,1.7619781724032));
#28191=CARTESIAN_POINT('Ctrl Pts',(-0.755220979975262,1.,1.7619781724032));
#28192=CARTESIAN_POINT('Ctrl Pts',(-0.756421896028403,-1.,1.76789396003141));
#28193=CARTESIAN_POINT('Ctrl Pts',(-0.756421896028403,1.,1.76789396003141));
#28194=CARTESIAN_POINT('Ctrl Pts',(-0.757578264077238,-1.,1.77394167108342));
#28195=CARTESIAN_POINT('Ctrl Pts',(-0.757578264077238,1.,1.77394167108342));
#28196=CARTESIAN_POINT('Ctrl Pts',(-0.75865062667738,-1.,1.77999411220912));
#28197=CARTESIAN_POINT('Ctrl Pts',(-0.75865062667738,1.,1.77999411220912));
#28198=CARTESIAN_POINT('Ctrl Pts',(-0.759614401109868,-1.,1.78596964884526));
#28199=CARTESIAN_POINT('Ctrl Pts',(-0.759614401109868,1.,1.78596964884526));
#28200=CARTESIAN_POINT('Ctrl Pts',(-0.760469555880425,-1.,1.79185815610802));
#28201=CARTESIAN_POINT('Ctrl Pts',(-0.760469555880425,1.,1.79185815610802));
#28202=CARTESIAN_POINT('Ctrl Pts',(-0.761229695230359,-1.,1.79768986997735));
#28203=CARTESIAN_POINT('Ctrl Pts',(-0.761229695230359,1.,1.79768986997735));
#28204=CARTESIAN_POINT('Ctrl Pts',(-0.761915336443516,-1.,1.80351583877334));
#28205=CARTESIAN_POINT('Ctrl Pts',(-0.761915336443516,1.,1.80351583877334));
#28206=CARTESIAN_POINT('Ctrl Pts',(-0.762546129464036,-1.,1.80938551463989));
#28207=CARTESIAN_POINT('Ctrl Pts',(-0.762546129464036,1.,1.80938551463989));
#28208=CARTESIAN_POINT('Ctrl Pts',(-0.763132003836783,-1.,1.81532118405566));
#28209=CARTESIAN_POINT('Ctrl Pts',(-0.763132003836783,1.,1.81532118405566));
#28210=CARTESIAN_POINT('Ctrl Pts',(-0.763673465462854,-1.,1.82131873145297));
#28211=CARTESIAN_POINT('Ctrl Pts',(-0.763673465462854,1.,1.82131873145297));
#28212=CARTESIAN_POINT('Ctrl Pts',(-0.764165902606055,-1.,1.8273599120008));
#28213=CARTESIAN_POINT('Ctrl Pts',(-0.764165902606055,1.,1.8273599120008));
#28214=CARTESIAN_POINT('Ctrl Pts',(-0.764602549687845,-1.,1.8334207722714));
#28215=CARTESIAN_POINT('Ctrl Pts',(-0.764602549687845,1.,1.8334207722714));
#28216=CARTESIAN_POINT('Ctrl Pts',(-0.764978057881687,-1.,1.83948181064823));
#28217=CARTESIAN_POINT('Ctrl Pts',(-0.764978057881687,1.,1.83948181064823));
#28218=CARTESIAN_POINT('Ctrl Pts',(-0.765291664861971,-1.,1.8455369887591));
#28219=CARTESIAN_POINT('Ctrl Pts',(-0.765291664861971,1.,1.8455369887591));
#28220=CARTESIAN_POINT('Ctrl Pts',(-0.765545710619023,-1.,1.85158945130054));
#28221=CARTESIAN_POINT('Ctrl Pts',(-0.765545710619023,1.,1.85158945130054));
#28222=CARTESIAN_POINT('Ctrl Pts',(-0.765744212909305,-1.,1.85764741390391));
#28223=CARTESIAN_POINT('Ctrl Pts',(-0.765744212909305,1.,1.85764741390391));
#28224=CARTESIAN_POINT('Ctrl Pts',(-0.765891519092557,-1.,1.86372027063314));
#28225=CARTESIAN_POINT('Ctrl Pts',(-0.765891519092557,1.,1.86372027063314));
#28226=CARTESIAN_POINT('Ctrl Pts',(-0.765990708546111,-1.,1.86981398314345));
#28227=CARTESIAN_POINT('Ctrl Pts',(-0.765990708546111,1.,1.86981398314345));
#28228=CARTESIAN_POINT('Ctrl Pts',(-0.766042837036759,-1.,1.87592888967886));
#28229=CARTESIAN_POINT('Ctrl Pts',(-0.766042837036759,1.,1.87592888967886));
#28230=CARTESIAN_POINT('Ctrl Pts',(-0.766047794851869,-1.,1.88206215302561));
#28231=CARTESIAN_POINT('Ctrl Pts',(-0.766047794851869,1.,1.88206215302561));
#28232=CARTESIAN_POINT('Ctrl Pts',(-0.76600483706209,-1.,1.88820926433409));
#28233=CARTESIAN_POINT('Ctrl Pts',(-0.76600483706209,1.,1.88820926433409));
#28234=CARTESIAN_POINT('Ctrl Pts',(-0.765913193856979,-1.,1.89436577771389));
#28235=CARTESIAN_POINT('Ctrl Pts',(-0.765913193856979,1.,1.89436577771389));
#28236=CARTESIAN_POINT('Ctrl Pts',(-0.765772772593395,-1.,1.90052930393599));
#28237=CARTESIAN_POINT('Ctrl Pts',(-0.765772772593395,1.,1.90052930393599));
#28238=CARTESIAN_POINT('Ctrl Pts',(-0.765584196937936,-1.,1.90669961402362));
#28239=CARTESIAN_POINT('Ctrl Pts',(-0.765584196937936,1.,1.90669961402362));
#28240=CARTESIAN_POINT('Ctrl Pts',(-0.765348465884739,-1.,1.91287765805174));
#28241=CARTESIAN_POINT('Ctrl Pts',(-0.765348465884739,1.,1.91287765805174));
#28242=CARTESIAN_POINT('Ctrl Pts',(-0.765066729667095,-1.,1.91906491634197));
#28243=CARTESIAN_POINT('Ctrl Pts',(-0.765066729667095,1.,1.91906491634197));
#28244=CARTESIAN_POINT('Ctrl Pts',(-0.764740025488189,-1.,1.92526263537041));
#28245=CARTESIAN_POINT('Ctrl Pts',(-0.764740025488189,1.,1.92526263537041));
#28246=CARTESIAN_POINT('Ctrl Pts',(-0.764369010673889,-1.,1.93147105496367));
#28247=CARTESIAN_POINT('Ctrl Pts',(-0.764369010673889,1.,1.93147105496367));
#28248=CARTESIAN_POINT('Ctrl Pts',(-0.763954049121393,-1.,1.93768964875867));
#28249=CARTESIAN_POINT('Ctrl Pts',(-0.763954049121393,1.,1.93768964875867));
#28250=CARTESIAN_POINT('Ctrl Pts',(-0.76349533353858,-1.,1.94391746617626));
#28251=CARTESIAN_POINT('Ctrl Pts',(-0.76349533353858,1.,1.94391746617626));
#28252=CARTESIAN_POINT('Ctrl Pts',(-0.762992990878774,-1.,1.95015342590025));
#28253=CARTESIAN_POINT('Ctrl Pts',(-0.762992990878774,1.,1.95015342590025));
#28254=CARTESIAN_POINT('Ctrl Pts',(-0.762447203806263,-1.,1.95639665309893));
#28255=CARTESIAN_POINT('Ctrl Pts',(-0.762447203806263,1.,1.95639665309893));
#28256=CARTESIAN_POINT('Ctrl Pts',(-0.761858300014575,-1.,1.96264672744229));
#28257=CARTESIAN_POINT('Ctrl Pts',(-0.761858300014575,1.,1.96264672744229));
#28258=CARTESIAN_POINT('Ctrl Pts',(-0.761226690483986,-1.,1.96890351582545));
#28259=CARTESIAN_POINT('Ctrl Pts',(-0.761226690483986,1.,1.96890351582545));
#28260=CARTESIAN_POINT('Ctrl Pts',(-0.760552825409855,-1.,1.97516705321521));
#28261=CARTESIAN_POINT('Ctrl Pts',(-0.760552825409855,1.,1.97516705321521));
#28262=CARTESIAN_POINT('Ctrl Pts',(-0.759837147452135,-1.,1.98143741418156));
#28263=CARTESIAN_POINT('Ctrl Pts',(-0.759837147452135,1.,1.98143741418156));
#28264=CARTESIAN_POINT('Ctrl Pts',(-0.759080037802243,-1.,1.98771456680806));
#28265=CARTESIAN_POINT('Ctrl Pts',(-0.759080037802243,1.,1.98771456680806));
#28266=CARTESIAN_POINT('Ctrl Pts',(-0.758281796766377,-1.,1.9939983109871));
#28267=CARTESIAN_POINT('Ctrl Pts',(-0.758281796766377,1.,1.9939983109871));
#28268=CARTESIAN_POINT('Ctrl Pts',(-0.757442676862341,-1.,2.00028834739072));
#28269=CARTESIAN_POINT('Ctrl Pts',(-0.757442676862341,1.,2.00028834739072));
#28270=CARTESIAN_POINT('Ctrl Pts',(-0.756562904646496,-1.,2.00658431587682));
#28271=CARTESIAN_POINT('Ctrl Pts',(-0.756562904646496,1.,2.00658431587682));
#28272=CARTESIAN_POINT('Ctrl Pts',(-0.7556427049581,-1.,2.01288584328149));
#28273=CARTESIAN_POINT('Ctrl Pts',(-0.7556427049581,1.,2.01288584328149));
#28274=CARTESIAN_POINT('Ctrl Pts',(-0.75468233072352,-1.,2.01919259406003));
#28275=CARTESIAN_POINT('Ctrl Pts',(-0.75468233072352,1.,2.01919259406003));
#28276=CARTESIAN_POINT('Ctrl Pts',(-0.753682061113766,-1.,2.02550428623587));
#28277=CARTESIAN_POINT('Ctrl Pts',(-0.753682061113766,1.,2.02550428623587));
#28278=CARTESIAN_POINT('Ctrl Pts',(-0.752642180488104,-1.,2.03182068456467));
#28279=CARTESIAN_POINT('Ctrl Pts',(-0.752642180488104,1.,2.03182068456467));
#28280=CARTESIAN_POINT('Ctrl Pts',(-0.751562963361384,-1.,2.03814160092173));
#28281=CARTESIAN_POINT('Ctrl Pts',(-0.751562963361384,1.,2.03814160092173));
#28282=CARTESIAN_POINT('Ctrl Pts',(-0.750444657874758,-1.,2.04446689147754));
#28283=CARTESIAN_POINT('Ctrl Pts',(-0.750444657874758,1.,2.04446689147754));
#28284=CARTESIAN_POINT('Ctrl Pts',(-0.749287468663053,-1.,2.05079645591606));
#28285=CARTESIAN_POINT('Ctrl Pts',(-0.749287468663053,1.,2.05079645591606));
#28286=CARTESIAN_POINT('Ctrl Pts',(-0.748091554181101,-1.,2.05713023030263));
#28287=CARTESIAN_POINT('Ctrl Pts',(-0.748091554181101,1.,2.05713023030263));
#28288=CARTESIAN_POINT('Ctrl Pts',(-0.747103932785504,-1.,2.06220058927162));
#28289=CARTESIAN_POINT('Ctrl Pts',(-0.747103932785504,1.,2.06220058927162));
#28290=CARTESIAN_POINT('Ctrl Pts',(-0.746345871542696,-1.,2.06600523016401));
#28291=CARTESIAN_POINT('Ctrl Pts',(-0.746345871542696,1.,2.06600523016401));
#28292=CARTESIAN_POINT('Ctrl Pts',(-0.74583279137781,-1.,2.06854248895575));
#28293=CARTESIAN_POINT('Ctrl Pts',(-0.74583279137781,1.,2.06854248895575));
#28294=CARTESIAN_POINT('Ctrl Pts',(-0.745574324794401,-1.,2.0698113262342));
#28295=CARTESIAN_POINT('Ctrl Pts',(-0.745574324794401,1.,2.0698113262342));
#28296=CARTESIAN_POINT('',(-0.693717979106306,1.,1.60662857109684));
#28297=CARTESIAN_POINT('Ctrl Pts',(-0.693717979106306,1.,1.60662857109684));
#28298=CARTESIAN_POINT('Ctrl Pts',(-0.695712097881194,1.,1.61106790958151));
#28299=CARTESIAN_POINT('Ctrl Pts',(-0.699605146405088,1.,1.61974673472612));
#28300=CARTESIAN_POINT('Ctrl Pts',(-0.705159151988319,1.,1.63216541664676));
#28301=CARTESIAN_POINT('Ctrl Pts',(-0.711993139355394,1.,1.64752408832016));
#28302=CARTESIAN_POINT('Ctrl Pts',(-0.719585433804282,1.,1.6647288055568));
#28303=CARTESIAN_POINT('Ctrl Pts',(-0.726235967997433,1.,1.67996158455503));
#28304=CARTESIAN_POINT('Ctrl Pts',(-0.731963238697195,1.,1.69326921975743));
#28305=CARTESIAN_POINT('Ctrl Pts',(-0.736799665724771,1.,1.70473309006121));
#28306=CARTESIAN_POINT('Ctrl Pts',(-0.740795162032088,1.,1.71447789751927));
#28307=CARTESIAN_POINT('Ctrl Pts',(-0.744021445433764,1.,1.7226822991693));
#28308=CARTESIAN_POINT('Ctrl Pts',(-0.746574710096436,1.,1.72958533647399));
#28309=CARTESIAN_POINT('Ctrl Pts',(-0.748582462954855,1.,1.73550351679848));
#28310=CARTESIAN_POINT('Ctrl Pts',(-0.75019343597954,1.,1.74080458266705));
#28311=CARTESIAN_POINT('Ctrl Pts',(-0.751555614163629,1.,1.74585086852298));
#28312=CARTESIAN_POINT('Ctrl Pts',(-0.752797683531377,1.,1.75095139468809));
#28313=CARTESIAN_POINT('Ctrl Pts',(-0.75400925402848,1.,1.75631083600175));
#28314=CARTESIAN_POINT('Ctrl Pts',(-0.755220979975262,1.,1.7619781724032));
#28315=CARTESIAN_POINT('Ctrl Pts',(-0.756421896028403,1.,1.76789396003141));
#28316=CARTESIAN_POINT('Ctrl Pts',(-0.757578264077238,1.,1.77394167108342));
#28317=CARTESIAN_POINT('Ctrl Pts',(-0.75865062667738,1.,1.77999411220912));
#28318=CARTESIAN_POINT('Ctrl Pts',(-0.759614401109868,1.,1.78596964884526));
#28319=CARTESIAN_POINT('Ctrl Pts',(-0.760469555880425,1.,1.79185815610802));
#28320=CARTESIAN_POINT('Ctrl Pts',(-0.761229695230359,1.,1.79768986997735));
#28321=CARTESIAN_POINT('Ctrl Pts',(-0.761915336443516,1.,1.80351583877334));
#28322=CARTESIAN_POINT('Ctrl Pts',(-0.762546129464036,1.,1.80938551463989));
#28323=CARTESIAN_POINT('Ctrl Pts',(-0.763132003836783,1.,1.81532118405566));
#28324=CARTESIAN_POINT('Ctrl Pts',(-0.763673465462854,1.,1.82131873145297));
#28325=CARTESIAN_POINT('Ctrl Pts',(-0.764165902606055,1.,1.8273599120008));
#28326=CARTESIAN_POINT('Ctrl Pts',(-0.764602549687845,1.,1.8334207722714));
#28327=CARTESIAN_POINT('Ctrl Pts',(-0.764978057881687,1.,1.83948181064823));
#28328=CARTESIAN_POINT('Ctrl Pts',(-0.765291664861971,1.,1.8455369887591));
#28329=CARTESIAN_POINT('Ctrl Pts',(-0.765545710619023,1.,1.85158945130054));
#28330=CARTESIAN_POINT('Ctrl Pts',(-0.765744212909305,1.,1.85764741390391));
#28331=CARTESIAN_POINT('Ctrl Pts',(-0.765891519092557,1.,1.86372027063314));
#28332=CARTESIAN_POINT('Ctrl Pts',(-0.765990708546111,1.,1.86981398314345));
#28333=CARTESIAN_POINT('Ctrl Pts',(-0.766042837036759,1.,1.87592888967886));
#28334=CARTESIAN_POINT('Ctrl Pts',(-0.766047794851869,1.,1.88206215302561));
#28335=CARTESIAN_POINT('Ctrl Pts',(-0.76600483706209,1.,1.88820926433409));
#28336=CARTESIAN_POINT('Ctrl Pts',(-0.765913193856979,1.,1.89436577771389));
#28337=CARTESIAN_POINT('Ctrl Pts',(-0.765772772593395,1.,1.90052930393599));
#28338=CARTESIAN_POINT('Ctrl Pts',(-0.765584196937936,1.,1.90669961402362));
#28339=CARTESIAN_POINT('Ctrl Pts',(-0.765348465884739,1.,1.91287765805174));
#28340=CARTESIAN_POINT('Ctrl Pts',(-0.765066729667095,1.,1.91906491634197));
#28341=CARTESIAN_POINT('Ctrl Pts',(-0.764740025488189,1.,1.92526263537041));
#28342=CARTESIAN_POINT('Ctrl Pts',(-0.764369010673889,1.,1.93147105496367));
#28343=CARTESIAN_POINT('Ctrl Pts',(-0.763954049121393,1.,1.93768964875867));
#28344=CARTESIAN_POINT('Ctrl Pts',(-0.76349533353858,1.,1.94391746617626));
#28345=CARTESIAN_POINT('Ctrl Pts',(-0.762992990878774,1.,1.95015342590025));
#28346=CARTESIAN_POINT('Ctrl Pts',(-0.762447203806263,1.,1.95639665309893));
#28347=CARTESIAN_POINT('Ctrl Pts',(-0.761858300014575,1.,1.96264672744229));
#28348=CARTESIAN_POINT('Ctrl Pts',(-0.761226690483986,1.,1.96890351582545));
#28349=CARTESIAN_POINT('Ctrl Pts',(-0.760552825409855,1.,1.97516705321521));
#28350=CARTESIAN_POINT('Ctrl Pts',(-0.759837147452135,1.,1.98143741418156));
#28351=CARTESIAN_POINT('Ctrl Pts',(-0.759080037802243,1.,1.98771456680806));
#28352=CARTESIAN_POINT('Ctrl Pts',(-0.758281796766377,1.,1.9939983109871));
#28353=CARTESIAN_POINT('Ctrl Pts',(-0.757442676862341,1.,2.00028834739072));
#28354=CARTESIAN_POINT('Ctrl Pts',(-0.756562904646496,1.,2.00658431587682));
#28355=CARTESIAN_POINT('Ctrl Pts',(-0.7556427049581,1.,2.01288584328149));
#28356=CARTESIAN_POINT('Ctrl Pts',(-0.75468233072352,1.,2.01919259406003));
#28357=CARTESIAN_POINT('Ctrl Pts',(-0.753682061113766,1.,2.02550428623587));
#28358=CARTESIAN_POINT('Ctrl Pts',(-0.752642180488104,1.,2.03182068456467));
#28359=CARTESIAN_POINT('Ctrl Pts',(-0.751562963361384,1.,2.03814160092173));
#28360=CARTESIAN_POINT('Ctrl Pts',(-0.750444657874758,1.,2.04446689147754));
#28361=CARTESIAN_POINT('Ctrl Pts',(-0.749287468663053,1.,2.05079645591606));
#28362=CARTESIAN_POINT('Ctrl Pts',(-0.748091554181101,1.,2.05713023030263));
#28363=CARTESIAN_POINT('Ctrl Pts',(-0.747103932785504,1.,2.06220058927162));
#28364=CARTESIAN_POINT('Ctrl Pts',(-0.746345871542696,1.,2.06600523016401));
#28365=CARTESIAN_POINT('Ctrl Pts',(-0.74583279137781,1.,2.06854248895575));
#28366=CARTESIAN_POINT('Ctrl Pts',(-0.745574324794401,1.,2.0698113262342));
#28367=CARTESIAN_POINT('',(-0.693717979106306,0.,1.60662857109684));
#28368=CARTESIAN_POINT('Origin',(0.,0.,0.));
#28369=CARTESIAN_POINT('',(-0.892032620296855,1.,1.5055822144029));
#28370=CARTESIAN_POINT('Origin',(0.,1.,0.));
#28371=CARTESIAN_POINT('',(-0.892032620296855,0.,1.5055822144029));
#28372=CARTESIAN_POINT('Ctrl Pts',(-1.23627494547115,-1.,1.81978687191668));
#28373=CARTESIAN_POINT('Ctrl Pts',(-1.23627494547115,1.,1.81978687191668));
#28374=CARTESIAN_POINT('Ctrl Pts',(-1.23509651170476,-1.,1.81925017193666));
#28375=CARTESIAN_POINT('Ctrl Pts',(-1.23509651170476,1.,1.81925017193666));
#28376=CARTESIAN_POINT('Ctrl Pts',(-1.2327422452705,-1.,1.81817389921279));
#28377=CARTESIAN_POINT('Ctrl Pts',(-1.2327422452705,1.,1.81817389921279));
#28378=CARTESIAN_POINT('Ctrl Pts',(-1.2292186489137,-1.,1.8165508718364));
#28379=CARTESIAN_POINT('Ctrl Pts',(-1.2292186489137,1.,1.8165508718364));
#28380=CARTESIAN_POINT('Ctrl Pts',(-1.2245361330495,-1.,1.81436959210434));
#28381=CARTESIAN_POINT('Ctrl Pts',(-1.2245361330495,1.,1.81436959210434));
#28382=CARTESIAN_POINT('Ctrl Pts',(-1.21870906103557,-1.,1.81161420806656));
#28383=CARTESIAN_POINT('Ctrl Pts',(-1.21870906103557,1.,1.81161420806656));
#28384=CARTESIAN_POINT('Ctrl Pts',(-1.21290815708314,-1.,1.80882996917129));
#28385=CARTESIAN_POINT('Ctrl Pts',(-1.21290815708314,1.,1.80882996917129));
#28386=CARTESIAN_POINT('Ctrl Pts',(-1.20713356605475,-1.,1.80601678480707));
#28387=CARTESIAN_POINT('Ctrl Pts',(-1.20713356605475,1.,1.80601678480707));
#28388=CARTESIAN_POINT('Ctrl Pts',(-1.20138548938974,-1.,1.80317454838603));
#28389=CARTESIAN_POINT('Ctrl Pts',(-1.20138548938974,1.,1.80317454838603));
#28390=CARTESIAN_POINT('Ctrl Pts',(-1.19566418930242,-1.,1.80030314369879));
#28391=CARTESIAN_POINT('Ctrl Pts',(-1.19566418930242,1.,1.80030314369879));
#28392=CARTESIAN_POINT('Ctrl Pts',(-1.18996997934445,-1.,1.79740245923478));
#28393=CARTESIAN_POINT('Ctrl Pts',(-1.18996997934445,1.,1.79740245923478));
#28394=CARTESIAN_POINT('Ctrl Pts',(-1.18430321697432,-1.,1.79447240321515));
#28395=CARTESIAN_POINT('Ctrl Pts',(-1.18430321697432,1.,1.79447240321515));
#28396=CARTESIAN_POINT('Ctrl Pts',(-1.17866429440809,-1.,1.79151291552689));
#28397=CARTESIAN_POINT('Ctrl Pts',(-1.17866429440809,1.,1.79151291552689));
#28398=CARTESIAN_POINT('Ctrl Pts',(-1.17305363177328,-1.,1.78852398877616));
#28399=CARTESIAN_POINT('Ctrl Pts',(-1.17305363177328,1.,1.78852398877616));
#28400=CARTESIAN_POINT('Ctrl Pts',(-1.16747166312303,-1.,1.78550566040443));
#28401=CARTESIAN_POINT('Ctrl Pts',(-1.16747166312303,1.,1.78550566040443));
#28402=CARTESIAN_POINT('Ctrl Pts',(-1.16191881298499,-1.,1.78245795881009));
#28403=CARTESIAN_POINT('Ctrl Pts',(-1.16191881298499,1.,1.78245795881009));
#28404=CARTESIAN_POINT('Ctrl Pts',(-1.15639547194698,-1.,1.77938085564275));
#28405=CARTESIAN_POINT('Ctrl Pts',(-1.15639547194698,1.,1.77938085564275));
#28406=CARTESIAN_POINT('Ctrl Pts',(-1.15090197841515,-1.,1.7762742255701));
#28407=CARTESIAN_POINT('Ctrl Pts',(-1.15090197841515,1.,1.7762742255701));
#28408=CARTESIAN_POINT('Ctrl Pts',(-1.1454385822692,-1.,1.77313777896194));
#28409=CARTESIAN_POINT('Ctrl Pts',(-1.1454385822692,1.,1.77313777896194));
#28410=CARTESIAN_POINT('Ctrl Pts',(-1.14000548336975,-1.,1.76997111386769));
#28411=CARTESIAN_POINT('Ctrl Pts',(-1.14000548336975,1.,1.76997111386769));
#28412=CARTESIAN_POINT('Ctrl Pts',(-1.1346029180462,-1.,1.76677384551862));
#28413=CARTESIAN_POINT('Ctrl Pts',(-1.1346029180462,1.,1.76677384551862));
#28414=CARTESIAN_POINT('Ctrl Pts',(-1.12923123555075,-1.,1.7635457196617));
#28415=CARTESIAN_POINT('Ctrl Pts',(-1.12923123555075,1.,1.7635457196617));
#28416=CARTESIAN_POINT('Ctrl Pts',(-1.12389096855086,-1.,1.76028671825096));
#28417=CARTESIAN_POINT('Ctrl Pts',(-1.12389096855086,1.,1.76028671825096));
#28418=CARTESIAN_POINT('Ctrl Pts',(-1.11858293216763,-1.,1.75699720772105));
#28419=CARTESIAN_POINT('Ctrl Pts',(-1.11858293216763,1.,1.75699720772105));
#28420=CARTESIAN_POINT('Ctrl Pts',(-1.11330807582551,-1.,1.7536777209463));
#28421=CARTESIAN_POINT('Ctrl Pts',(-1.11330807582551,1.,1.7536777209463));
#28422=CARTESIAN_POINT('Ctrl Pts',(-1.10806728183007,-1.,1.7503286607592));
#28423=CARTESIAN_POINT('Ctrl Pts',(-1.10806728183007,1.,1.7503286607592));
#28424=CARTESIAN_POINT('Ctrl Pts',(-1.10286118991143,-1.,1.74695004214923));
#28425=CARTESIAN_POINT('Ctrl Pts',(-1.10286118991143,1.,1.74695004214923));
#28426=CARTESIAN_POINT('Ctrl Pts',(-1.09768999241225,-1.,1.74354119236208));
#28427=CARTESIAN_POINT('Ctrl Pts',(-1.09768999241225,1.,1.74354119236208));
#28428=CARTESIAN_POINT('Ctrl Pts',(-1.09255329056493,-1.,1.74010053962247));
#28429=CARTESIAN_POINT('Ctrl Pts',(-1.09255329056493,1.,1.74010053962247));
#28430=CARTESIAN_POINT('Ctrl Pts',(-1.08745056285427,-1.,1.73662628326091));
#28431=CARTESIAN_POINT('Ctrl Pts',(-1.08745056285427,1.,1.73662628326091));
#28432=CARTESIAN_POINT('Ctrl Pts',(-1.08238162784749,-1.,1.73311705663407));
#28433=CARTESIAN_POINT('Ctrl Pts',(-1.08238162784749,1.,1.73311705663407));
#28434=CARTESIAN_POINT('Ctrl Pts',(-1.0773470373727,-1.,1.72957248977424));
#28435=CARTESIAN_POINT('Ctrl Pts',(-1.0773470373727,1.,1.72957248977424));
#28436=CARTESIAN_POINT('Ctrl Pts',(-1.07234866990252,-1.,1.72599406198488));
#28437=CARTESIAN_POINT('Ctrl Pts',(-1.07234866990252,1.,1.72599406198488));
#28438=CARTESIAN_POINT('Ctrl Pts',(-1.06738966975462,-1.,1.72238500928453));
#28439=CARTESIAN_POINT('Ctrl Pts',(-1.06738966975462,1.,1.72238500928453));
#28440=CARTESIAN_POINT('Ctrl Pts',(-1.06247324680647,-1.,1.71874858456904));
#28441=CARTESIAN_POINT('Ctrl Pts',(-1.06247324680647,1.,1.71874858456904));
#28442=CARTESIAN_POINT('Ctrl Pts',(-1.05760163192479,-1.,1.7150865442702));
#28443=CARTESIAN_POINT('Ctrl Pts',(-1.05760163192479,1.,1.7150865442702));
#28444=CARTESIAN_POINT('Ctrl Pts',(-1.05277517202855,-1.,1.71139783543989));
#28445=CARTESIAN_POINT('Ctrl Pts',(-1.05277517202855,1.,1.71139783543989));
#28446=CARTESIAN_POINT('Ctrl Pts',(-1.04799085404995,-1.,1.70767646263649));
#28447=CARTESIAN_POINT('Ctrl Pts',(-1.04799085404995,1.,1.70767646263649));
#28448=CARTESIAN_POINT('Ctrl Pts',(-1.04324363334554,-1.,1.70391338707982));
#28449=CARTESIAN_POINT('Ctrl Pts',(-1.04324363334554,1.,1.70391338707982));
#28450=CARTESIAN_POINT('Ctrl Pts',(-1.03852922490789,-1.,1.70010052930962));
#28451=CARTESIAN_POINT('Ctrl Pts',(-1.03852922490789,1.,1.70010052930962));
#28452=CARTESIAN_POINT('Ctrl Pts',(-1.03384646003588,-1.,1.69623414782771));
#28453=CARTESIAN_POINT('Ctrl Pts',(-1.03384646003588,1.,1.69623414782771));
#28454=CARTESIAN_POINT('Ctrl Pts',(-1.02919977579147,-1.,1.69231840863458));
#28455=CARTESIAN_POINT('Ctrl Pts',(-1.02919977579147,1.,1.69231840863458));
#28456=CARTESIAN_POINT('Ctrl Pts',(-1.02460180535255,-1.,1.68836910178447));
#28457=CARTESIAN_POINT('Ctrl Pts',(-1.02460180535255,1.,1.68836910178447));
#28458=CARTESIAN_POINT('Ctrl Pts',(-1.02006795074201,-1.,1.68440578021706));
#28459=CARTESIAN_POINT('Ctrl Pts',(-1.02006795074201,1.,1.68440578021706));
#28460=CARTESIAN_POINT('Ctrl Pts',(-1.01561026162773,-1.,1.68044289894798));
#28461=CARTESIAN_POINT('Ctrl Pts',(-1.01561026162773,1.,1.68044289894798));
#28462=CARTESIAN_POINT('Ctrl Pts',(-1.01123236493511,-1.,1.67648246776464));
#28463=CARTESIAN_POINT('Ctrl Pts',(-1.01123236493511,1.,1.67648246776464));
#28464=CARTESIAN_POINT('Ctrl Pts',(-1.00692206696414,-1.,1.67250335383293));
#28465=CARTESIAN_POINT('Ctrl Pts',(-1.00692206696414,1.,1.67250335383293));
#28466=CARTESIAN_POINT('Ctrl Pts',(-1.00265091003727,-1.,1.66846059277303));
#28467=CARTESIAN_POINT('Ctrl Pts',(-1.00265091003727,1.,1.66846059277303));
#28468=CARTESIAN_POINT('Ctrl Pts',(-0.998389654952758,-1.,1.66430758030376));
#28469=CARTESIAN_POINT('Ctrl Pts',(-0.998389654952758,1.,1.66430758030376));
#28470=CARTESIAN_POINT('Ctrl Pts',(-0.994121836661306,-1.,1.66001553809947));
#28471=CARTESIAN_POINT('Ctrl Pts',(-0.994121836661306,1.,1.66001553809947));
#28472=CARTESIAN_POINT('Ctrl Pts',(-0.989855627854165,-1.,1.65559044289699));
#28473=CARTESIAN_POINT('Ctrl Pts',(-0.989855627854165,1.,1.65559044289699));
#28474=CARTESIAN_POINT('Ctrl Pts',(-0.985642622920821,-1.,1.65110016612638));
#28475=CARTESIAN_POINT('Ctrl Pts',(-0.985642622920821,1.,1.65110016612638));
#28476=CARTESIAN_POINT('Ctrl Pts',(-0.981562530939489,-1.,1.64665139190656));
#28477=CARTESIAN_POINT('Ctrl Pts',(-0.981562530939489,1.,1.64665139190656));
#28478=CARTESIAN_POINT('Ctrl Pts',(-0.977689794119416,-1.,1.64233990826687));
#28479=CARTESIAN_POINT('Ctrl Pts',(-0.977689794119416,1.,1.64233990826687));
#28480=CARTESIAN_POINT('Ctrl Pts',(-0.974066058287418,-1.,1.63820952658144));
#28481=CARTESIAN_POINT('Ctrl Pts',(-0.974066058287418,1.,1.63820952658144));
#28482=CARTESIAN_POINT('Ctrl Pts',(-0.970669715997509,-1.,1.63420665729798));
#28483=CARTESIAN_POINT('Ctrl Pts',(-0.970669715997509,1.,1.63420665729798));
#28484=CARTESIAN_POINT('Ctrl Pts',(-0.967387853230345,-1.,1.63013849959461));
#28485=CARTESIAN_POINT('Ctrl Pts',(-0.967387853230345,1.,1.63013849959461));
#28486=CARTESIAN_POINT('Ctrl Pts',(-0.964046107040536,-1.,1.62571930670187));
#28487=CARTESIAN_POINT('Ctrl Pts',(-0.964046107040536,1.,1.62571930670187));
#28488=CARTESIAN_POINT('Ctrl Pts',(-0.960438326101729,-1.,1.62061638140221));
#28489=CARTESIAN_POINT('Ctrl Pts',(-0.960438326101729,1.,1.62061638140221));
#28490=CARTESIAN_POINT('Ctrl Pts',(-0.956354422920671,-1.,1.61449324337085));
#28491=CARTESIAN_POINT('Ctrl Pts',(-0.956354422920671,1.,1.61449324337085));
#28492=CARTESIAN_POINT('Ctrl Pts',(-0.951613284356035,-1.,1.60706069896936));
#28493=CARTESIAN_POINT('Ctrl Pts',(-0.951613284356035,1.,1.60706069896936));
#28494=CARTESIAN_POINT('Ctrl Pts',(-0.946078063315257,-1.,1.59810042043673));
#28495=CARTESIAN_POINT('Ctrl Pts',(-0.946078063315257,1.,1.59810042043673));
#28496=CARTESIAN_POINT('Ctrl Pts',(-0.939646377893399,-1.,1.58744937487176));
#28497=CARTESIAN_POINT('Ctrl Pts',(-0.939646377893399,1.,1.58744937487176));
#28498=CARTESIAN_POINT('Ctrl Pts',(-0.932246680108685,-1.,1.57499388382243));
#28499=CARTESIAN_POINT('Ctrl Pts',(-0.932246680108685,1.,1.57499388382243));
#28500=CARTESIAN_POINT('Ctrl Pts',(-0.923832188944341,-1.,1.56065988578893));
#28501=CARTESIAN_POINT('Ctrl Pts',(-0.923832188944341,1.,1.56065988578893));
#28502=CARTESIAN_POINT('Ctrl Pts',(-0.914375919026456,-1.,1.54440491149498));
#28503=CARTESIAN_POINT('Ctrl Pts',(-0.914375919026456,1.,1.54440491149498));
#28504=CARTESIAN_POINT('Ctrl Pts',(-0.905967409625651,-1.,1.52984849887993));
#28505=CARTESIAN_POINT('Ctrl Pts',(-0.905967409625651,1.,1.52984849887993));
#28506=CARTESIAN_POINT('Ctrl Pts',(-0.899185047483511,-1.,1.51805569590094));
#28507=CARTESIAN_POINT('Ctrl Pts',(-0.899185047483511,1.,1.51805569590094));
#28508=CARTESIAN_POINT('Ctrl Pts',(-0.894452006964543,-1.,1.50980486806688));
#28509=CARTESIAN_POINT('Ctrl Pts',(-0.894452006964543,1.,1.50980486806688));
#28510=CARTESIAN_POINT('Ctrl Pts',(-0.892032620296855,-1.,1.5055822144029));
#28511=CARTESIAN_POINT('Ctrl Pts',(-0.892032620296855,1.,1.5055822144029));
#28512=CARTESIAN_POINT('',(-1.23627494547115,1.,1.81978687191668));
#28513=CARTESIAN_POINT('Ctrl Pts',(-1.23627494547115,1.,1.81978687191668));
#28514=CARTESIAN_POINT('Ctrl Pts',(-1.23509651170476,1.,1.81925017193666));
#28515=CARTESIAN_POINT('Ctrl Pts',(-1.2327422452705,1.,1.81817389921279));
#28516=CARTESIAN_POINT('Ctrl Pts',(-1.2292186489137,1.,1.8165508718364));
#28517=CARTESIAN_POINT('Ctrl Pts',(-1.2245361330495,1.,1.81436959210434));
#28518=CARTESIAN_POINT('Ctrl Pts',(-1.21870906103557,1.,1.81161420806656));
#28519=CARTESIAN_POINT('Ctrl Pts',(-1.21290815708314,1.,1.80882996917129));
#28520=CARTESIAN_POINT('Ctrl Pts',(-1.20713356605475,1.,1.80601678480707));
#28521=CARTESIAN_POINT('Ctrl Pts',(-1.20138548938974,1.,1.80317454838603));
#28522=CARTESIAN_POINT('Ctrl Pts',(-1.19566418930242,1.,1.80030314369879));
#28523=CARTESIAN_POINT('Ctrl Pts',(-1.18996997934445,1.,1.79740245923478));
#28524=CARTESIAN_POINT('Ctrl Pts',(-1.18430321697432,1.,1.79447240321515));
#28525=CARTESIAN_POINT('Ctrl Pts',(-1.17866429440809,1.,1.79151291552689));
#28526=CARTESIAN_POINT('Ctrl Pts',(-1.17305363177328,1.,1.78852398877616));
#28527=CARTESIAN_POINT('Ctrl Pts',(-1.16747166312303,1.,1.78550566040443));
#28528=CARTESIAN_POINT('Ctrl Pts',(-1.16191881298499,1.,1.78245795881009));
#28529=CARTESIAN_POINT('Ctrl Pts',(-1.15639547194698,1.,1.77938085564275));
#28530=CARTESIAN_POINT('Ctrl Pts',(-1.15090197841515,1.,1.7762742255701));
#28531=CARTESIAN_POINT('Ctrl Pts',(-1.1454385822692,1.,1.77313777896194));
#28532=CARTESIAN_POINT('Ctrl Pts',(-1.14000548336975,1.,1.76997111386769));
#28533=CARTESIAN_POINT('Ctrl Pts',(-1.1346029180462,1.,1.76677384551862));
#28534=CARTESIAN_POINT('Ctrl Pts',(-1.12923123555075,1.,1.7635457196617));
#28535=CARTESIAN_POINT('Ctrl Pts',(-1.12389096855086,1.,1.76028671825096));
#28536=CARTESIAN_POINT('Ctrl Pts',(-1.11858293216763,1.,1.75699720772105));
#28537=CARTESIAN_POINT('Ctrl Pts',(-1.11330807582551,1.,1.7536777209463));
#28538=CARTESIAN_POINT('Ctrl Pts',(-1.10806728183007,1.,1.7503286607592));
#28539=CARTESIAN_POINT('Ctrl Pts',(-1.10286118991143,1.,1.74695004214923));
#28540=CARTESIAN_POINT('Ctrl Pts',(-1.09768999241225,1.,1.74354119236208));
#28541=CARTESIAN_POINT('Ctrl Pts',(-1.09255329056493,1.,1.74010053962247));
#28542=CARTESIAN_POINT('Ctrl Pts',(-1.08745056285427,1.,1.73662628326091));
#28543=CARTESIAN_POINT('Ctrl Pts',(-1.08238162784749,1.,1.73311705663407));
#28544=CARTESIAN_POINT('Ctrl Pts',(-1.0773470373727,1.,1.72957248977424));
#28545=CARTESIAN_POINT('Ctrl Pts',(-1.07234866990252,1.,1.72599406198488));
#28546=CARTESIAN_POINT('Ctrl Pts',(-1.06738966975462,1.,1.72238500928453));
#28547=CARTESIAN_POINT('Ctrl Pts',(-1.06247324680647,1.,1.71874858456904));
#28548=CARTESIAN_POINT('Ctrl Pts',(-1.05760163192479,1.,1.7150865442702));
#28549=CARTESIAN_POINT('Ctrl Pts',(-1.05277517202855,1.,1.71139783543989));
#28550=CARTESIAN_POINT('Ctrl Pts',(-1.04799085404995,1.,1.70767646263649));
#28551=CARTESIAN_POINT('Ctrl Pts',(-1.04324363334554,1.,1.70391338707982));
#28552=CARTESIAN_POINT('Ctrl Pts',(-1.03852922490789,1.,1.70010052930962));
#28553=CARTESIAN_POINT('Ctrl Pts',(-1.03384646003588,1.,1.69623414782771));
#28554=CARTESIAN_POINT('Ctrl Pts',(-1.02919977579147,1.,1.69231840863458));
#28555=CARTESIAN_POINT('Ctrl Pts',(-1.02460180535255,1.,1.68836910178447));
#28556=CARTESIAN_POINT('Ctrl Pts',(-1.02006795074201,1.,1.68440578021706));
#28557=CARTESIAN_POINT('Ctrl Pts',(-1.01561026162773,1.,1.68044289894798));
#28558=CARTESIAN_POINT('Ctrl Pts',(-1.01123236493511,1.,1.67648246776464));
#28559=CARTESIAN_POINT('Ctrl Pts',(-1.00692206696414,1.,1.67250335383293));
#28560=CARTESIAN_POINT('Ctrl Pts',(-1.00265091003727,1.,1.66846059277303));
#28561=CARTESIAN_POINT('Ctrl Pts',(-0.998389654952758,1.,1.66430758030376));
#28562=CARTESIAN_POINT('Ctrl Pts',(-0.994121836661306,1.,1.66001553809947));
#28563=CARTESIAN_POINT('Ctrl Pts',(-0.989855627854165,1.,1.65559044289699));
#28564=CARTESIAN_POINT('Ctrl Pts',(-0.985642622920821,1.,1.65110016612638));
#28565=CARTESIAN_POINT('Ctrl Pts',(-0.981562530939489,1.,1.64665139190656));
#28566=CARTESIAN_POINT('Ctrl Pts',(-0.977689794119416,1.,1.64233990826687));
#28567=CARTESIAN_POINT('Ctrl Pts',(-0.974066058287418,1.,1.63820952658144));
#28568=CARTESIAN_POINT('Ctrl Pts',(-0.970669715997509,1.,1.63420665729798));
#28569=CARTESIAN_POINT('Ctrl Pts',(-0.967387853230345,1.,1.63013849959461));
#28570=CARTESIAN_POINT('Ctrl Pts',(-0.964046107040536,1.,1.62571930670187));
#28571=CARTESIAN_POINT('Ctrl Pts',(-0.960438326101729,1.,1.62061638140221));
#28572=CARTESIAN_POINT('Ctrl Pts',(-0.956354422920671,1.,1.61449324337085));
#28573=CARTESIAN_POINT('Ctrl Pts',(-0.951613284356035,1.,1.60706069896936));
#28574=CARTESIAN_POINT('Ctrl Pts',(-0.946078063315257,1.,1.59810042043673));
#28575=CARTESIAN_POINT('Ctrl Pts',(-0.939646377893399,1.,1.58744937487176));
#28576=CARTESIAN_POINT('Ctrl Pts',(-0.932246680108685,1.,1.57499388382243));
#28577=CARTESIAN_POINT('Ctrl Pts',(-0.923832188944341,1.,1.56065988578893));
#28578=CARTESIAN_POINT('Ctrl Pts',(-0.914375919026456,1.,1.54440491149498));
#28579=CARTESIAN_POINT('Ctrl Pts',(-0.905967409625651,1.,1.52984849887993));
#28580=CARTESIAN_POINT('Ctrl Pts',(-0.899185047483511,1.,1.51805569590094));
#28581=CARTESIAN_POINT('Ctrl Pts',(-0.894452006964543,1.,1.50980486806688));
#28582=CARTESIAN_POINT('Ctrl Pts',(-0.892032620296855,1.,1.5055822144029));
#28583=CARTESIAN_POINT('',(-1.23627494547115,0.,1.81978687191668));
#28584=CARTESIAN_POINT('Origin',(-1.34869019493419,0.,1.73811241238545));
#28585=CARTESIAN_POINT('',(-1.34869019493419,1.,1.73811241238545));
#28586=CARTESIAN_POINT('',(-1.23627494547115,1.,1.81978687191668));
#28587=CARTESIAN_POINT('',(-1.34869019493419,0.,1.73811241238545));
#28588=CARTESIAN_POINT('Ctrl Pts',(-1.15624053661742,-1.,1.31362392696032));
#28589=CARTESIAN_POINT('Ctrl Pts',(-1.15624053661742,1.,1.31362392696032));
#28590=CARTESIAN_POINT('Ctrl Pts',(-1.15950888730809,-1.,1.31722977216397));
#28591=CARTESIAN_POINT('Ctrl Pts',(-1.15950888730809,1.,1.31722977216397));
#28592=CARTESIAN_POINT('Ctrl Pts',(-1.16589330093588,-1.,1.32428080721772));
#28593=CARTESIAN_POINT('Ctrl Pts',(-1.16589330093588,1.,1.32428080721772));
#28594=CARTESIAN_POINT('Ctrl Pts',(-1.17501305789857,-1.,1.33437539347008));
#28595=CARTESIAN_POINT('Ctrl Pts',(-1.17501305789857,1.,1.33437539347008));
#28596=CARTESIAN_POINT('Ctrl Pts',(-1.18625865667441,-1.,1.34687054001093));
#28597=CARTESIAN_POINT('Ctrl Pts',(-1.18625865667441,1.,1.34687054001093));
#28598=CARTESIAN_POINT('Ctrl Pts',(-1.1987959077932,-1.,1.36088705043885));
#28599=CARTESIAN_POINT('Ctrl Pts',(-1.1987959077932,1.,1.36088705043885));
#28600=CARTESIAN_POINT('Ctrl Pts',(-1.20982812925645,-1.,1.37331915607905));
#28601=CARTESIAN_POINT('Ctrl Pts',(-1.20982812925645,1.,1.37331915607905));
#28602=CARTESIAN_POINT('Ctrl Pts',(-1.21938737280852,-1.,1.38420564527715));
#28603=CARTESIAN_POINT('Ctrl Pts',(-1.21938737280852,1.,1.38420564527715));
#28604=CARTESIAN_POINT('Ctrl Pts',(-1.22752961899387,-1.,1.39361389568796));
#28605=CARTESIAN_POINT('Ctrl Pts',(-1.22752961899387,1.,1.39361389568796));
#28606=CARTESIAN_POINT('Ctrl Pts',(-1.23434087290423,-1.,1.40164708206106));
#28607=CARTESIAN_POINT('Ctrl Pts',(-1.23434087290423,1.,1.40164708206106));
#28608=CARTESIAN_POINT('Ctrl Pts',(-1.23994455029534,-1.,1.40845295531283));
#28609=CARTESIAN_POINT('Ctrl Pts',(-1.23994455029534,1.,1.40845295531283));
#28610=CARTESIAN_POINT('Ctrl Pts',(-1.24450600513056,-1.,1.41422913175179));
#28611=CARTESIAN_POINT('Ctrl Pts',(-1.24450600513056,1.,1.41422913175179));
#28612=CARTESIAN_POINT('Ctrl Pts',(-1.24824430986571,-1.,1.41923722596025));
#28613=CARTESIAN_POINT('Ctrl Pts',(-1.24824430986571,1.,1.41923722596025));
#28614=CARTESIAN_POINT('Ctrl Pts',(-1.2514145557001,-1.,1.42378102115575));
#28615=CARTESIAN_POINT('Ctrl Pts',(-1.2514145557001,1.,1.42378102115575));
#28616=CARTESIAN_POINT('Ctrl Pts',(-1.25426945222639,-1.,1.42815938799387));
#28617=CARTESIAN_POINT('Ctrl Pts',(-1.25426945222639,1.,1.42815938799387));
#28618=CARTESIAN_POINT('Ctrl Pts',(-1.25702687965755,-1.,1.43262645609691));
#28619=CARTESIAN_POINT('Ctrl Pts',(-1.25702687965755,1.,1.43262645609691));
#28620=CARTESIAN_POINT('Ctrl Pts',(-1.25983531012005,-1.,1.43734919180848));
#28621=CARTESIAN_POINT('Ctrl Pts',(-1.25983531012005,1.,1.43734919180848));
#28622=CARTESIAN_POINT('Ctrl Pts',(-1.26273903323859,-1.,1.44236470511303));
#28623=CARTESIAN_POINT('Ctrl Pts',(-1.26273903323859,1.,1.44236470511303));
#28624=CARTESIAN_POINT('Ctrl Pts',(-1.26570925118868,-1.,1.44761985001662));
#28625=CARTESIAN_POINT('Ctrl Pts',(-1.26570925118868,1.,1.44761985001662));
#28626=CARTESIAN_POINT('Ctrl Pts',(-1.2686778680489,-1.,1.45301422764247));
#28627=CARTESIAN_POINT('Ctrl Pts',(-1.2686778680489,1.,1.45301422764247));
#28628=CARTESIAN_POINT('Ctrl Pts',(-1.27156805265289,-1.,1.45843906294697));
#28629=CARTESIAN_POINT('Ctrl Pts',(-1.27156805265289,1.,1.45843906294697));
#28630=CARTESIAN_POINT('Ctrl Pts',(-1.27433119897822,-1.,1.46382431332476));
#28631=CARTESIAN_POINT('Ctrl Pts',(-1.27433119897822,1.,1.46382431332476));
#28632=CARTESIAN_POINT('Ctrl Pts',(-1.27696414831089,-1.,1.46916035917133));
#28633=CARTESIAN_POINT('Ctrl Pts',(-1.27696414831089,1.,1.46916035917133));
#28634=CARTESIAN_POINT('Ctrl Pts',(-1.2794891824849,-1.,1.4744717526707));
#28635=CARTESIAN_POINT('Ctrl Pts',(-1.2794891824849,1.,1.4744717526707));
#28636=CARTESIAN_POINT('Ctrl Pts',(-1.28194158939517,-1.,1.47980070347095));
#28637=CARTESIAN_POINT('Ctrl Pts',(-1.28194158939517,1.,1.47980070347095));
#28638=CARTESIAN_POINT('Ctrl Pts',(-1.28435533880201,-1.,1.4851881711891));
#28639=CARTESIAN_POINT('Ctrl Pts',(-1.28435533880201,1.,1.4851881711891));
#28640=CARTESIAN_POINT('Ctrl Pts',(-1.2867467611644,-1.,1.4906522831278));
#28641=CARTESIAN_POINT('Ctrl Pts',(-1.2867467611644,1.,1.4906522831278));
#28642=CARTESIAN_POINT('Ctrl Pts',(-1.28911506584254,-1.,1.49618896881754));
#28643=CARTESIAN_POINT('Ctrl Pts',(-1.28911506584254,1.,1.49618896881754));
#28644=CARTESIAN_POINT('Ctrl Pts',(-1.29145022885181,-1.,1.50178230149776));
#28645=CARTESIAN_POINT('Ctrl Pts',(-1.29145022885181,1.,1.50178230149776));
#28646=CARTESIAN_POINT('Ctrl Pts',(-1.29373841372842,-1.,1.50741159078365));
#28647=CARTESIAN_POINT('Ctrl Pts',(-1.29373841372842,1.,1.50741159078365));
#28648=CARTESIAN_POINT('Ctrl Pts',(-1.29596850710509,-1.,1.51305994241402));
#28649=CARTESIAN_POINT('Ctrl Pts',(-1.29596850710509,1.,1.51305994241402));
#28650=CARTESIAN_POINT('Ctrl Pts',(-1.29813791800747,-1.,1.51872184912724));
#28651=CARTESIAN_POINT('Ctrl Pts',(-1.29813791800747,1.,1.51872184912724));
#28652=CARTESIAN_POINT('Ctrl Pts',(-1.30024984366328,-1.,1.52439957861062));
#28653=CARTESIAN_POINT('Ctrl Pts',(-1.30024984366328,1.,1.52439957861062));
#28654=CARTESIAN_POINT('Ctrl Pts',(-1.30231064395568,-1.,1.53009970283891));
#28655=CARTESIAN_POINT('Ctrl Pts',(-1.30231064395568,1.,1.53009970283891));
#28656=CARTESIAN_POINT('Ctrl Pts',(-1.30432735639489,-1.,1.53582981268977));
#28657=CARTESIAN_POINT('Ctrl Pts',(-1.30432735639489,1.,1.53582981268977));
#28658=CARTESIAN_POINT('Ctrl Pts',(-1.30630475189556,-1.,1.54159462645432));
#28659=CARTESIAN_POINT('Ctrl Pts',(-1.30630475189556,1.,1.54159462645432));
#28660=CARTESIAN_POINT('Ctrl Pts',(-1.30824393907473,-1.,1.54739413957185));
#28661=CARTESIAN_POINT('Ctrl Pts',(-1.30824393907473,1.,1.54739413957185));
#28662=CARTESIAN_POINT('Ctrl Pts',(-1.31014393684222,-1.,1.55322568759481));
#28663=CARTESIAN_POINT('Ctrl Pts',(-1.31014393684222,1.,1.55322568759481));
#28664=CARTESIAN_POINT('Ctrl Pts',(-1.31200264341696,-1.,1.55908521254821));
#28665=CARTESIAN_POINT('Ctrl Pts',(-1.31200264341696,1.,1.55908521254821));
#28666=CARTESIAN_POINT('Ctrl Pts',(-1.31381795281002,-1.,1.56496872402353));
#28667=CARTESIAN_POINT('Ctrl Pts',(-1.31381795281002,1.,1.56496872402353));
#28668=CARTESIAN_POINT('Ctrl Pts',(-1.31558903860016,-1.,1.57087397835723));
#28669=CARTESIAN_POINT('Ctrl Pts',(-1.31558903860016,1.,1.57087397835723));
#28670=CARTESIAN_POINT('Ctrl Pts',(-1.31731642317187,-1.,1.5768005650559));
#28671=CARTESIAN_POINT('Ctrl Pts',(-1.31731642317187,1.,1.5768005650559));
#28672=CARTESIAN_POINT('Ctrl Pts',(-1.31900135021432,-1.,1.58274907898834));
#28673=CARTESIAN_POINT('Ctrl Pts',(-1.31900135021432,1.,1.58274907898834));
#28674=CARTESIAN_POINT('Ctrl Pts',(-1.32064537110892,-1.,1.58872057258245));
#28675=CARTESIAN_POINT('Ctrl Pts',(-1.32064537110892,1.,1.58872057258245));
#28676=CARTESIAN_POINT('Ctrl Pts',(-1.32224985747682,-1.,1.59471591079403));
#28677=CARTESIAN_POINT('Ctrl Pts',(-1.32224985747682,1.,1.59471591079403));
#28678=CARTESIAN_POINT('Ctrl Pts',(-1.32381550858256,-1.,1.60073511858687));
#28679=CARTESIAN_POINT('Ctrl Pts',(-1.32381550858256,1.,1.60073511858687));
#28680=CARTESIAN_POINT('Ctrl Pts',(-1.32534250785782,-1.,1.60677758290954));
#28681=CARTESIAN_POINT('Ctrl Pts',(-1.32534250785782,1.,1.60677758290954));
#28682=CARTESIAN_POINT('Ctrl Pts',(-1.32683074483356,-1.,1.6128423401575));
#28683=CARTESIAN_POINT('Ctrl Pts',(-1.32683074483356,1.,1.6128423401575));
#28684=CARTESIAN_POINT('Ctrl Pts',(-1.32828000610449,-1.,1.61892832270724));
#28685=CARTESIAN_POINT('Ctrl Pts',(-1.32828000610449,1.,1.61892832270724));
#28686=CARTESIAN_POINT('Ctrl Pts',(-1.3296901950568,-1.,1.62503464209797));
#28687=CARTESIAN_POINT('Ctrl Pts',(-1.3296901950568,1.,1.62503464209797));
#28688=CARTESIAN_POINT('Ctrl Pts',(-1.33106149345645,-1.,1.63116079730923));
#28689=CARTESIAN_POINT('Ctrl Pts',(-1.33106149345645,1.,1.63116079730923));
#28690=CARTESIAN_POINT('Ctrl Pts',(-1.33239425103724,-1.,1.63730653475089));
#28691=CARTESIAN_POINT('Ctrl Pts',(-1.33239425103724,1.,1.63730653475089));
#28692=CARTESIAN_POINT('Ctrl Pts',(-1.33368890676572,-1.,1.6434717485603));
#28693=CARTESIAN_POINT('Ctrl Pts',(-1.33368890676572,1.,1.6434717485603));
#28694=CARTESIAN_POINT('Ctrl Pts',(-1.33494590467993,-1.,1.6496563728683));
#28695=CARTESIAN_POINT('Ctrl Pts',(-1.33494590467993,1.,1.6496563728683));
#28696=CARTESIAN_POINT('Ctrl Pts',(-1.33616559745172,-1.,1.65586025952593));
#28697=CARTESIAN_POINT('Ctrl Pts',(-1.33616559745172,1.,1.65586025952593));
#28698=CARTESIAN_POINT('Ctrl Pts',(-1.33734820885262,-1.,1.66208312541983));
#28699=CARTESIAN_POINT('Ctrl Pts',(-1.33734820885262,1.,1.66208312541983));
#28700=CARTESIAN_POINT('Ctrl Pts',(-1.33849388654388,-1.,1.66832460783989));
#28701=CARTESIAN_POINT('Ctrl Pts',(-1.33849388654388,1.,1.66832460783989));
#28702=CARTESIAN_POINT('Ctrl Pts',(-1.3396027347034,-1.,1.67458429426086));
#28703=CARTESIAN_POINT('Ctrl Pts',(-1.3396027347034,1.,1.67458429426086));
#28704=CARTESIAN_POINT('Ctrl Pts',(-1.34067485185203,-1.,1.68086176030362));
#28705=CARTESIAN_POINT('Ctrl Pts',(-1.34067485185203,1.,1.68086176030362));
#28706=CARTESIAN_POINT('Ctrl Pts',(-1.341710374848,-1.,1.68715660868764));
#28707=CARTESIAN_POINT('Ctrl Pts',(-1.341710374848,1.,1.68715660868764));
#28708=CARTESIAN_POINT('Ctrl Pts',(-1.34270948206319,-1.,1.6934684849687));
#28709=CARTESIAN_POINT('Ctrl Pts',(-1.34270948206319,1.,1.6934684849687));
#28710=CARTESIAN_POINT('Ctrl Pts',(-1.34367237124483,-1.,1.69979707754427));
#28711=CARTESIAN_POINT('Ctrl Pts',(-1.34367237124483,1.,1.69979707754427));
#28712=CARTESIAN_POINT('Ctrl Pts',(-1.34459924533831,-1.,1.70614212266738));
#28713=CARTESIAN_POINT('Ctrl Pts',(-1.34459924533831,1.,1.70614212266738));
#28714=CARTESIAN_POINT('Ctrl Pts',(-1.34549029589416,-1.,1.71250340686822));
#28715=CARTESIAN_POINT('Ctrl Pts',(-1.34549029589416,1.,1.71250340686822));
#28716=CARTESIAN_POINT('Ctrl Pts',(-1.34634568653227,-1.,1.7188807715049));
#28717=CARTESIAN_POINT('Ctrl Pts',(-1.34634568653227,1.,1.7188807715049));
#28718=CARTESIAN_POINT('Ctrl Pts',(-1.34716554819527,-1.,1.72527410680674));
#28719=CARTESIAN_POINT('Ctrl Pts',(-1.34716554819527,1.,1.72527410680674));
#28720=CARTESIAN_POINT('Ctrl Pts',(-1.34779309152035,-1.,1.7304014965394));
#28721=CARTESIAN_POINT('Ctrl Pts',(-1.34779309152035,1.,1.7304014965394));
#28722=CARTESIAN_POINT('Ctrl Pts',(-1.34824783112887,-1.,1.73425417885907));
#28723=CARTESIAN_POINT('Ctrl Pts',(-1.34824783112887,1.,1.73425417885907));
#28724=CARTESIAN_POINT('Ctrl Pts',(-1.34854391898045,-1.,1.73682580585691));
#28725=CARTESIAN_POINT('Ctrl Pts',(-1.34854391898045,1.,1.73682580585691));
#28726=CARTESIAN_POINT('Ctrl Pts',(-1.34869019493419,-1.,1.73811241238545));
#28727=CARTESIAN_POINT('Ctrl Pts',(-1.34869019493419,1.,1.73811241238545));
#28728=CARTESIAN_POINT('',(-1.15624053661742,1.,1.31362392696032));
#28729=CARTESIAN_POINT('Ctrl Pts',(-1.15624053661742,1.,1.31362392696032));
#28730=CARTESIAN_POINT('Ctrl Pts',(-1.15950888730809,1.,1.31722977216397));
#28731=CARTESIAN_POINT('Ctrl Pts',(-1.16589330093588,1.,1.32428080721772));
#28732=CARTESIAN_POINT('Ctrl Pts',(-1.17501305789857,1.,1.33437539347008));
#28733=CARTESIAN_POINT('Ctrl Pts',(-1.18625865667441,1.,1.34687054001093));
#28734=CARTESIAN_POINT('Ctrl Pts',(-1.1987959077932,1.,1.36088705043885));
#28735=CARTESIAN_POINT('Ctrl Pts',(-1.20982812925645,1.,1.37331915607905));
#28736=CARTESIAN_POINT('Ctrl Pts',(-1.21938737280852,1.,1.38420564527715));
#28737=CARTESIAN_POINT('Ctrl Pts',(-1.22752961899387,1.,1.39361389568796));
#28738=CARTESIAN_POINT('Ctrl Pts',(-1.23434087290423,1.,1.40164708206106));
#28739=CARTESIAN_POINT('Ctrl Pts',(-1.23994455029534,1.,1.40845295531283));
#28740=CARTESIAN_POINT('Ctrl Pts',(-1.24450600513056,1.,1.41422913175179));
#28741=CARTESIAN_POINT('Ctrl Pts',(-1.24824430986571,1.,1.41923722596025));
#28742=CARTESIAN_POINT('Ctrl Pts',(-1.2514145557001,1.,1.42378102115575));
#28743=CARTESIAN_POINT('Ctrl Pts',(-1.25426945222639,1.,1.42815938799387));
#28744=CARTESIAN_POINT('Ctrl Pts',(-1.25702687965755,1.,1.43262645609691));
#28745=CARTESIAN_POINT('Ctrl Pts',(-1.25983531012005,1.,1.43734919180848));
#28746=CARTESIAN_POINT('Ctrl Pts',(-1.26273903323859,1.,1.44236470511303));
#28747=CARTESIAN_POINT('Ctrl Pts',(-1.26570925118868,1.,1.44761985001662));
#28748=CARTESIAN_POINT('Ctrl Pts',(-1.2686778680489,1.,1.45301422764247));
#28749=CARTESIAN_POINT('Ctrl Pts',(-1.27156805265289,1.,1.45843906294697));
#28750=CARTESIAN_POINT('Ctrl Pts',(-1.27433119897822,1.,1.46382431332476));
#28751=CARTESIAN_POINT('Ctrl Pts',(-1.27696414831089,1.,1.46916035917133));
#28752=CARTESIAN_POINT('Ctrl Pts',(-1.2794891824849,1.,1.4744717526707));
#28753=CARTESIAN_POINT('Ctrl Pts',(-1.28194158939517,1.,1.47980070347095));
#28754=CARTESIAN_POINT('Ctrl Pts',(-1.28435533880201,1.,1.4851881711891));
#28755=CARTESIAN_POINT('Ctrl Pts',(-1.2867467611644,1.,1.4906522831278));
#28756=CARTESIAN_POINT('Ctrl Pts',(-1.28911506584254,1.,1.49618896881754));
#28757=CARTESIAN_POINT('Ctrl Pts',(-1.29145022885181,1.,1.50178230149776));
#28758=CARTESIAN_POINT('Ctrl Pts',(-1.29373841372842,1.,1.50741159078365));
#28759=CARTESIAN_POINT('Ctrl Pts',(-1.29596850710509,1.,1.51305994241402));
#28760=CARTESIAN_POINT('Ctrl Pts',(-1.29813791800747,1.,1.51872184912724));
#28761=CARTESIAN_POINT('Ctrl Pts',(-1.30024984366328,1.,1.52439957861062));
#28762=CARTESIAN_POINT('Ctrl Pts',(-1.30231064395568,1.,1.53009970283891));
#28763=CARTESIAN_POINT('Ctrl Pts',(-1.30432735639489,1.,1.53582981268977));
#28764=CARTESIAN_POINT('Ctrl Pts',(-1.30630475189556,1.,1.54159462645432));
#28765=CARTESIAN_POINT('Ctrl Pts',(-1.30824393907473,1.,1.54739413957185));
#28766=CARTESIAN_POINT('Ctrl Pts',(-1.31014393684222,1.,1.55322568759481));
#28767=CARTESIAN_POINT('Ctrl Pts',(-1.31200264341696,1.,1.55908521254821));
#28768=CARTESIAN_POINT('Ctrl Pts',(-1.31381795281002,1.,1.56496872402353));
#28769=CARTESIAN_POINT('Ctrl Pts',(-1.31558903860016,1.,1.57087397835723));
#28770=CARTESIAN_POINT('Ctrl Pts',(-1.31731642317187,1.,1.5768005650559));
#28771=CARTESIAN_POINT('Ctrl Pts',(-1.31900135021432,1.,1.58274907898834));
#28772=CARTESIAN_POINT('Ctrl Pts',(-1.32064537110892,1.,1.58872057258245));
#28773=CARTESIAN_POINT('Ctrl Pts',(-1.32224985747682,1.,1.59471591079403));
#28774=CARTESIAN_POINT('Ctrl Pts',(-1.32381550858256,1.,1.60073511858687));
#28775=CARTESIAN_POINT('Ctrl Pts',(-1.32534250785782,1.,1.60677758290954));
#28776=CARTESIAN_POINT('Ctrl Pts',(-1.32683074483356,1.,1.6128423401575));
#28777=CARTESIAN_POINT('Ctrl Pts',(-1.32828000610449,1.,1.61892832270724));
#28778=CARTESIAN_POINT('Ctrl Pts',(-1.3296901950568,1.,1.62503464209797));
#28779=CARTESIAN_POINT('Ctrl Pts',(-1.33106149345645,1.,1.63116079730923));
#28780=CARTESIAN_POINT('Ctrl Pts',(-1.33239425103724,1.,1.63730653475089));
#28781=CARTESIAN_POINT('Ctrl Pts',(-1.33368890676572,1.,1.6434717485603));
#28782=CARTESIAN_POINT('Ctrl Pts',(-1.33494590467993,1.,1.6496563728683));
#28783=CARTESIAN_POINT('Ctrl Pts',(-1.33616559745172,1.,1.65586025952593));
#28784=CARTESIAN_POINT('Ctrl Pts',(-1.33734820885262,1.,1.66208312541983));
#28785=CARTESIAN_POINT('Ctrl Pts',(-1.33849388654388,1.,1.66832460783989));
#28786=CARTESIAN_POINT('Ctrl Pts',(-1.3396027347034,1.,1.67458429426086));
#28787=CARTESIAN_POINT('Ctrl Pts',(-1.34067485185203,1.,1.68086176030362));
#28788=CARTESIAN_POINT('Ctrl Pts',(-1.341710374848,1.,1.68715660868764));
#28789=CARTESIAN_POINT('Ctrl Pts',(-1.34270948206319,1.,1.6934684849687));
#28790=CARTESIAN_POINT('Ctrl Pts',(-1.34367237124483,1.,1.69979707754427));
#28791=CARTESIAN_POINT('Ctrl Pts',(-1.34459924533831,1.,1.70614212266738));
#28792=CARTESIAN_POINT('Ctrl Pts',(-1.34549029589416,1.,1.71250340686822));
#28793=CARTESIAN_POINT('Ctrl Pts',(-1.34634568653227,1.,1.7188807715049));
#28794=CARTESIAN_POINT('Ctrl Pts',(-1.34716554819527,1.,1.72527410680674));
#28795=CARTESIAN_POINT('Ctrl Pts',(-1.34779309152035,1.,1.7304014965394));
#28796=CARTESIAN_POINT('Ctrl Pts',(-1.34824783112887,1.,1.73425417885907));
#28797=CARTESIAN_POINT('Ctrl Pts',(-1.34854391898045,1.,1.73682580585691));
#28798=CARTESIAN_POINT('Ctrl Pts',(-1.34869019493419,1.,1.73811241238545));
#28799=CARTESIAN_POINT('',(-1.15624053661742,0.,1.31362392696032));
#28800=CARTESIAN_POINT('Origin',(0.,0.,0.));
#28801=CARTESIAN_POINT('',(-1.31362392696033,1.,1.15624053661742));
#28802=CARTESIAN_POINT('Origin',(0.,1.,0.));
#28803=CARTESIAN_POINT('',(-1.31362392696033,0.,1.15624053661742));
#28804=CARTESIAN_POINT('Ctrl Pts',(-1.73811241238545,-1.,1.34869019493419));
#28805=CARTESIAN_POINT('Ctrl Pts',(-1.73811241238545,1.,1.34869019493419));
#28806=CARTESIAN_POINT('Ctrl Pts',(-1.73682580585819,-1.,1.34854391898145));
#28807=CARTESIAN_POINT('Ctrl Pts',(-1.73682580585819,1.,1.34854391898145));
#28808=CARTESIAN_POINT('Ctrl Pts',(-1.73425417886255,-1.,1.34824783113158));
#28809=CARTESIAN_POINT('Ctrl Pts',(-1.73425417886255,1.,1.34824783113158));
#28810=CARTESIAN_POINT('Ctrl Pts',(-1.73040149654497,-1.,1.3477930915247));
#28811=CARTESIAN_POINT('Ctrl Pts',(-1.73040149654497,1.,1.3477930915247));
#28812=CARTESIAN_POINT('Ctrl Pts',(-1.72527410681298,-1.,1.34716554820013));
#28813=CARTESIAN_POINT('Ctrl Pts',(-1.72527410681298,1.,1.34716554820013));
#28814=CARTESIAN_POINT('Ctrl Pts',(-1.7188807715095,-1.,1.34634568653586));
#28815=CARTESIAN_POINT('Ctrl Pts',(-1.7188807715095,1.,1.34634568653586));
#28816=CARTESIAN_POINT('Ctrl Pts',(-1.71250340687011,-1.,1.34549029589563));
#28817=CARTESIAN_POINT('Ctrl Pts',(-1.71250340687011,1.,1.34549029589563));
#28818=CARTESIAN_POINT('Ctrl Pts',(-1.70614212266676,-1.,1.34459924533783));
#28819=CARTESIAN_POINT('Ctrl Pts',(-1.70614212266676,1.,1.34459924533783));
#28820=CARTESIAN_POINT('Ctrl Pts',(-1.69979707754221,-1.,1.34367237124322));
#28821=CARTESIAN_POINT('Ctrl Pts',(-1.69979707754221,1.,1.34367237124322));
#28822=CARTESIAN_POINT('Ctrl Pts',(-1.6934684849664,-1.,1.34270948206139));
#28823=CARTESIAN_POINT('Ctrl Pts',(-1.6934684849664,1.,1.34270948206139));
#28824=CARTESIAN_POINT('Ctrl Pts',(-1.68715660868602,-1.,1.34171037484673));
#28825=CARTESIAN_POINT('Ctrl Pts',(-1.68715660868602,1.,1.34171037484673));
#28826=CARTESIAN_POINT('Ctrl Pts',(-1.68086176030308,-1.,1.3406748518516));
#28827=CARTESIAN_POINT('Ctrl Pts',(-1.68086176030308,1.,1.3406748518516));
#28828=CARTESIAN_POINT('Ctrl Pts',(-1.67458429426126,-1.,1.33960273470372));
#28829=CARTESIAN_POINT('Ctrl Pts',(-1.67458429426126,1.,1.33960273470372));
#28830=CARTESIAN_POINT('Ctrl Pts',(-1.66832460784078,-1.,1.33849388654458));
#28831=CARTESIAN_POINT('Ctrl Pts',(-1.66832460784078,1.,1.33849388654458));
#28832=CARTESIAN_POINT('Ctrl Pts',(-1.66208312542073,-1.,1.33734820885331));
#28833=CARTESIAN_POINT('Ctrl Pts',(-1.66208312542073,1.,1.33734820885331));
#28834=CARTESIAN_POINT('Ctrl Pts',(-1.65586025952651,-1.,1.33616559745217));
#28835=CARTESIAN_POINT('Ctrl Pts',(-1.65586025952651,1.,1.33616559745217));
#28836=CARTESIAN_POINT('Ctrl Pts',(-1.64965637286843,-1.,1.33494590468003));
#28837=CARTESIAN_POINT('Ctrl Pts',(-1.64965637286843,1.,1.33494590468003));
#28838=CARTESIAN_POINT('Ctrl Pts',(-1.64347174856007,-1.,1.33368890676554));
#28839=CARTESIAN_POINT('Ctrl Pts',(-1.64347174856007,1.,1.33368890676554));
#28840=CARTESIAN_POINT('Ctrl Pts',(-1.6373065347505,-1.,1.33239425103694));
#28841=CARTESIAN_POINT('Ctrl Pts',(-1.6373065347505,1.,1.33239425103694));
#28842=CARTESIAN_POINT('Ctrl Pts',(-1.63116079730887,-1.,1.33106149345618));
#28843=CARTESIAN_POINT('Ctrl Pts',(-1.63116079730887,1.,1.33106149345618));
#28844=CARTESIAN_POINT('Ctrl Pts',(-1.62503464209777,-1.,1.32969019505665));
#28845=CARTESIAN_POINT('Ctrl Pts',(-1.62503464209777,1.,1.32969019505665));
#28846=CARTESIAN_POINT('Ctrl Pts',(-1.61892832270723,-1.,1.32828000610448));
#28847=CARTESIAN_POINT('Ctrl Pts',(-1.61892832270723,1.,1.32828000610448));
#28848=CARTESIAN_POINT('Ctrl Pts',(-1.61284234015762,-1.,1.32683074483365));
#28849=CARTESIAN_POINT('Ctrl Pts',(-1.61284234015762,1.,1.32683074483365));
#28850=CARTESIAN_POINT('Ctrl Pts',(-1.6067775829097,-1.,1.32534250785794));
#28851=CARTESIAN_POINT('Ctrl Pts',(-1.6067775829097,1.,1.32534250785794));
#28852=CARTESIAN_POINT('Ctrl Pts',(-1.600735118587,-1.,1.32381550858266));
#28853=CARTESIAN_POINT('Ctrl Pts',(-1.600735118587,1.,1.32381550858266));
#28854=CARTESIAN_POINT('Ctrl Pts',(-1.59471591079408,-1.,1.32224985747686));
#28855=CARTESIAN_POINT('Ctrl Pts',(-1.59471591079408,1.,1.32224985747686));
#28856=CARTESIAN_POINT('Ctrl Pts',(-1.58872057258244,-1.,1.32064537110891));
#28857=CARTESIAN_POINT('Ctrl Pts',(-1.58872057258244,1.,1.32064537110891));
#28858=CARTESIAN_POINT('Ctrl Pts',(-1.58274907898829,-1.,1.31900135021428));
#28859=CARTESIAN_POINT('Ctrl Pts',(-1.58274907898829,1.,1.31900135021428));
#28860=CARTESIAN_POINT('Ctrl Pts',(-1.57680056505585,-1.,1.31731642317183));
#28861=CARTESIAN_POINT('Ctrl Pts',(-1.57680056505585,1.,1.31731642317183));
#28862=CARTESIAN_POINT('Ctrl Pts',(-1.57087397835721,-1.,1.31558903860015));
#28863=CARTESIAN_POINT('Ctrl Pts',(-1.57087397835721,1.,1.31558903860015));
#28864=CARTESIAN_POINT('Ctrl Pts',(-1.56496872402352,-1.,1.31381795281002));
#28865=CARTESIAN_POINT('Ctrl Pts',(-1.56496872402352,1.,1.31381795281002));
#28866=CARTESIAN_POINT('Ctrl Pts',(-1.55908521254822,-1.,1.31200264341696));
#28867=CARTESIAN_POINT('Ctrl Pts',(-1.55908521254822,1.,1.31200264341696));
#28868=CARTESIAN_POINT('Ctrl Pts',(-1.55322568759481,-1.,1.31014393684221));
#28869=CARTESIAN_POINT('Ctrl Pts',(-1.55322568759481,1.,1.31014393684221));
#28870=CARTESIAN_POINT('Ctrl Pts',(-1.54739413957183,-1.,1.30824393907471));
#28871=CARTESIAN_POINT('Ctrl Pts',(-1.54739413957183,1.,1.30824393907471));
#28872=CARTESIAN_POINT('Ctrl Pts',(-1.54159462645428,-1.,1.30630475189553));
#28873=CARTESIAN_POINT('Ctrl Pts',(-1.54159462645428,1.,1.30630475189553));
#28874=CARTESIAN_POINT('Ctrl Pts',(-1.53582981268976,-1.,1.30432735639487));
#28875=CARTESIAN_POINT('Ctrl Pts',(-1.53582981268976,1.,1.30432735639487));
#28876=CARTESIAN_POINT('Ctrl Pts',(-1.53009970283893,-1.,1.3023106439557));
#28877=CARTESIAN_POINT('Ctrl Pts',(-1.53009970283893,1.,1.3023106439557));
#28878=CARTESIAN_POINT('Ctrl Pts',(-1.5243995786107,-1.,1.30024984366334));
#28879=CARTESIAN_POINT('Ctrl Pts',(-1.5243995786107,1.,1.30024984366334));
#28880=CARTESIAN_POINT('Ctrl Pts',(-1.51872184912735,-1.,1.29813791800757));
#28881=CARTESIAN_POINT('Ctrl Pts',(-1.51872184912735,1.,1.29813791800757));
#28882=CARTESIAN_POINT('Ctrl Pts',(-1.51305994241412,-1.,1.29596850710518));
#28883=CARTESIAN_POINT('Ctrl Pts',(-1.51305994241412,1.,1.29596850710518));
#28884=CARTESIAN_POINT('Ctrl Pts',(-1.50741159078367,-1.,1.29373841372843));
#28885=CARTESIAN_POINT('Ctrl Pts',(-1.50741159078367,1.,1.29373841372843));
#28886=CARTESIAN_POINT('Ctrl Pts',(-1.50178230149764,-1.,1.29145022885171));
#28887=CARTESIAN_POINT('Ctrl Pts',(-1.50178230149764,1.,1.29145022885171));
#28888=CARTESIAN_POINT('Ctrl Pts',(-1.49618896881729,-1.,1.28911506584232));
#28889=CARTESIAN_POINT('Ctrl Pts',(-1.49618896881729,1.,1.28911506584232));
#28890=CARTESIAN_POINT('Ctrl Pts',(-1.4906522831275,-1.,1.28674676116415));
#28891=CARTESIAN_POINT('Ctrl Pts',(-1.4906522831275,1.,1.28674676116415));
#28892=CARTESIAN_POINT('Ctrl Pts',(-1.48518817118891,-1.,1.28435533880184));
#28893=CARTESIAN_POINT('Ctrl Pts',(-1.48518817118891,1.,1.28435533880184));
#28894=CARTESIAN_POINT('Ctrl Pts',(-1.47980070347102,-1.,1.28194158939522));
#28895=CARTESIAN_POINT('Ctrl Pts',(-1.47980070347102,1.,1.28194158939522));
#28896=CARTESIAN_POINT('Ctrl Pts',(-1.4744717526711,-1.,1.27948918248524));
#28897=CARTESIAN_POINT('Ctrl Pts',(-1.4744717526711,1.,1.27948918248524));
#28898=CARTESIAN_POINT('Ctrl Pts',(-1.46916035917197,-1.,1.27696414831144));
#28899=CARTESIAN_POINT('Ctrl Pts',(-1.46916035917197,1.,1.27696414831144));
#28900=CARTESIAN_POINT('Ctrl Pts',(-1.4638243133254,-1.,1.27433119897877));
#28901=CARTESIAN_POINT('Ctrl Pts',(-1.4638243133254,1.,1.27433119897877));
#28902=CARTESIAN_POINT('Ctrl Pts',(-1.45843906294725,-1.,1.27156805265312));
#28903=CARTESIAN_POINT('Ctrl Pts',(-1.45843906294725,1.,1.27156805265312));
#28904=CARTESIAN_POINT('Ctrl Pts',(-1.45301422764205,-1.,1.26867786804854));
#28905=CARTESIAN_POINT('Ctrl Pts',(-1.45301422764205,1.,1.26867786804854));
#28906=CARTESIAN_POINT('Ctrl Pts',(-1.44761985001544,-1.,1.26570925118767));
#28907=CARTESIAN_POINT('Ctrl Pts',(-1.44761985001544,1.,1.26570925118767));
#28908=CARTESIAN_POINT('Ctrl Pts',(-1.44236470511145,-1.,1.26273903323723));
#28909=CARTESIAN_POINT('Ctrl Pts',(-1.44236470511145,1.,1.26273903323723));
#28910=CARTESIAN_POINT('Ctrl Pts',(-1.43734919180719,-1.,1.25983531011894));
#28911=CARTESIAN_POINT('Ctrl Pts',(-1.43734919180719,1.,1.25983531011894));
#28912=CARTESIAN_POINT('Ctrl Pts',(-1.43262645609679,-1.,1.25702687965744));
#28913=CARTESIAN_POINT('Ctrl Pts',(-1.43262645609679,1.,1.25702687965744));
#28914=CARTESIAN_POINT('Ctrl Pts',(-1.42815938799555,-1.,1.25426945222783));
#28915=CARTESIAN_POINT('Ctrl Pts',(-1.42815938799555,1.,1.25426945222783));
#28916=CARTESIAN_POINT('Ctrl Pts',(-1.42378102115911,-1.,1.25141455570299));
#28917=CARTESIAN_POINT('Ctrl Pts',(-1.42378102115911,1.,1.25141455570299));
#28918=CARTESIAN_POINT('Ctrl Pts',(-1.41923722596421,-1.,1.24824430986911));
#28919=CARTESIAN_POINT('Ctrl Pts',(-1.41923722596421,1.,1.24824430986911));
#28920=CARTESIAN_POINT('Ctrl Pts',(-1.41422913175437,-1.,1.24450600513278));
#28921=CARTESIAN_POINT('Ctrl Pts',(-1.41422913175437,1.,1.24450600513278));
#28922=CARTESIAN_POINT('Ctrl Pts',(-1.40845295531151,-1.,1.23994455029421));
#28923=CARTESIAN_POINT('Ctrl Pts',(-1.40845295531151,1.,1.23994455029421));
#28924=CARTESIAN_POINT('Ctrl Pts',(-1.40164708205345,-1.,1.23434087289768));
#28925=CARTESIAN_POINT('Ctrl Pts',(-1.40164708205345,1.,1.23434087289768));
#28926=CARTESIAN_POINT('Ctrl Pts',(-1.39361389567257,-1.,1.22752961898063));
#28927=CARTESIAN_POINT('Ctrl Pts',(-1.39361389567257,1.,1.22752961898063));
#28928=CARTESIAN_POINT('Ctrl Pts',(-1.38420564525391,-1.,1.21938737278853));
#28929=CARTESIAN_POINT('Ctrl Pts',(-1.38420564525391,1.,1.21938737278853));
#28930=CARTESIAN_POINT('Ctrl Pts',(-1.37331915604962,-1.,1.20982812923113));
#28931=CARTESIAN_POINT('Ctrl Pts',(-1.37331915604962,1.,1.20982812923113));
#28932=CARTESIAN_POINT('Ctrl Pts',(-1.36088705040677,-1.,1.1987959077656));
#28933=CARTESIAN_POINT('Ctrl Pts',(-1.36088705040677,1.,1.1987959077656));
#28934=CARTESIAN_POINT('Ctrl Pts',(-1.34687053998157,-1.,1.18625865664915));
#28935=CARTESIAN_POINT('Ctrl Pts',(-1.34687053998157,1.,1.18625865664915));
#28936=CARTESIAN_POINT('Ctrl Pts',(-1.33437539344842,-1.,1.17501305787994));
#28937=CARTESIAN_POINT('Ctrl Pts',(-1.33437539344842,1.,1.17501305787994));
#28938=CARTESIAN_POINT('Ctrl Pts',(-1.32428080720544,-1.,1.16589330092532));
#28939=CARTESIAN_POINT('Ctrl Pts',(-1.32428080720544,1.,1.16589330092532));
#28940=CARTESIAN_POINT('Ctrl Pts',(-1.3172297721596,-1.,1.15950888730433));
#28941=CARTESIAN_POINT('Ctrl Pts',(-1.3172297721596,1.,1.15950888730433));
#28942=CARTESIAN_POINT('Ctrl Pts',(-1.31362392696033,-1.,1.15624053661742));
#28943=CARTESIAN_POINT('Ctrl Pts',(-1.31362392696033,1.,1.15624053661742));
#28944=CARTESIAN_POINT('',(-1.73811241238545,1.,1.34869019493419));
#28945=CARTESIAN_POINT('Ctrl Pts',(-1.73811241238545,1.,1.34869019493419));
#28946=CARTESIAN_POINT('Ctrl Pts',(-1.73682580585819,1.,1.34854391898145));
#28947=CARTESIAN_POINT('Ctrl Pts',(-1.73425417886255,1.,1.34824783113158));
#28948=CARTESIAN_POINT('Ctrl Pts',(-1.73040149654497,1.,1.3477930915247));
#28949=CARTESIAN_POINT('Ctrl Pts',(-1.72527410681298,1.,1.34716554820013));
#28950=CARTESIAN_POINT('Ctrl Pts',(-1.7188807715095,1.,1.34634568653586));
#28951=CARTESIAN_POINT('Ctrl Pts',(-1.71250340687011,1.,1.34549029589563));
#28952=CARTESIAN_POINT('Ctrl Pts',(-1.70614212266676,1.,1.34459924533783));
#28953=CARTESIAN_POINT('Ctrl Pts',(-1.69979707754221,1.,1.34367237124322));
#28954=CARTESIAN_POINT('Ctrl Pts',(-1.6934684849664,1.,1.34270948206139));
#28955=CARTESIAN_POINT('Ctrl Pts',(-1.68715660868602,1.,1.34171037484673));
#28956=CARTESIAN_POINT('Ctrl Pts',(-1.68086176030308,1.,1.3406748518516));
#28957=CARTESIAN_POINT('Ctrl Pts',(-1.67458429426126,1.,1.33960273470372));
#28958=CARTESIAN_POINT('Ctrl Pts',(-1.66832460784078,1.,1.33849388654458));
#28959=CARTESIAN_POINT('Ctrl Pts',(-1.66208312542073,1.,1.33734820885331));
#28960=CARTESIAN_POINT('Ctrl Pts',(-1.65586025952651,1.,1.33616559745217));
#28961=CARTESIAN_POINT('Ctrl Pts',(-1.64965637286843,1.,1.33494590468003));
#28962=CARTESIAN_POINT('Ctrl Pts',(-1.64347174856007,1.,1.33368890676554));
#28963=CARTESIAN_POINT('Ctrl Pts',(-1.6373065347505,1.,1.33239425103694));
#28964=CARTESIAN_POINT('Ctrl Pts',(-1.63116079730887,1.,1.33106149345618));
#28965=CARTESIAN_POINT('Ctrl Pts',(-1.62503464209777,1.,1.32969019505665));
#28966=CARTESIAN_POINT('Ctrl Pts',(-1.61892832270723,1.,1.32828000610448));
#28967=CARTESIAN_POINT('Ctrl Pts',(-1.61284234015762,1.,1.32683074483365));
#28968=CARTESIAN_POINT('Ctrl Pts',(-1.6067775829097,1.,1.32534250785794));
#28969=CARTESIAN_POINT('Ctrl Pts',(-1.600735118587,1.,1.32381550858266));
#28970=CARTESIAN_POINT('Ctrl Pts',(-1.59471591079408,1.,1.32224985747686));
#28971=CARTESIAN_POINT('Ctrl Pts',(-1.58872057258244,1.,1.32064537110891));
#28972=CARTESIAN_POINT('Ctrl Pts',(-1.58274907898829,1.,1.31900135021428));
#28973=CARTESIAN_POINT('Ctrl Pts',(-1.57680056505585,1.,1.31731642317183));
#28974=CARTESIAN_POINT('Ctrl Pts',(-1.57087397835721,1.,1.31558903860015));
#28975=CARTESIAN_POINT('Ctrl Pts',(-1.56496872402352,1.,1.31381795281002));
#28976=CARTESIAN_POINT('Ctrl Pts',(-1.55908521254822,1.,1.31200264341696));
#28977=CARTESIAN_POINT('Ctrl Pts',(-1.55322568759481,1.,1.31014393684221));
#28978=CARTESIAN_POINT('Ctrl Pts',(-1.54739413957183,1.,1.30824393907471));
#28979=CARTESIAN_POINT('Ctrl Pts',(-1.54159462645428,1.,1.30630475189553));
#28980=CARTESIAN_POINT('Ctrl Pts',(-1.53582981268976,1.,1.30432735639487));
#28981=CARTESIAN_POINT('Ctrl Pts',(-1.53009970283893,1.,1.3023106439557));
#28982=CARTESIAN_POINT('Ctrl Pts',(-1.5243995786107,1.,1.30024984366334));
#28983=CARTESIAN_POINT('Ctrl Pts',(-1.51872184912735,1.,1.29813791800757));
#28984=CARTESIAN_POINT('Ctrl Pts',(-1.51305994241412,1.,1.29596850710518));
#28985=CARTESIAN_POINT('Ctrl Pts',(-1.50741159078367,1.,1.29373841372843));
#28986=CARTESIAN_POINT('Ctrl Pts',(-1.50178230149764,1.,1.29145022885171));
#28987=CARTESIAN_POINT('Ctrl Pts',(-1.49618896881729,1.,1.28911506584232));
#28988=CARTESIAN_POINT('Ctrl Pts',(-1.4906522831275,1.,1.28674676116415));
#28989=CARTESIAN_POINT('Ctrl Pts',(-1.48518817118891,1.,1.28435533880184));
#28990=CARTESIAN_POINT('Ctrl Pts',(-1.47980070347102,1.,1.28194158939522));
#28991=CARTESIAN_POINT('Ctrl Pts',(-1.4744717526711,1.,1.27948918248524));
#28992=CARTESIAN_POINT('Ctrl Pts',(-1.46916035917197,1.,1.27696414831144));
#28993=CARTESIAN_POINT('Ctrl Pts',(-1.4638243133254,1.,1.27433119897877));
#28994=CARTESIAN_POINT('Ctrl Pts',(-1.45843906294725,1.,1.27156805265312));
#28995=CARTESIAN_POINT('Ctrl Pts',(-1.45301422764205,1.,1.26867786804854));
#28996=CARTESIAN_POINT('Ctrl Pts',(-1.44761985001544,1.,1.26570925118767));
#28997=CARTESIAN_POINT('Ctrl Pts',(-1.44236470511145,1.,1.26273903323723));
#28998=CARTESIAN_POINT('Ctrl Pts',(-1.43734919180719,1.,1.25983531011894));
#28999=CARTESIAN_POINT('Ctrl Pts',(-1.43262645609679,1.,1.25702687965744));
#29000=CARTESIAN_POINT('Ctrl Pts',(-1.42815938799555,1.,1.25426945222783));
#29001=CARTESIAN_POINT('Ctrl Pts',(-1.42378102115911,1.,1.25141455570299));
#29002=CARTESIAN_POINT('Ctrl Pts',(-1.41923722596421,1.,1.24824430986911));
#29003=CARTESIAN_POINT('Ctrl Pts',(-1.41422913175437,1.,1.24450600513278));
#29004=CARTESIAN_POINT('Ctrl Pts',(-1.40845295531151,1.,1.23994455029421));
#29005=CARTESIAN_POINT('Ctrl Pts',(-1.40164708205345,1.,1.23434087289768));
#29006=CARTESIAN_POINT('Ctrl Pts',(-1.39361389567257,1.,1.22752961898063));
#29007=CARTESIAN_POINT('Ctrl Pts',(-1.38420564525391,1.,1.21938737278853));
#29008=CARTESIAN_POINT('Ctrl Pts',(-1.37331915604962,1.,1.20982812923113));
#29009=CARTESIAN_POINT('Ctrl Pts',(-1.36088705040677,1.,1.1987959077656));
#29010=CARTESIAN_POINT('Ctrl Pts',(-1.34687053998157,1.,1.18625865664915));
#29011=CARTESIAN_POINT('Ctrl Pts',(-1.33437539344842,1.,1.17501305787994));
#29012=CARTESIAN_POINT('Ctrl Pts',(-1.32428080720544,1.,1.16589330092532));
#29013=CARTESIAN_POINT('Ctrl Pts',(-1.3172297721596,1.,1.15950888730433));
#29014=CARTESIAN_POINT('Ctrl Pts',(-1.31362392696033,1.,1.15624053661742));
#29015=CARTESIAN_POINT('',(-1.73811241238545,0.,1.34869019493419));
#29016=CARTESIAN_POINT('Origin',(-1.81978687191668,0.,1.23627494547115));
#29017=CARTESIAN_POINT('',(-1.81978687191668,1.,1.23627494547115));
#29018=CARTESIAN_POINT('',(-1.73811241238545,1.,1.34869019493419));
#29019=CARTESIAN_POINT('',(-1.81978687191668,0.,1.23627494547115));
#29020=CARTESIAN_POINT('Ctrl Pts',(-1.5055822144029,-1.,0.892032620296855));
#29021=CARTESIAN_POINT('Ctrl Pts',(-1.5055822144029,1.,0.892032620296855));
#29022=CARTESIAN_POINT('Ctrl Pts',(-1.50980486807181,-1.,0.894452006967538));
#29023=CARTESIAN_POINT('Ctrl Pts',(-1.50980486807181,1.,0.894452006967538));
#29024=CARTESIAN_POINT('Ctrl Pts',(-1.51805569591479,-1.,0.89918504749193));
#29025=CARTESIAN_POINT('Ctrl Pts',(-1.51805569591479,1.,0.89918504749193));
#29026=CARTESIAN_POINT('Ctrl Pts',(-1.52984849890434,-1.,0.905967409640499));
#29027=CARTESIAN_POINT('Ctrl Pts',(-1.52984849890434,1.,0.905967409640499));
#29028=CARTESIAN_POINT('Ctrl Pts',(-1.54440491152808,-1.,0.91437591904658));
#29029=CARTESIAN_POINT('Ctrl Pts',(-1.54440491152808,1.,0.91437591904658));
#29030=CARTESIAN_POINT('Ctrl Pts',(-1.56065988582509,-1.,0.923832188966322));
#29031=CARTESIAN_POINT('Ctrl Pts',(-1.56065988582509,1.,0.923832188966322));
#29032=CARTESIAN_POINT('Ctrl Pts',(-1.57499388385561,-1.,0.932246680128849));
#29033=CARTESIAN_POINT('Ctrl Pts',(-1.57499388385561,1.,0.932246680128849));
#29034=CARTESIAN_POINT('Ctrl Pts',(-1.58744937489796,-1.,0.939646377909319));
#29035=CARTESIAN_POINT('Ctrl Pts',(-1.58744937489796,1.,0.939646377909319));
#29036=CARTESIAN_POINT('Ctrl Pts',(-1.59810042045408,-1.,0.946078063325796));
#29037=CARTESIAN_POINT('Ctrl Pts',(-1.59810042045408,1.,0.946078063325796));
#29038=CARTESIAN_POINT('Ctrl Pts',(-1.60706069897794,-1.,0.951613284361248));
#29039=CARTESIAN_POINT('Ctrl Pts',(-1.60706069897794,1.,0.951613284361248));
#29040=CARTESIAN_POINT('Ctrl Pts',(-1.61449324337233,-1.,0.956354422921573));
#29041=CARTESIAN_POINT('Ctrl Pts',(-1.61449324337233,1.,0.956354422921573));
#29042=CARTESIAN_POINT('Ctrl Pts',(-1.62061638139929,-1.,0.960438326099958));
#29043=CARTESIAN_POINT('Ctrl Pts',(-1.62061638139929,1.,0.960438326099958));
#29044=CARTESIAN_POINT('Ctrl Pts',(-1.6257193066974,-1.,0.964046107037821));
#29045=CARTESIAN_POINT('Ctrl Pts',(-1.6257193066974,1.,0.964046107037821));
#29046=CARTESIAN_POINT('Ctrl Pts',(-1.63013849959083,-1.,0.967387853228041));
#29047=CARTESIAN_POINT('Ctrl Pts',(-1.63013849959083,1.,0.967387853228041));
#29048=CARTESIAN_POINT('Ctrl Pts',(-1.63420665729609,-1.,0.970669715996356));
#29049=CARTESIAN_POINT('Ctrl Pts',(-1.63420665729609,1.,0.970669715996356));
#29050=CARTESIAN_POINT('Ctrl Pts',(-1.63820952658157,-1.,0.974066058287501));
#29051=CARTESIAN_POINT('Ctrl Pts',(-1.63820952658157,1.,0.974066058287501));
#29052=CARTESIAN_POINT('Ctrl Pts',(-1.64233990826831,-1.,0.977689794120297));
#29053=CARTESIAN_POINT('Ctrl Pts',(-1.64233990826831,1.,0.977689794120297));
#29054=CARTESIAN_POINT('Ctrl Pts',(-1.64665139190834,-1.,0.981562530940574));
#29055=CARTESIAN_POINT('Ctrl Pts',(-1.64665139190834,1.,0.981562530940574));
#29056=CARTESIAN_POINT('Ctrl Pts',(-1.6511001661277,-1.,0.985642622921626));
#29057=CARTESIAN_POINT('Ctrl Pts',(-1.6511001661277,1.,0.985642622921626));
#29058=CARTESIAN_POINT('Ctrl Pts',(-1.65559044289746,-1.,0.98985562785445));
#29059=CARTESIAN_POINT('Ctrl Pts',(-1.65559044289746,1.,0.98985562785445));
#29060=CARTESIAN_POINT('Ctrl Pts',(-1.66001553809916,-1.,0.994121836661116));
#29061=CARTESIAN_POINT('Ctrl Pts',(-1.66001553809916,1.,0.994121836661116));
#29062=CARTESIAN_POINT('Ctrl Pts',(-1.66430758030304,-1.,0.998389654952317));
#29063=CARTESIAN_POINT('Ctrl Pts',(-1.66430758030304,1.,0.998389654952317));
#29064=CARTESIAN_POINT('Ctrl Pts',(-1.66846059277231,-1.,1.00265091003682));
#29065=CARTESIAN_POINT('Ctrl Pts',(-1.66846059277231,1.,1.00265091003682));
#29066=CARTESIAN_POINT('Ctrl Pts',(-1.67250335383248,-1.,1.00692206696387));
#29067=CARTESIAN_POINT('Ctrl Pts',(-1.67250335383248,1.,1.00692206696387));
#29068=CARTESIAN_POINT('Ctrl Pts',(-1.67648246776457,-1.,1.01123236493507));
#29069=CARTESIAN_POINT('Ctrl Pts',(-1.67648246776457,1.,1.01123236493507));
#29070=CARTESIAN_POINT('Ctrl Pts',(-1.6804428989482,-1.,1.01561026162787));
#29071=CARTESIAN_POINT('Ctrl Pts',(-1.6804428989482,1.,1.01561026162787));
#29072=CARTESIAN_POINT('Ctrl Pts',(-1.68440578021739,-1.,1.02006795074222));
#29073=CARTESIAN_POINT('Ctrl Pts',(-1.68440578021739,1.,1.02006795074222));
#29074=CARTESIAN_POINT('Ctrl Pts',(-1.68836910178475,-1.,1.02460180535272));
#29075=CARTESIAN_POINT('Ctrl Pts',(-1.68836910178475,1.,1.02460180535272));
#29076=CARTESIAN_POINT('Ctrl Pts',(-1.69231840863471,-1.,1.02919977579155));
#29077=CARTESIAN_POINT('Ctrl Pts',(-1.69231840863471,1.,1.02919977579155));
#29078=CARTESIAN_POINT('Ctrl Pts',(-1.69623414782769,-1.,1.03384646003587));
#29079=CARTESIAN_POINT('Ctrl Pts',(-1.69623414782769,1.,1.03384646003587));
#29080=CARTESIAN_POINT('Ctrl Pts',(-1.70010052930951,-1.,1.03852922490782));
#29081=CARTESIAN_POINT('Ctrl Pts',(-1.70010052930951,1.,1.03852922490782));
#29082=CARTESIAN_POINT('Ctrl Pts',(-1.70391338707969,-1.,1.04324363334546));
#29083=CARTESIAN_POINT('Ctrl Pts',(-1.70391338707969,1.,1.04324363334546));
#29084=CARTESIAN_POINT('Ctrl Pts',(-1.70767646263641,-1.,1.0479908540499));
#29085=CARTESIAN_POINT('Ctrl Pts',(-1.70767646263641,1.,1.0479908540499));
#29086=CARTESIAN_POINT('Ctrl Pts',(-1.71139783543986,-1.,1.05277517202854));
#29087=CARTESIAN_POINT('Ctrl Pts',(-1.71139783543986,1.,1.05277517202854));
#29088=CARTESIAN_POINT('Ctrl Pts',(-1.71508654427022,-1.,1.05760163192481));
#29089=CARTESIAN_POINT('Ctrl Pts',(-1.71508654427022,1.,1.05760163192481));
#29090=CARTESIAN_POINT('Ctrl Pts',(-1.71874858456908,-1.,1.0624732468065));
#29091=CARTESIAN_POINT('Ctrl Pts',(-1.71874858456908,1.,1.0624732468065));
#29092=CARTESIAN_POINT('Ctrl Pts',(-1.72238500928456,-1.,1.06738966975463));
#29093=CARTESIAN_POINT('Ctrl Pts',(-1.72238500928456,1.,1.06738966975463));
#29094=CARTESIAN_POINT('Ctrl Pts',(-1.72599406198489,-1.,1.07234866990252));
#29095=CARTESIAN_POINT('Ctrl Pts',(-1.72599406198489,1.,1.07234866990252));
#29096=CARTESIAN_POINT('Ctrl Pts',(-1.72957248977424,-1.,1.0773470373727));
#29097=CARTESIAN_POINT('Ctrl Pts',(-1.72957248977424,1.,1.0773470373727));
#29098=CARTESIAN_POINT('Ctrl Pts',(-1.73311705663407,-1.,1.08238162784749));
#29099=CARTESIAN_POINT('Ctrl Pts',(-1.73311705663407,1.,1.08238162784749));
#29100=CARTESIAN_POINT('Ctrl Pts',(-1.73662628326093,-1.,1.08745056285429));
#29101=CARTESIAN_POINT('Ctrl Pts',(-1.73662628326093,1.,1.08745056285429));
#29102=CARTESIAN_POINT('Ctrl Pts',(-1.74010053962252,-1.,1.09255329056496));
#29103=CARTESIAN_POINT('Ctrl Pts',(-1.74010053962252,1.,1.09255329056496));
#29104=CARTESIAN_POINT('Ctrl Pts',(-1.74354119236212,-1.,1.09768999241229));
#29105=CARTESIAN_POINT('Ctrl Pts',(-1.74354119236212,1.,1.09768999241229));
#29106=CARTESIAN_POINT('Ctrl Pts',(-1.74695004214924,-1.,1.10286118991144));
#29107=CARTESIAN_POINT('Ctrl Pts',(-1.74695004214924,1.,1.10286118991144));
#29108=CARTESIAN_POINT('Ctrl Pts',(-1.75032866075914,-1.,1.10806728183003));
#29109=CARTESIAN_POINT('Ctrl Pts',(-1.75032866075914,1.,1.10806728183003));
#29110=CARTESIAN_POINT('Ctrl Pts',(-1.75367772094617,-1.,1.11330807582542));
#29111=CARTESIAN_POINT('Ctrl Pts',(-1.75367772094617,1.,1.11330807582542));
#29112=CARTESIAN_POINT('Ctrl Pts',(-1.75699720772089,-1.,1.11858293216752));
#29113=CARTESIAN_POINT('Ctrl Pts',(-1.75699720772089,1.,1.11858293216752));
#29114=CARTESIAN_POINT('Ctrl Pts',(-1.76028671825084,-1.,1.12389096855078));
#29115=CARTESIAN_POINT('Ctrl Pts',(-1.76028671825084,1.,1.12389096855078));
#29116=CARTESIAN_POINT('Ctrl Pts',(-1.76354571966171,-1.,1.12923123555076));
#29117=CARTESIAN_POINT('Ctrl Pts',(-1.76354571966171,1.,1.12923123555076));
#29118=CARTESIAN_POINT('Ctrl Pts',(-1.76677384551883,-1.,1.13460291804635));
#29119=CARTESIAN_POINT('Ctrl Pts',(-1.76677384551883,1.,1.13460291804635));
#29120=CARTESIAN_POINT('Ctrl Pts',(-1.76997111386806,-1.,1.14000548337));
#29121=CARTESIAN_POINT('Ctrl Pts',(-1.76997111386806,1.,1.14000548337));
#29122=CARTESIAN_POINT('Ctrl Pts',(-1.77313777896234,-1.,1.14543858226948));
#29123=CARTESIAN_POINT('Ctrl Pts',(-1.77313777896234,1.,1.14543858226948));
#29124=CARTESIAN_POINT('Ctrl Pts',(-1.77627422557034,-1.,1.15090197841531));
#29125=CARTESIAN_POINT('Ctrl Pts',(-1.77627422557034,1.,1.15090197841531));
#29126=CARTESIAN_POINT('Ctrl Pts',(-1.77938085564261,-1.,1.15639547194689));
#29127=CARTESIAN_POINT('Ctrl Pts',(-1.77938085564261,1.,1.15639547194689));
#29128=CARTESIAN_POINT('Ctrl Pts',(-1.78245795880949,-1.,1.16191881298458));
#29129=CARTESIAN_POINT('Ctrl Pts',(-1.78245795880949,1.,1.16191881298458));
#29130=CARTESIAN_POINT('Ctrl Pts',(-1.78550566040349,-1.,1.16747166312239));
#29131=CARTESIAN_POINT('Ctrl Pts',(-1.78550566040349,1.,1.16747166312239));
#29132=CARTESIAN_POINT('Ctrl Pts',(-1.78852398877523,-1.,1.17305363177265));
#29133=CARTESIAN_POINT('Ctrl Pts',(-1.78852398877523,1.,1.17305363177265));
#29134=CARTESIAN_POINT('Ctrl Pts',(-1.79151291552646,-1.,1.17866429440781));
#29135=CARTESIAN_POINT('Ctrl Pts',(-1.79151291552646,1.,1.17866429440781));
#29136=CARTESIAN_POINT('Ctrl Pts',(-1.79447240321572,-1.,1.18430321697471));
#29137=CARTESIAN_POINT('Ctrl Pts',(-1.79447240321572,1.,1.18430321697471));
#29138=CARTESIAN_POINT('Ctrl Pts',(-1.79740245923649,-1.,1.1899699793456));
#29139=CARTESIAN_POINT('Ctrl Pts',(-1.79740245923649,1.,1.1899699793456));
#29140=CARTESIAN_POINT('Ctrl Pts',(-1.80030314370121,-1.,1.19566418930405));
#29141=CARTESIAN_POINT('Ctrl Pts',(-1.80030314370121,1.,1.19566418930405));
#29142=CARTESIAN_POINT('Ctrl Pts',(-1.8031745483882,-1.,1.2013854893912));
#29143=CARTESIAN_POINT('Ctrl Pts',(-1.8031745483882,1.,1.2013854893912));
#29144=CARTESIAN_POINT('Ctrl Pts',(-1.80601678480772,-1.,1.20713356605519));
#29145=CARTESIAN_POINT('Ctrl Pts',(-1.80601678480772,1.,1.20713356605519));
#29146=CARTESIAN_POINT('Ctrl Pts',(-1.80882996916931,-1.,1.2129081570818));
#29147=CARTESIAN_POINT('Ctrl Pts',(-1.80882996916931,1.,1.2129081570818));
#29148=CARTESIAN_POINT('Ctrl Pts',(-1.81161420806172,-1.,1.2187090610323));
#29149=CARTESIAN_POINT('Ctrl Pts',(-1.81161420806172,1.,1.2187090610323));
#29150=CARTESIAN_POINT('Ctrl Pts',(-1.81436959209778,-1.,1.22453613304507));
#29151=CARTESIAN_POINT('Ctrl Pts',(-1.81436959209778,1.,1.22453613304507));
#29152=CARTESIAN_POINT('Ctrl Pts',(-1.81655087183054,-1.,1.22921864890975));
#29153=CARTESIAN_POINT('Ctrl Pts',(-1.81655087183054,1.,1.22921864890975));
#29154=CARTESIAN_POINT('Ctrl Pts',(-1.81817389920914,-1.,1.23274224526804));
#29155=CARTESIAN_POINT('Ctrl Pts',(-1.81817389920914,1.,1.23274224526804));
#29156=CARTESIAN_POINT('Ctrl Pts',(-1.81925017193531,-1.,1.23509651170384));
#29157=CARTESIAN_POINT('Ctrl Pts',(-1.81925017193531,1.,1.23509651170384));
#29158=CARTESIAN_POINT('Ctrl Pts',(-1.81978687191668,-1.,1.23627494547115));
#29159=CARTESIAN_POINT('Ctrl Pts',(-1.81978687191668,1.,1.23627494547115));
#29160=CARTESIAN_POINT('',(-1.5055822144029,1.,0.892032620296855));
#29161=CARTESIAN_POINT('Ctrl Pts',(-1.5055822144029,1.,0.892032620296855));
#29162=CARTESIAN_POINT('Ctrl Pts',(-1.50980486807181,1.,0.894452006967538));
#29163=CARTESIAN_POINT('Ctrl Pts',(-1.51805569591479,1.,0.89918504749193));
#29164=CARTESIAN_POINT('Ctrl Pts',(-1.52984849890434,1.,0.905967409640499));
#29165=CARTESIAN_POINT('Ctrl Pts',(-1.54440491152808,1.,0.91437591904658));
#29166=CARTESIAN_POINT('Ctrl Pts',(-1.56065988582509,1.,0.923832188966322));
#29167=CARTESIAN_POINT('Ctrl Pts',(-1.57499388385561,1.,0.932246680128849));
#29168=CARTESIAN_POINT('Ctrl Pts',(-1.58744937489796,1.,0.939646377909319));
#29169=CARTESIAN_POINT('Ctrl Pts',(-1.59810042045408,1.,0.946078063325796));
#29170=CARTESIAN_POINT('Ctrl Pts',(-1.60706069897794,1.,0.951613284361248));
#29171=CARTESIAN_POINT('Ctrl Pts',(-1.61449324337233,1.,0.956354422921573));
#29172=CARTESIAN_POINT('Ctrl Pts',(-1.62061638139929,1.,0.960438326099958));
#29173=CARTESIAN_POINT('Ctrl Pts',(-1.6257193066974,1.,0.964046107037821));
#29174=CARTESIAN_POINT('Ctrl Pts',(-1.63013849959083,1.,0.967387853228041));
#29175=CARTESIAN_POINT('Ctrl Pts',(-1.63420665729609,1.,0.970669715996356));
#29176=CARTESIAN_POINT('Ctrl Pts',(-1.63820952658157,1.,0.974066058287501));
#29177=CARTESIAN_POINT('Ctrl Pts',(-1.64233990826831,1.,0.977689794120297));
#29178=CARTESIAN_POINT('Ctrl Pts',(-1.64665139190834,1.,0.981562530940574));
#29179=CARTESIAN_POINT('Ctrl Pts',(-1.6511001661277,1.,0.985642622921626));
#29180=CARTESIAN_POINT('Ctrl Pts',(-1.65559044289746,1.,0.98985562785445));
#29181=CARTESIAN_POINT('Ctrl Pts',(-1.66001553809916,1.,0.994121836661116));
#29182=CARTESIAN_POINT('Ctrl Pts',(-1.66430758030304,1.,0.998389654952317));
#29183=CARTESIAN_POINT('Ctrl Pts',(-1.66846059277231,1.,1.00265091003682));
#29184=CARTESIAN_POINT('Ctrl Pts',(-1.67250335383248,1.,1.00692206696387));
#29185=CARTESIAN_POINT('Ctrl Pts',(-1.67648246776457,1.,1.01123236493507));
#29186=CARTESIAN_POINT('Ctrl Pts',(-1.6804428989482,1.,1.01561026162787));
#29187=CARTESIAN_POINT('Ctrl Pts',(-1.68440578021739,1.,1.02006795074222));
#29188=CARTESIAN_POINT('Ctrl Pts',(-1.68836910178475,1.,1.02460180535272));
#29189=CARTESIAN_POINT('Ctrl Pts',(-1.69231840863471,1.,1.02919977579155));
#29190=CARTESIAN_POINT('Ctrl Pts',(-1.69623414782769,1.,1.03384646003587));
#29191=CARTESIAN_POINT('Ctrl Pts',(-1.70010052930951,1.,1.03852922490782));
#29192=CARTESIAN_POINT('Ctrl Pts',(-1.70391338707969,1.,1.04324363334546));
#29193=CARTESIAN_POINT('Ctrl Pts',(-1.70767646263641,1.,1.0479908540499));
#29194=CARTESIAN_POINT('Ctrl Pts',(-1.71139783543986,1.,1.05277517202854));
#29195=CARTESIAN_POINT('Ctrl Pts',(-1.71508654427022,1.,1.05760163192481));
#29196=CARTESIAN_POINT('Ctrl Pts',(-1.71874858456908,1.,1.0624732468065));
#29197=CARTESIAN_POINT('Ctrl Pts',(-1.72238500928456,1.,1.06738966975463));
#29198=CARTESIAN_POINT('Ctrl Pts',(-1.72599406198489,1.,1.07234866990252));
#29199=CARTESIAN_POINT('Ctrl Pts',(-1.72957248977424,1.,1.0773470373727));
#29200=CARTESIAN_POINT('Ctrl Pts',(-1.73311705663407,1.,1.08238162784749));
#29201=CARTESIAN_POINT('Ctrl Pts',(-1.73662628326093,1.,1.08745056285429));
#29202=CARTESIAN_POINT('Ctrl Pts',(-1.74010053962252,1.,1.09255329056496));
#29203=CARTESIAN_POINT('Ctrl Pts',(-1.74354119236212,1.,1.09768999241229));
#29204=CARTESIAN_POINT('Ctrl Pts',(-1.74695004214924,1.,1.10286118991144));
#29205=CARTESIAN_POINT('Ctrl Pts',(-1.75032866075914,1.,1.10806728183003));
#29206=CARTESIAN_POINT('Ctrl Pts',(-1.75367772094617,1.,1.11330807582542));
#29207=CARTESIAN_POINT('Ctrl Pts',(-1.75699720772089,1.,1.11858293216752));
#29208=CARTESIAN_POINT('Ctrl Pts',(-1.76028671825084,1.,1.12389096855078));
#29209=CARTESIAN_POINT('Ctrl Pts',(-1.76354571966171,1.,1.12923123555076));
#29210=CARTESIAN_POINT('Ctrl Pts',(-1.76677384551883,1.,1.13460291804635));
#29211=CARTESIAN_POINT('Ctrl Pts',(-1.76997111386806,1.,1.14000548337));
#29212=CARTESIAN_POINT('Ctrl Pts',(-1.77313777896234,1.,1.14543858226948));
#29213=CARTESIAN_POINT('Ctrl Pts',(-1.77627422557034,1.,1.15090197841531));
#29214=CARTESIAN_POINT('Ctrl Pts',(-1.77938085564261,1.,1.15639547194689));
#29215=CARTESIAN_POINT('Ctrl Pts',(-1.78245795880949,1.,1.16191881298458));
#29216=CARTESIAN_POINT('Ctrl Pts',(-1.78550566040349,1.,1.16747166312239));
#29217=CARTESIAN_POINT('Ctrl Pts',(-1.78852398877523,1.,1.17305363177265));
#29218=CARTESIAN_POINT('Ctrl Pts',(-1.79151291552646,1.,1.17866429440781));
#29219=CARTESIAN_POINT('Ctrl Pts',(-1.79447240321572,1.,1.18430321697471));
#29220=CARTESIAN_POINT('Ctrl Pts',(-1.79740245923649,1.,1.1899699793456));
#29221=CARTESIAN_POINT('Ctrl Pts',(-1.80030314370121,1.,1.19566418930405));
#29222=CARTESIAN_POINT('Ctrl Pts',(-1.8031745483882,1.,1.2013854893912));
#29223=CARTESIAN_POINT('Ctrl Pts',(-1.80601678480772,1.,1.20713356605519));
#29224=CARTESIAN_POINT('Ctrl Pts',(-1.80882996916931,1.,1.2129081570818));
#29225=CARTESIAN_POINT('Ctrl Pts',(-1.81161420806172,1.,1.2187090610323));
#29226=CARTESIAN_POINT('Ctrl Pts',(-1.81436959209778,1.,1.22453613304507));
#29227=CARTESIAN_POINT('Ctrl Pts',(-1.81655087183054,1.,1.22921864890975));
#29228=CARTESIAN_POINT('Ctrl Pts',(-1.81817389920914,1.,1.23274224526804));
#29229=CARTESIAN_POINT('Ctrl Pts',(-1.81925017193531,1.,1.23509651170384));
#29230=CARTESIAN_POINT('Ctrl Pts',(-1.81978687191668,1.,1.23627494547115));
#29231=CARTESIAN_POINT('',(-1.5055822144029,0.,0.892032620296856));
#29232=CARTESIAN_POINT('Origin',(0.,0.,0.));
#29233=CARTESIAN_POINT('',(-1.60662857109684,1.,0.693717979106305));
#29234=CARTESIAN_POINT('Origin',(0.,1.,0.));
#29235=CARTESIAN_POINT('',(-1.60662857109684,0.,0.693717979106306));
#29236=CARTESIAN_POINT('Ctrl Pts',(-2.0698113262342,-1.,0.7455743247944));
#29237=CARTESIAN_POINT('Ctrl Pts',(-2.0698113262342,1.,0.7455743247944));
#29238=CARTESIAN_POINT('Ctrl Pts',(-2.06854248895728,-1.,0.745832791378367));
#29239=CARTESIAN_POINT('Ctrl Pts',(-2.06854248895728,1.,0.745832791378367));
#29240=CARTESIAN_POINT('Ctrl Pts',(-2.06600523016815,-1.,0.7463458715442));
#29241=CARTESIAN_POINT('Ctrl Pts',(-2.06600523016815,1.,0.7463458715442));
#29242=CARTESIAN_POINT('Ctrl Pts',(-2.06220058927826,-1.,0.747103932787919));
#29243=CARTESIAN_POINT('Ctrl Pts',(-2.06220058927826,1.,0.747103932787919));
#29244=CARTESIAN_POINT('Ctrl Pts',(-2.05713023031006,-1.,0.748091554183802));
#29245=CARTESIAN_POINT('Ctrl Pts',(-2.05713023031006,1.,0.748091554183802));
#29246=CARTESIAN_POINT('Ctrl Pts',(-2.05079645592154,-1.,0.749287468665046));
#29247=CARTESIAN_POINT('Ctrl Pts',(-2.05079645592154,1.,0.749287468665046));
#29248=CARTESIAN_POINT('Ctrl Pts',(-2.04446689147979,-1.,0.750444657875576));
#29249=CARTESIAN_POINT('Ctrl Pts',(-2.04446689147979,1.,0.750444657875576));
#29250=CARTESIAN_POINT('Ctrl Pts',(-2.03814160092099,-1.,0.751562963361115));
#29251=CARTESIAN_POINT('Ctrl Pts',(-2.03814160092099,1.,0.751562963361115));
#29252=CARTESIAN_POINT('Ctrl Pts',(-2.03182068456221,-1.,0.752642180487211));
#29253=CARTESIAN_POINT('Ctrl Pts',(-2.03182068456221,1.,0.752642180487211));
#29254=CARTESIAN_POINT('Ctrl Pts',(-2.02550428623313,-1.,0.753682061112768));
#29255=CARTESIAN_POINT('Ctrl Pts',(-2.02550428623313,1.,0.753682061112768));
#29256=CARTESIAN_POINT('Ctrl Pts',(-2.01919259405809,-1.,0.754682330722816));
#29257=CARTESIAN_POINT('Ctrl Pts',(-2.01919259405809,1.,0.754682330722816));
#29258=CARTESIAN_POINT('Ctrl Pts',(-2.01288584328084,-1.,0.755642704957865));
#29259=CARTESIAN_POINT('Ctrl Pts',(-2.01288584328084,1.,0.755642704957865));
#29260=CARTESIAN_POINT('Ctrl Pts',(-2.0065843158773,-1.,0.75656290464667));
#29261=CARTESIAN_POINT('Ctrl Pts',(-2.0065843158773,1.,0.75656290464667));
#29262=CARTESIAN_POINT('Ctrl Pts',(-2.00028834739178,-1.,0.757442676862724));
#29263=CARTESIAN_POINT('Ctrl Pts',(-2.00028834739178,1.,0.757442676862724));
#29264=CARTESIAN_POINT('Ctrl Pts',(-1.99399831098817,-1.,0.758281796766761));
#29265=CARTESIAN_POINT('Ctrl Pts',(-1.99399831098817,1.,0.758281796766761));
#29266=CARTESIAN_POINT('Ctrl Pts',(-1.98771456680874,-1.,0.759080037802488));
#29267=CARTESIAN_POINT('Ctrl Pts',(-1.98771456680874,1.,0.759080037802488));
#29268=CARTESIAN_POINT('Ctrl Pts',(-1.98143741418172,-1.,0.75983714745219));
#29269=CARTESIAN_POINT('Ctrl Pts',(-1.98143741418172,1.,0.75983714745219));
#29270=CARTESIAN_POINT('Ctrl Pts',(-1.97516705321494,-1.,0.760552825409757));
#29271=CARTESIAN_POINT('Ctrl Pts',(-1.97516705321494,1.,0.760552825409757));
#29272=CARTESIAN_POINT('Ctrl Pts',(-1.96890351582499,-1.,0.76122669048382));
#29273=CARTESIAN_POINT('Ctrl Pts',(-1.96890351582499,1.,0.76122669048382));
#29274=CARTESIAN_POINT('Ctrl Pts',(-1.96264672744186,-1.,0.761858300014423));
#29275=CARTESIAN_POINT('Ctrl Pts',(-1.96264672744186,1.,0.761858300014423));
#29276=CARTESIAN_POINT('Ctrl Pts',(-1.95639665309869,-1.,0.762447203806179));
#29277=CARTESIAN_POINT('Ctrl Pts',(-1.95639665309869,1.,0.762447203806179));
#29278=CARTESIAN_POINT('Ctrl Pts',(-1.95015342590024,-1.,0.762992990878769));
#29279=CARTESIAN_POINT('Ctrl Pts',(-1.95015342590024,1.,0.762992990878769));
#29280=CARTESIAN_POINT('Ctrl Pts',(-1.9439174661764,-1.,0.763495333538629));
#29281=CARTESIAN_POINT('Ctrl Pts',(-1.9439174661764,1.,0.763495333538629));
#29282=CARTESIAN_POINT('Ctrl Pts',(-1.93768964875886,-1.,0.763954049121458));
#29283=CARTESIAN_POINT('Ctrl Pts',(-1.93768964875886,1.,0.763954049121458));
#29284=CARTESIAN_POINT('Ctrl Pts',(-1.93147105496382,-1.,0.76436901067394));
#29285=CARTESIAN_POINT('Ctrl Pts',(-1.93147105496382,1.,0.76436901067394));
#29286=CARTESIAN_POINT('Ctrl Pts',(-1.92526263537048,-1.,0.764740025488211));
#29287=CARTESIAN_POINT('Ctrl Pts',(-1.92526263537048,1.,0.764740025488211));
#29288=CARTESIAN_POINT('Ctrl Pts',(-1.91906491634196,-1.,0.765066729667088));
#29289=CARTESIAN_POINT('Ctrl Pts',(-1.91906491634196,1.,0.765066729667088));
#29290=CARTESIAN_POINT('Ctrl Pts',(-1.91287765805169,-1.,0.765348465884722));
#29291=CARTESIAN_POINT('Ctrl Pts',(-1.91287765805169,1.,0.765348465884722));
#29292=CARTESIAN_POINT('Ctrl Pts',(-1.90669961402356,-1.,0.765584196937919));
#29293=CARTESIAN_POINT('Ctrl Pts',(-1.90669961402356,1.,0.765584196937919));
#29294=CARTESIAN_POINT('Ctrl Pts',(-1.90052930393596,-1.,0.765772772593386));
#29295=CARTESIAN_POINT('Ctrl Pts',(-1.90052930393596,1.,0.765772772593386));
#29296=CARTESIAN_POINT('Ctrl Pts',(-1.89436577771388,-1.,0.765913193856978));
#29297=CARTESIAN_POINT('Ctrl Pts',(-1.89436577771388,1.,0.765913193856978));
#29298=CARTESIAN_POINT('Ctrl Pts',(-1.88820926433409,-1.,0.766004837062091));
#29299=CARTESIAN_POINT('Ctrl Pts',(-1.88820926433409,1.,0.766004837062091));
#29300=CARTESIAN_POINT('Ctrl Pts',(-1.88206215302561,-1.,0.766047794851864));
#29301=CARTESIAN_POINT('Ctrl Pts',(-1.88206215302561,1.,0.766047794851864));
#29302=CARTESIAN_POINT('Ctrl Pts',(-1.87592888967883,-1.,0.766042837036744));
#29303=CARTESIAN_POINT('Ctrl Pts',(-1.87592888967883,1.,0.766042837036744));
#29304=CARTESIAN_POINT('Ctrl Pts',(-1.86981398314341,-1.,0.765990708546091));
#29305=CARTESIAN_POINT('Ctrl Pts',(-1.86981398314341,1.,0.765990708546091));
#29306=CARTESIAN_POINT('Ctrl Pts',(-1.86372027063312,-1.,0.765891519092547));
#29307=CARTESIAN_POINT('Ctrl Pts',(-1.86372027063312,1.,0.765891519092547));
#29308=CARTESIAN_POINT('Ctrl Pts',(-1.85764741390394,-1.,0.765744212909318));
#29309=CARTESIAN_POINT('Ctrl Pts',(-1.85764741390394,1.,0.765744212909318));
#29310=CARTESIAN_POINT('Ctrl Pts',(-1.85158945130063,-1.,0.765545710619062));
#29311=CARTESIAN_POINT('Ctrl Pts',(-1.85158945130063,1.,0.765545710619062));
#29312=CARTESIAN_POINT('Ctrl Pts',(-1.84553698875924,-1.,0.765291664862029));
#29313=CARTESIAN_POINT('Ctrl Pts',(-1.84553698875924,1.,0.765291664862029));
#29314=CARTESIAN_POINT('Ctrl Pts',(-1.83948181064835,-1.,0.764978057881737));
#29315=CARTESIAN_POINT('Ctrl Pts',(-1.83948181064835,1.,0.764978057881737));
#29316=CARTESIAN_POINT('Ctrl Pts',(-1.83342077227142,-1.,0.764602549687853));
#29317=CARTESIAN_POINT('Ctrl Pts',(-1.83342077227142,1.,0.764602549687853));
#29318=CARTESIAN_POINT('Ctrl Pts',(-1.82735991200065,-1.,0.764165902605995));
#29319=CARTESIAN_POINT('Ctrl Pts',(-1.82735991200065,1.,0.764165902605995));
#29320=CARTESIAN_POINT('Ctrl Pts',(-1.82131873145266,-1.,0.763673465462726));
#29321=CARTESIAN_POINT('Ctrl Pts',(-1.82131873145266,1.,0.763673465462726));
#29322=CARTESIAN_POINT('Ctrl Pts',(-1.8153211840553,-1.,0.763132003836634));
#29323=CARTESIAN_POINT('Ctrl Pts',(-1.8153211840553,1.,0.763132003836634));
#29324=CARTESIAN_POINT('Ctrl Pts',(-1.80938551463965,-1.,0.762546129463938));
#29325=CARTESIAN_POINT('Ctrl Pts',(-1.80938551463965,1.,0.762546129463938));
#29326=CARTESIAN_POINT('Ctrl Pts',(-1.80351583877342,-1.,0.761915336443547));
#29327=CARTESIAN_POINT('Ctrl Pts',(-1.80351583877342,1.,0.761915336443547));
#29328=CARTESIAN_POINT('Ctrl Pts',(-1.79768986997783,-1.,0.761229695230558));
#29329=CARTESIAN_POINT('Ctrl Pts',(-1.79768986997783,1.,0.761229695230558));
#29330=CARTESIAN_POINT('Ctrl Pts',(-1.7918581561088,-1.,0.760469555880749));
#29331=CARTESIAN_POINT('Ctrl Pts',(-1.7918581561088,1.,0.760469555880749));
#29332=CARTESIAN_POINT('Ctrl Pts',(-1.78596964884604,-1.,0.759614401110189));
#29333=CARTESIAN_POINT('Ctrl Pts',(-1.78596964884604,1.,0.759614401110189));
#29334=CARTESIAN_POINT('Ctrl Pts',(-1.77999411220945,-1.,0.758650626677518));
#29335=CARTESIAN_POINT('Ctrl Pts',(-1.77999411220945,1.,0.758650626677518));
#29336=CARTESIAN_POINT('Ctrl Pts',(-1.77394167108292,-1.,0.757578264077029));
#29337=CARTESIAN_POINT('Ctrl Pts',(-1.77394167108292,1.,0.757578264077029));
#29338=CARTESIAN_POINT('Ctrl Pts',(-1.76789396002998,-1.,0.75642189602781));
#29339=CARTESIAN_POINT('Ctrl Pts',(-1.76789396002998,1.,0.75642189602781));
#29340=CARTESIAN_POINT('Ctrl Pts',(-1.76197817240128,-1.,0.755220979974461));
#29341=CARTESIAN_POINT('Ctrl Pts',(-1.76197817240128,1.,0.755220979974461));
#29342=CARTESIAN_POINT('Ctrl Pts',(-1.75631083600019,-1.,0.754009254027829));
#29343=CARTESIAN_POINT('Ctrl Pts',(-1.75631083600019,1.,0.754009254027829));
#29344=CARTESIAN_POINT('Ctrl Pts',(-1.75095139468794,-1.,0.752797683531314));
#29345=CARTESIAN_POINT('Ctrl Pts',(-1.75095139468794,1.,0.752797683531314));
#29346=CARTESIAN_POINT('Ctrl Pts',(-1.74585086852502,-1.,0.751555614164482));
#29347=CARTESIAN_POINT('Ctrl Pts',(-1.74585086852502,1.,0.751555614164482));
#29348=CARTESIAN_POINT('Ctrl Pts',(-1.74080458267114,-1.,0.750193435981249));
#29349=CARTESIAN_POINT('Ctrl Pts',(-1.74080458267114,1.,0.750193435981249));
#29350=CARTESIAN_POINT('Ctrl Pts',(-1.7355035168033,-1.,0.74858246295687));
#29351=CARTESIAN_POINT('Ctrl Pts',(-1.7355035168033,1.,0.74858246295687));
#29352=CARTESIAN_POINT('Ctrl Pts',(-1.72958533647714,-1.,0.746574710097752));
#29353=CARTESIAN_POINT('Ctrl Pts',(-1.72958533647714,1.,0.746574710097752));
#29354=CARTESIAN_POINT('Ctrl Pts',(-1.72268229916769,-1.,0.744021445433093));
#29355=CARTESIAN_POINT('Ctrl Pts',(-1.72268229916769,1.,0.744021445433093));
#29356=CARTESIAN_POINT('Ctrl Pts',(-1.71447789751001,-1.,0.74079516202821));
#29357=CARTESIAN_POINT('Ctrl Pts',(-1.71447789751001,1.,0.74079516202821));
#29358=CARTESIAN_POINT('Ctrl Pts',(-1.70473309004249,-1.,0.736799665716932));
#29359=CARTESIAN_POINT('Ctrl Pts',(-1.70473309004249,1.,0.736799665716932));
#29360=CARTESIAN_POINT('Ctrl Pts',(-1.69326921972915,-1.,0.731963238685357));
#29361=CARTESIAN_POINT('Ctrl Pts',(-1.69326921972915,1.,0.731963238685357));
#29362=CARTESIAN_POINT('Ctrl Pts',(-1.67996158451922,-1.,0.726235967982445));
#29363=CARTESIAN_POINT('Ctrl Pts',(-1.67996158451922,1.,0.726235967982445));
#29364=CARTESIAN_POINT('Ctrl Pts',(-1.66472880551777,-1.,0.71958543378795));
#29365=CARTESIAN_POINT('Ctrl Pts',(-1.66472880551777,1.,0.71958543378795));
#29366=CARTESIAN_POINT('Ctrl Pts',(-1.64752408828442,-1.,0.711993139340447));
#29367=CARTESIAN_POINT('Ctrl Pts',(-1.64752408828442,1.,0.711993139340447));
#29368=CARTESIAN_POINT('Ctrl Pts',(-1.6321654166204,-1.,0.705159151977294));
#29369=CARTESIAN_POINT('Ctrl Pts',(-1.6321654166204,1.,0.705159151977294));
#29370=CARTESIAN_POINT('Ctrl Pts',(-1.61974673471117,-1.,0.699605146398837));
#29371=CARTESIAN_POINT('Ctrl Pts',(-1.61974673471117,1.,0.699605146398837));
#29372=CARTESIAN_POINT('Ctrl Pts',(-1.61106790957619,-1.,0.69571209787897));
#29373=CARTESIAN_POINT('Ctrl Pts',(-1.61106790957619,1.,0.69571209787897));
#29374=CARTESIAN_POINT('Ctrl Pts',(-1.60662857109684,-1.,0.693717979106305));
#29375=CARTESIAN_POINT('Ctrl Pts',(-1.60662857109684,1.,0.693717979106305));
#29376=CARTESIAN_POINT('',(-2.0698113262342,1.,0.7455743247944));
#29377=CARTESIAN_POINT('Ctrl Pts',(-2.0698113262342,1.,0.7455743247944));
#29378=CARTESIAN_POINT('Ctrl Pts',(-2.06854248895728,1.,0.745832791378367));
#29379=CARTESIAN_POINT('Ctrl Pts',(-2.06600523016815,1.,0.7463458715442));
#29380=CARTESIAN_POINT('Ctrl Pts',(-2.06220058927826,1.,0.747103932787919));
#29381=CARTESIAN_POINT('Ctrl Pts',(-2.05713023031006,1.,0.748091554183802));
#29382=CARTESIAN_POINT('Ctrl Pts',(-2.05079645592154,1.,0.749287468665046));
#29383=CARTESIAN_POINT('Ctrl Pts',(-2.04446689147979,1.,0.750444657875576));
#29384=CARTESIAN_POINT('Ctrl Pts',(-2.03814160092099,1.,0.751562963361115));
#29385=CARTESIAN_POINT('Ctrl Pts',(-2.03182068456221,1.,0.752642180487211));
#29386=CARTESIAN_POINT('Ctrl Pts',(-2.02550428623313,1.,0.753682061112768));
#29387=CARTESIAN_POINT('Ctrl Pts',(-2.01919259405809,1.,0.754682330722816));
#29388=CARTESIAN_POINT('Ctrl Pts',(-2.01288584328084,1.,0.755642704957865));
#29389=CARTESIAN_POINT('Ctrl Pts',(-2.0065843158773,1.,0.75656290464667));
#29390=CARTESIAN_POINT('Ctrl Pts',(-2.00028834739178,1.,0.757442676862724));
#29391=CARTESIAN_POINT('Ctrl Pts',(-1.99399831098817,1.,0.758281796766761));
#29392=CARTESIAN_POINT('Ctrl Pts',(-1.98771456680874,1.,0.759080037802488));
#29393=CARTESIAN_POINT('Ctrl Pts',(-1.98143741418172,1.,0.75983714745219));
#29394=CARTESIAN_POINT('Ctrl Pts',(-1.97516705321494,1.,0.760552825409757));
#29395=CARTESIAN_POINT('Ctrl Pts',(-1.96890351582499,1.,0.76122669048382));
#29396=CARTESIAN_POINT('Ctrl Pts',(-1.96264672744186,1.,0.761858300014423));
#29397=CARTESIAN_POINT('Ctrl Pts',(-1.95639665309869,1.,0.762447203806179));
#29398=CARTESIAN_POINT('Ctrl Pts',(-1.95015342590024,1.,0.762992990878769));
#29399=CARTESIAN_POINT('Ctrl Pts',(-1.9439174661764,1.,0.763495333538629));
#29400=CARTESIAN_POINT('Ctrl Pts',(-1.93768964875886,1.,0.763954049121458));
#29401=CARTESIAN_POINT('Ctrl Pts',(-1.93147105496382,1.,0.76436901067394));
#29402=CARTESIAN_POINT('Ctrl Pts',(-1.92526263537048,1.,0.764740025488211));
#29403=CARTESIAN_POINT('Ctrl Pts',(-1.91906491634196,1.,0.765066729667088));
#29404=CARTESIAN_POINT('Ctrl Pts',(-1.91287765805169,1.,0.765348465884722));
#29405=CARTESIAN_POINT('Ctrl Pts',(-1.90669961402356,1.,0.765584196937919));
#29406=CARTESIAN_POINT('Ctrl Pts',(-1.90052930393596,1.,0.765772772593386));
#29407=CARTESIAN_POINT('Ctrl Pts',(-1.89436577771388,1.,0.765913193856978));
#29408=CARTESIAN_POINT('Ctrl Pts',(-1.88820926433409,1.,0.766004837062091));
#29409=CARTESIAN_POINT('Ctrl Pts',(-1.88206215302561,1.,0.766047794851864));
#29410=CARTESIAN_POINT('Ctrl Pts',(-1.87592888967883,1.,0.766042837036744));
#29411=CARTESIAN_POINT('Ctrl Pts',(-1.86981398314341,1.,0.765990708546091));
#29412=CARTESIAN_POINT('Ctrl Pts',(-1.86372027063312,1.,0.765891519092547));
#29413=CARTESIAN_POINT('Ctrl Pts',(-1.85764741390394,1.,0.765744212909318));
#29414=CARTESIAN_POINT('Ctrl Pts',(-1.85158945130063,1.,0.765545710619062));
#29415=CARTESIAN_POINT('Ctrl Pts',(-1.84553698875924,1.,0.765291664862029));
#29416=CARTESIAN_POINT('Ctrl Pts',(-1.83948181064835,1.,0.764978057881737));
#29417=CARTESIAN_POINT('Ctrl Pts',(-1.83342077227142,1.,0.764602549687853));
#29418=CARTESIAN_POINT('Ctrl Pts',(-1.82735991200065,1.,0.764165902605995));
#29419=CARTESIAN_POINT('Ctrl Pts',(-1.82131873145266,1.,0.763673465462726));
#29420=CARTESIAN_POINT('Ctrl Pts',(-1.8153211840553,1.,0.763132003836634));
#29421=CARTESIAN_POINT('Ctrl Pts',(-1.80938551463965,1.,0.762546129463938));
#29422=CARTESIAN_POINT('Ctrl Pts',(-1.80351583877342,1.,0.761915336443547));
#29423=CARTESIAN_POINT('Ctrl Pts',(-1.79768986997783,1.,0.761229695230558));
#29424=CARTESIAN_POINT('Ctrl Pts',(-1.7918581561088,1.,0.760469555880749));
#29425=CARTESIAN_POINT('Ctrl Pts',(-1.78596964884604,1.,0.759614401110189));
#29426=CARTESIAN_POINT('Ctrl Pts',(-1.77999411220945,1.,0.758650626677518));
#29427=CARTESIAN_POINT('Ctrl Pts',(-1.77394167108292,1.,0.757578264077029));
#29428=CARTESIAN_POINT('Ctrl Pts',(-1.76789396002998,1.,0.75642189602781));
#29429=CARTESIAN_POINT('Ctrl Pts',(-1.76197817240128,1.,0.755220979974461));
#29430=CARTESIAN_POINT('Ctrl Pts',(-1.75631083600019,1.,0.754009254027829));
#29431=CARTESIAN_POINT('Ctrl Pts',(-1.75095139468794,1.,0.752797683531314));
#29432=CARTESIAN_POINT('Ctrl Pts',(-1.74585086852502,1.,0.751555614164482));
#29433=CARTESIAN_POINT('Ctrl Pts',(-1.74080458267114,1.,0.750193435981249));
#29434=CARTESIAN_POINT('Ctrl Pts',(-1.7355035168033,1.,0.74858246295687));
#29435=CARTESIAN_POINT('Ctrl Pts',(-1.72958533647714,1.,0.746574710097752));
#29436=CARTESIAN_POINT('Ctrl Pts',(-1.72268229916769,1.,0.744021445433093));
#29437=CARTESIAN_POINT('Ctrl Pts',(-1.71447789751001,1.,0.74079516202821));
#29438=CARTESIAN_POINT('Ctrl Pts',(-1.70473309004249,1.,0.736799665716932));
#29439=CARTESIAN_POINT('Ctrl Pts',(-1.69326921972915,1.,0.731963238685357));
#29440=CARTESIAN_POINT('Ctrl Pts',(-1.67996158451922,1.,0.726235967982445));
#29441=CARTESIAN_POINT('Ctrl Pts',(-1.66472880551777,1.,0.71958543378795));
#29442=CARTESIAN_POINT('Ctrl Pts',(-1.64752408828442,1.,0.711993139340447));
#29443=CARTESIAN_POINT('Ctrl Pts',(-1.6321654166204,1.,0.705159151977294));
#29444=CARTESIAN_POINT('Ctrl Pts',(-1.61974673471117,1.,0.699605146398837));
#29445=CARTESIAN_POINT('Ctrl Pts',(-1.61106790957619,1.,0.69571209787897));
#29446=CARTESIAN_POINT('Ctrl Pts',(-1.60662857109684,1.,0.693717979106305));
#29447=CARTESIAN_POINT('',(-2.0698113262342,0.,0.7455743247944));
#29448=CARTESIAN_POINT('Origin',(-2.11275013067528,0.,0.61342227326009));
#29449=CARTESIAN_POINT('',(-2.11275013067528,1.,0.61342227326009));
#29450=CARTESIAN_POINT('',(-2.0698113262342,1.,0.7455743247944));
#29451=CARTESIAN_POINT('',(-2.11275013067528,0.,0.61342227326009));
#29452=CARTESIAN_POINT('Ctrl Pts',(-1.7075470150345,-1.,0.383122945602004));
#29453=CARTESIAN_POINT('Ctrl Pts',(-1.7075470150345,1.,0.383122945602004));
#29454=CARTESIAN_POINT('Ctrl Pts',(-1.71231062891958,-1.,0.384119047315542));
#29455=CARTESIAN_POINT('Ctrl Pts',(-1.71231062891958,1.,0.384119047315542));
#29456=CARTESIAN_POINT('Ctrl Pts',(-1.72162022246158,-1.,0.38607079032701));
#29457=CARTESIAN_POINT('Ctrl Pts',(-1.72162022246158,1.,0.38607079032701));
#29458=CARTESIAN_POINT('Ctrl Pts',(-1.7349317097561,-1.,0.388877023509191));
#29459=CARTESIAN_POINT('Ctrl Pts',(-1.7349317097561,1.,0.388877023509191));
#29460=CARTESIAN_POINT('Ctrl Pts',(-1.75137405313962,-1.,0.392375812294307));
#29461=CARTESIAN_POINT('Ctrl Pts',(-1.75137405313962,1.,0.392375812294307));
#29462=CARTESIAN_POINT('Ctrl Pts',(-1.7697556004756,-1.,0.39634619612042));
#29463=CARTESIAN_POINT('Ctrl Pts',(-1.7697556004756,1.,0.39634619612042));
#29464=CARTESIAN_POINT('Ctrl Pts',(-1.78598826347533,-1.,0.39991940378308));
#29465=CARTESIAN_POINT('Ctrl Pts',(-1.78598826347533,1.,0.39991940378308));
#29466=CARTESIAN_POINT('Ctrl Pts',(-1.80012077176221,-1.,0.403107976170441));
#29467=CARTESIAN_POINT('Ctrl Pts',(-1.80012077176221,1.,0.403107976170441));
#29468=CARTESIAN_POINT('Ctrl Pts',(-1.81223801813988,-1.,0.405933518411838));
#29469=CARTESIAN_POINT('Ctrl Pts',(-1.81223801813988,1.,0.405933518411838));
#29470=CARTESIAN_POINT('Ctrl Pts',(-1.8224702267854,-1.,0.408428948108533));
#29471=CARTESIAN_POINT('Ctrl Pts',(-1.8224702267854,1.,0.408428948108533));
#29472=CARTESIAN_POINT('Ctrl Pts',(-1.83100408895216,-1.,0.410641256301675));
#29473=CARTESIAN_POINT('Ctrl Pts',(-1.83100408895216,1.,0.410641256301675));
#29474=CARTESIAN_POINT('Ctrl Pts',(-1.83808953475839,-1.,0.412633125322161));
#29475=CARTESIAN_POINT('Ctrl Pts',(-1.83808953475839,1.,0.412633125322161));
#29476=CARTESIAN_POINT('Ctrl Pts',(-1.8440575707371,-1.,0.41448743825434));
#29477=CARTESIAN_POINT('Ctrl Pts',(-1.8440575707371,1.,0.41448743825434));
#29478=CARTESIAN_POINT('Ctrl Pts',(-1.84929312929882,-1.,0.416300022038864));
#29479=CARTESIAN_POINT('Ctrl Pts',(-1.84929312929882,1.,0.416300022038864));
#29480=CARTESIAN_POINT('Ctrl Pts',(-1.85417632856234,-1.,0.418164129143534));
#29481=CARTESIAN_POINT('Ctrl Pts',(-1.85417632856234,1.,0.418164129143534));
#29482=CARTESIAN_POINT('Ctrl Pts',(-1.85903281096686,-1.,0.420157287975619));
#29483=CARTESIAN_POINT('Ctrl Pts',(-1.85903281096686,1.,0.420157287975619));
#29484=CARTESIAN_POINT('Ctrl Pts',(-1.86408083334028,-1.,0.422327307418275));
#29485=CARTESIAN_POINT('Ctrl Pts',(-1.86408083334028,1.,0.422327307418275));
#29486=CARTESIAN_POINT('Ctrl Pts',(-1.86937803944323,-1.,0.424678177291359));
#29487=CARTESIAN_POINT('Ctrl Pts',(-1.86937803944323,1.,0.424678177291359));
#29488=CARTESIAN_POINT('Ctrl Pts',(-1.87486989291484,-1.,0.427183828519102));
#29489=CARTESIAN_POINT('Ctrl Pts',(-1.87486989291484,1.,0.427183828519102));
#29490=CARTESIAN_POINT('Ctrl Pts',(-1.88044229001832,-1.,0.429803062482344));
#29491=CARTESIAN_POINT('Ctrl Pts',(-1.88044229001832,1.,0.429803062482344));
#29492=CARTESIAN_POINT('Ctrl Pts',(-1.88596913666793,-1.,0.432493038548748));
#29493=CARTESIAN_POINT('Ctrl Pts',(-1.88596913666793,1.,0.432493038548748));
#29494=CARTESIAN_POINT('Ctrl Pts',(-1.89136993975504,-1.,0.435225660963383));
#29495=CARTESIAN_POINT('Ctrl Pts',(-1.89136993975504,1.,0.435225660963383));
#29496=CARTESIAN_POINT('Ctrl Pts',(-1.89663648956466,-1.,0.437995003948244));
#29497=CARTESIAN_POINT('Ctrl Pts',(-1.89663648956466,1.,0.437995003948244));
#29498=CARTESIAN_POINT('Ctrl Pts',(-1.90180124389086,-1.,0.440807833704038));
#29499=CARTESIAN_POINT('Ctrl Pts',(-1.90180124389086,1.,0.440807833704038));
#29500=CARTESIAN_POINT('Ctrl Pts',(-1.90691756144898,-1.,0.44367755684915));
#29501=CARTESIAN_POINT('Ctrl Pts',(-1.90691756144898,1.,0.44367755684915));
#29502=CARTESIAN_POINT('Ctrl Pts',(-1.9120369998112,-1.,0.446617343485711));
#29503=CARTESIAN_POINT('Ctrl Pts',(-1.9120369998112,1.,0.446617343485711));
#29504=CARTESIAN_POINT('Ctrl Pts',(-1.91718342555755,-1.,0.449632260106662));
#29505=CARTESIAN_POINT('Ctrl Pts',(-1.91718342555755,1.,0.449632260106662));
#29506=CARTESIAN_POINT('Ctrl Pts',(-1.92235380648502,-1.,0.452719478359432));
#29507=CARTESIAN_POINT('Ctrl Pts',(-1.92235380648502,1.,0.452719478359432));
#29508=CARTESIAN_POINT('Ctrl Pts',(-1.92753067150476,-1.,0.455872005174371));
#29509=CARTESIAN_POINT('Ctrl Pts',(-1.92753067150476,1.,0.455872005174371));
#29510=CARTESIAN_POINT('Ctrl Pts',(-1.93269066517934,-1.,0.459081234547926));
#29511=CARTESIAN_POINT('Ctrl Pts',(-1.93269066517934,1.,0.459081234547926));
#29512=CARTESIAN_POINT('Ctrl Pts',(-1.93781486640821,-1.,0.462340031009056));
#29513=CARTESIAN_POINT('Ctrl Pts',(-1.93781486640821,1.,0.462340031009056));
#29514=CARTESIAN_POINT('Ctrl Pts',(-1.9428979419619,-1.,0.46564546202603));
#29515=CARTESIAN_POINT('Ctrl Pts',(-1.9428979419619,1.,0.46564546202603));
#29516=CARTESIAN_POINT('Ctrl Pts',(-1.94794381136514,-1.,0.468997482913135));
#29517=CARTESIAN_POINT('Ctrl Pts',(-1.94794381136514,1.,0.468997482913135));
#29518=CARTESIAN_POINT('Ctrl Pts',(-1.95296148278133,-1.,0.472397672264072));
#29519=CARTESIAN_POINT('Ctrl Pts',(-1.95296148278133,1.,0.472397672264072));
#29520=CARTESIAN_POINT('Ctrl Pts',(-1.95796111148177,-1.,0.475848034683176));
#29521=CARTESIAN_POINT('Ctrl Pts',(-1.95796111148177,1.,0.475848034683176));
#29522=CARTESIAN_POINT('Ctrl Pts',(-1.96294933055943,-1.,0.479349583074855));
#29523=CARTESIAN_POINT('Ctrl Pts',(-1.96294933055943,1.,0.479349583074855));
#29524=CARTESIAN_POINT('Ctrl Pts',(-1.96792703422362,-1.,0.48290166212069));
#29525=CARTESIAN_POINT('Ctrl Pts',(-1.96792703422362,1.,0.48290166212069));
#29526=CARTESIAN_POINT('Ctrl Pts',(-1.97289186263272,-1.,0.486502692907659));
#29527=CARTESIAN_POINT('Ctrl Pts',(-1.97289186263272,1.,0.486502692907659));
#29528=CARTESIAN_POINT('Ctrl Pts',(-1.97783973019229,-1.,0.490150627860952));
#29529=CARTESIAN_POINT('Ctrl Pts',(-1.97783973019229,1.,0.490150627860952));
#29530=CARTESIAN_POINT('Ctrl Pts',(-1.98276658761821,-1.,0.493843476541494));
#29531=CARTESIAN_POINT('Ctrl Pts',(-1.98276658761821,1.,0.493843476541494));
#29532=CARTESIAN_POINT('Ctrl Pts',(-1.98767044752932,-1.,0.497579909545574));
#29533=CARTESIAN_POINT('Ctrl Pts',(-1.98767044752932,1.,0.497579909545574));
#29534=CARTESIAN_POINT('Ctrl Pts',(-1.99255149126155,-1.,0.501359287727146));
#29535=CARTESIAN_POINT('Ctrl Pts',(-1.99255149126155,1.,0.501359287727146));
#29536=CARTESIAN_POINT('Ctrl Pts',(-1.99741107463572,-1.,0.505181361323026));
#29537=CARTESIAN_POINT('Ctrl Pts',(-1.99741107463572,1.,0.505181361323026));
#29538=CARTESIAN_POINT('Ctrl Pts',(-2.00225107134734,-1.,0.509046069886157));
#29539=CARTESIAN_POINT('Ctrl Pts',(-2.00225107134734,1.,0.509046069886157));
#29540=CARTESIAN_POINT('Ctrl Pts',(-2.00707309946949,-1.,0.512953306961792));
#29541=CARTESIAN_POINT('Ctrl Pts',(-2.00707309946949,1.,0.512953306961792));
#29542=CARTESIAN_POINT('Ctrl Pts',(-2.01187773939242,-1.,0.516902681728687));
#29543=CARTESIAN_POINT('Ctrl Pts',(-2.01187773939242,1.,0.516902681728687));
#29544=CARTESIAN_POINT('Ctrl Pts',(-2.01666477917286,-1.,0.52089359039937));
#29545=CARTESIAN_POINT('Ctrl Pts',(-2.01666477917286,1.,0.52089359039937));
#29546=CARTESIAN_POINT('Ctrl Pts',(-2.02143356304698,-1.,0.524925318333476));
#29547=CARTESIAN_POINT('Ctrl Pts',(-2.02143356304698,1.,0.524925318333476));
#29548=CARTESIAN_POINT('Ctrl Pts',(-2.0261832908329,-1.,0.528997127241914));
#29549=CARTESIAN_POINT('Ctrl Pts',(-2.0261832908329,1.,0.528997127241914));
#29550=CARTESIAN_POINT('Ctrl Pts',(-2.03091336214426,-1.,0.533108355132976));
#29551=CARTESIAN_POINT('Ctrl Pts',(-2.03091336214426,1.,0.533108355132976));
#29552=CARTESIAN_POINT('Ctrl Pts',(-2.03562362954037,-1.,0.537258489833262));
#29553=CARTESIAN_POINT('Ctrl Pts',(-2.03562362954037,1.,0.537258489833262));
#29554=CARTESIAN_POINT('Ctrl Pts',(-2.04031422690527,-1.,0.541447120615659));
#29555=CARTESIAN_POINT('Ctrl Pts',(-2.04031422690527,1.,0.541447120615659));
#29556=CARTESIAN_POINT('Ctrl Pts',(-2.04498544714588,-1.,0.54567390381743));
#29557=CARTESIAN_POINT('Ctrl Pts',(-2.04498544714588,1.,0.54567390381743));
#29558=CARTESIAN_POINT('Ctrl Pts',(-2.04963761077958,-1.,0.549938525150295));
#29559=CARTESIAN_POINT('Ctrl Pts',(-2.04963761077958,1.,0.549938525150295));
#29560=CARTESIAN_POINT('Ctrl Pts',(-2.05427091604413,-1.,0.554240657463906));
#29561=CARTESIAN_POINT('Ctrl Pts',(-2.05427091604413,1.,0.554240657463906));
#29562=CARTESIAN_POINT('Ctrl Pts',(-2.05888537756462,-1.,0.558579940185151));
#29563=CARTESIAN_POINT('Ctrl Pts',(-2.05888537756462,1.,0.558579940185151));
#29564=CARTESIAN_POINT('Ctrl Pts',(-2.06348090160589,-1.,0.562955993082261));
#29565=CARTESIAN_POINT('Ctrl Pts',(-2.06348090160589,1.,0.562955993082261));
#29566=CARTESIAN_POINT('Ctrl Pts',(-2.06805732997334,-1.,0.567368421181087));
#29567=CARTESIAN_POINT('Ctrl Pts',(-2.06805732997334,1.,0.567368421181087));
#29568=CARTESIAN_POINT('Ctrl Pts',(-2.07261449292824,-1.,0.571816823242603));
#29569=CARTESIAN_POINT('Ctrl Pts',(-2.07261449292824,1.,0.571816823242603));
#29570=CARTESIAN_POINT('Ctrl Pts',(-2.07715226767559,-1.,0.576300797416844));
#29571=CARTESIAN_POINT('Ctrl Pts',(-2.07715226767559,1.,0.576300797416844));
#29572=CARTESIAN_POINT('Ctrl Pts',(-2.08167059018418,-1.,0.580819952108063));
#29573=CARTESIAN_POINT('Ctrl Pts',(-2.08167059018418,1.,0.580819952108063));
#29574=CARTESIAN_POINT('Ctrl Pts',(-2.08616943727951,-1.,0.585373918991617));
#29575=CARTESIAN_POINT('Ctrl Pts',(-2.08616943727951,1.,0.585373918991617));
#29576=CARTESIAN_POINT('Ctrl Pts',(-2.09064881812129,-1.,0.589962365403406));
#29577=CARTESIAN_POINT('Ctrl Pts',(-2.09064881812129,1.,0.589962365403406));
#29578=CARTESIAN_POINT('Ctrl Pts',(-2.0951087622027,-1.,0.594585006052162));
#29579=CARTESIAN_POINT('Ctrl Pts',(-2.0951087622027,1.,0.594585006052162));
#29580=CARTESIAN_POINT('Ctrl Pts',(-2.0995493086477,-1.,0.599241616420533));
#29581=CARTESIAN_POINT('Ctrl Pts',(-2.0995493086477,1.,0.599241616420533));
#29582=CARTESIAN_POINT('Ctrl Pts',(-2.10397049886949,-1.,0.60393203073603));
#29583=CARTESIAN_POINT('Ctrl Pts',(-2.10397049886949,1.,0.60393203073603));
#29584=CARTESIAN_POINT('Ctrl Pts',(-2.1074919961518,-1.,0.607711315454876));
#29585=CARTESIAN_POINT('Ctrl Pts',(-2.1074919961518,1.,0.607711315454876));
#29586=CARTESIAN_POINT('Ctrl Pts',(-2.11012443807238,-1.,0.610560911689899));
#29587=CARTESIAN_POINT('Ctrl Pts',(-2.11012443807238,1.,0.610560911689899));
#29588=CARTESIAN_POINT('Ctrl Pts',(-2.11187554259986,-1.,0.6124673655618));
#29589=CARTESIAN_POINT('Ctrl Pts',(-2.11187554259986,1.,0.6124673655618));
#29590=CARTESIAN_POINT('Ctrl Pts',(-2.11275013067528,-1.,0.61342227326009));
#29591=CARTESIAN_POINT('Ctrl Pts',(-2.11275013067528,1.,0.61342227326009));
#29592=CARTESIAN_POINT('',(-1.7075470150345,1.,0.383122945602004));
#29593=CARTESIAN_POINT('Ctrl Pts',(-1.7075470150345,1.,0.383122945602004));
#29594=CARTESIAN_POINT('Ctrl Pts',(-1.71231062891958,1.,0.384119047315542));
#29595=CARTESIAN_POINT('Ctrl Pts',(-1.72162022246158,1.,0.38607079032701));
#29596=CARTESIAN_POINT('Ctrl Pts',(-1.7349317097561,1.,0.388877023509191));
#29597=CARTESIAN_POINT('Ctrl Pts',(-1.75137405313962,1.,0.392375812294307));
#29598=CARTESIAN_POINT('Ctrl Pts',(-1.7697556004756,1.,0.39634619612042));
#29599=CARTESIAN_POINT('Ctrl Pts',(-1.78598826347533,1.,0.39991940378308));
#29600=CARTESIAN_POINT('Ctrl Pts',(-1.80012077176221,1.,0.403107976170441));
#29601=CARTESIAN_POINT('Ctrl Pts',(-1.81223801813988,1.,0.405933518411838));
#29602=CARTESIAN_POINT('Ctrl Pts',(-1.8224702267854,1.,0.408428948108533));
#29603=CARTESIAN_POINT('Ctrl Pts',(-1.83100408895216,1.,0.410641256301675));
#29604=CARTESIAN_POINT('Ctrl Pts',(-1.83808953475839,1.,0.412633125322161));
#29605=CARTESIAN_POINT('Ctrl Pts',(-1.8440575707371,1.,0.41448743825434));
#29606=CARTESIAN_POINT('Ctrl Pts',(-1.84929312929882,1.,0.416300022038864));
#29607=CARTESIAN_POINT('Ctrl Pts',(-1.85417632856234,1.,0.418164129143534));
#29608=CARTESIAN_POINT('Ctrl Pts',(-1.85903281096686,1.,0.420157287975619));
#29609=CARTESIAN_POINT('Ctrl Pts',(-1.86408083334028,1.,0.422327307418275));
#29610=CARTESIAN_POINT('Ctrl Pts',(-1.86937803944323,1.,0.424678177291359));
#29611=CARTESIAN_POINT('Ctrl Pts',(-1.87486989291484,1.,0.427183828519102));
#29612=CARTESIAN_POINT('Ctrl Pts',(-1.88044229001832,1.,0.429803062482344));
#29613=CARTESIAN_POINT('Ctrl Pts',(-1.88596913666793,1.,0.432493038548748));
#29614=CARTESIAN_POINT('Ctrl Pts',(-1.89136993975504,1.,0.435225660963383));
#29615=CARTESIAN_POINT('Ctrl Pts',(-1.89663648956466,1.,0.437995003948244));
#29616=CARTESIAN_POINT('Ctrl Pts',(-1.90180124389086,1.,0.440807833704038));
#29617=CARTESIAN_POINT('Ctrl Pts',(-1.90691756144898,1.,0.44367755684915));
#29618=CARTESIAN_POINT('Ctrl Pts',(-1.9120369998112,1.,0.446617343485711));
#29619=CARTESIAN_POINT('Ctrl Pts',(-1.91718342555755,1.,0.449632260106662));
#29620=CARTESIAN_POINT('Ctrl Pts',(-1.92235380648502,1.,0.452719478359432));
#29621=CARTESIAN_POINT('Ctrl Pts',(-1.92753067150476,1.,0.455872005174371));
#29622=CARTESIAN_POINT('Ctrl Pts',(-1.93269066517934,1.,0.459081234547926));
#29623=CARTESIAN_POINT('Ctrl Pts',(-1.93781486640821,1.,0.462340031009056));
#29624=CARTESIAN_POINT('Ctrl Pts',(-1.9428979419619,1.,0.46564546202603));
#29625=CARTESIAN_POINT('Ctrl Pts',(-1.94794381136514,1.,0.468997482913135));
#29626=CARTESIAN_POINT('Ctrl Pts',(-1.95296148278133,1.,0.472397672264072));
#29627=CARTESIAN_POINT('Ctrl Pts',(-1.95796111148177,1.,0.475848034683176));
#29628=CARTESIAN_POINT('Ctrl Pts',(-1.96294933055943,1.,0.479349583074855));
#29629=CARTESIAN_POINT('Ctrl Pts',(-1.96792703422362,1.,0.48290166212069));
#29630=CARTESIAN_POINT('Ctrl Pts',(-1.97289186263272,1.,0.486502692907659));
#29631=CARTESIAN_POINT('Ctrl Pts',(-1.97783973019229,1.,0.490150627860952));
#29632=CARTESIAN_POINT('Ctrl Pts',(-1.98276658761821,1.,0.493843476541494));
#29633=CARTESIAN_POINT('Ctrl Pts',(-1.98767044752932,1.,0.497579909545574));
#29634=CARTESIAN_POINT('Ctrl Pts',(-1.99255149126155,1.,0.501359287727146));
#29635=CARTESIAN_POINT('Ctrl Pts',(-1.99741107463572,1.,0.505181361323026));
#29636=CARTESIAN_POINT('Ctrl Pts',(-2.00225107134734,1.,0.509046069886157));
#29637=CARTESIAN_POINT('Ctrl Pts',(-2.00707309946949,1.,0.512953306961792));
#29638=CARTESIAN_POINT('Ctrl Pts',(-2.01187773939242,1.,0.516902681728687));
#29639=CARTESIAN_POINT('Ctrl Pts',(-2.01666477917286,1.,0.52089359039937));
#29640=CARTESIAN_POINT('Ctrl Pts',(-2.02143356304698,1.,0.524925318333476));
#29641=CARTESIAN_POINT('Ctrl Pts',(-2.0261832908329,1.,0.528997127241914));
#29642=CARTESIAN_POINT('Ctrl Pts',(-2.03091336214426,1.,0.533108355132976));
#29643=CARTESIAN_POINT('Ctrl Pts',(-2.03562362954037,1.,0.537258489833262));
#29644=CARTESIAN_POINT('Ctrl Pts',(-2.04031422690527,1.,0.541447120615659));
#29645=CARTESIAN_POINT('Ctrl Pts',(-2.04498544714588,1.,0.54567390381743));
#29646=CARTESIAN_POINT('Ctrl Pts',(-2.04963761077958,1.,0.549938525150295));
#29647=CARTESIAN_POINT('Ctrl Pts',(-2.05427091604413,1.,0.554240657463906));
#29648=CARTESIAN_POINT('Ctrl Pts',(-2.05888537756462,1.,0.558579940185151));
#29649=CARTESIAN_POINT('Ctrl Pts',(-2.06348090160589,1.,0.562955993082261));
#29650=CARTESIAN_POINT('Ctrl Pts',(-2.06805732997334,1.,0.567368421181087));
#29651=CARTESIAN_POINT('Ctrl Pts',(-2.07261449292824,1.,0.571816823242603));
#29652=CARTESIAN_POINT('Ctrl Pts',(-2.07715226767559,1.,0.576300797416844));
#29653=CARTESIAN_POINT('Ctrl Pts',(-2.08167059018418,1.,0.580819952108063));
#29654=CARTESIAN_POINT('Ctrl Pts',(-2.08616943727951,1.,0.585373918991617));
#29655=CARTESIAN_POINT('Ctrl Pts',(-2.09064881812129,1.,0.589962365403406));
#29656=CARTESIAN_POINT('Ctrl Pts',(-2.0951087622027,1.,0.594585006052162));
#29657=CARTESIAN_POINT('Ctrl Pts',(-2.0995493086477,1.,0.599241616420533));
#29658=CARTESIAN_POINT('Ctrl Pts',(-2.10397049886949,1.,0.60393203073603));
#29659=CARTESIAN_POINT('Ctrl Pts',(-2.1074919961518,1.,0.607711315454876));
#29660=CARTESIAN_POINT('Ctrl Pts',(-2.11012443807238,1.,0.610560911689899));
#29661=CARTESIAN_POINT('Ctrl Pts',(-2.11187554259986,1.,0.6124673655618));
#29662=CARTESIAN_POINT('Ctrl Pts',(-2.11275013067528,1.,0.61342227326009));
#29663=CARTESIAN_POINT('',(-1.7075470150345,0.,0.383122945602003));
#29664=CARTESIAN_POINT('Origin',(0.,0.,0.));
#29665=CARTESIAN_POINT('',(-1.74236521665491,1.,0.163289472382896));
#29666=CARTESIAN_POINT('Origin',(0.,1.,0.));
#29667=CARTESIAN_POINT('',(-1.74236521665491,0.,0.163289472382896));
#29668=CARTESIAN_POINT('Ctrl Pts',(-2.19890268624765,-1.,0.069476445021958));
#29669=CARTESIAN_POINT('Ctrl Pts',(-2.19890268624765,1.,0.069476445021958));
#29670=CARTESIAN_POINT('Ctrl Pts',(-2.19777582085423,-1.,0.0701143536325489));
#29671=CARTESIAN_POINT('Ctrl Pts',(-2.19777582085423,1.,0.0701143536325489));
#29672=CARTESIAN_POINT('Ctrl Pts',(-2.19552129484002,-1.,0.0713863779526153));
#29673=CARTESIAN_POINT('Ctrl Pts',(-2.19552129484002,1.,0.0713863779526153));
#29674=CARTESIAN_POINT('Ctrl Pts',(-2.19213712013662,-1.,0.0732830357306724));
#29675=CARTESIAN_POINT('Ctrl Pts',(-2.19213712013662,1.,0.0732830357306724));
#29676=CARTESIAN_POINT('Ctrl Pts',(-2.1876201139953,-1.,0.0757891465836146));
#29677=CARTESIAN_POINT('Ctrl Pts',(-2.1876201139953,1.,0.0757891465836146));
#29678=CARTESIAN_POINT('Ctrl Pts',(-2.18196589448887,-1.,0.0788837727685241));
#29679=CARTESIAN_POINT('Ctrl Pts',(-2.18196589448887,1.,0.0788837727685241));
#29680=CARTESIAN_POINT('Ctrl Pts',(-2.176303712113,-1.,0.0819402680872764));
#29681=CARTESIAN_POINT('Ctrl Pts',(-2.176303712113,1.,0.0819402680872764));
#29682=CARTESIAN_POINT('Ctrl Pts',(-2.17063357870952,-1.,0.0849584620835371));
#29683=CARTESIAN_POINT('Ctrl Pts',(-2.17063357870952,1.,0.0849584620835371));
#29684=CARTESIAN_POINT('Ctrl Pts',(-2.16495552645014,-1.,0.0879381291386921));
#29685=CARTESIAN_POINT('Ctrl Pts',(-2.16495552645014,1.,0.0879381291386921));
#29686=CARTESIAN_POINT('Ctrl Pts',(-2.15926961544516,-1.,0.0908789888107264));
#29687=CARTESIAN_POINT('Ctrl Pts',(-2.15926961544516,1.,0.0908789888107264));
#29688=CARTESIAN_POINT('Ctrl Pts',(-2.1535759397817,-1.,0.0937807218867642));
#29689=CARTESIAN_POINT('Ctrl Pts',(-2.1535759397817,1.,0.0937807218867642));
#29690=CARTESIAN_POINT('Ctrl Pts',(-2.14787463531795,-1.,0.0966429852305457));
#29691=CARTESIAN_POINT('Ctrl Pts',(-2.14787463531795,1.,0.0966429852305457));
#29692=CARTESIAN_POINT('Ctrl Pts',(-2.14216588396025,-1.,0.0994654261990914));
#29693=CARTESIAN_POINT('Ctrl Pts',(-2.14216588396025,1.,0.0994654261990914));
#29694=CARTESIAN_POINT('Ctrl Pts',(-2.13644992667165,-1.,0.1022477005561));
#29695=CARTESIAN_POINT('Ctrl Pts',(-2.13644992667165,1.,0.1022477005561));
#29696=CARTESIAN_POINT('Ctrl Pts',(-2.13072704887293,-1.,0.104989479152739));
#29697=CARTESIAN_POINT('Ctrl Pts',(-2.13072704887293,1.,0.104989479152739));
#29698=CARTESIAN_POINT('Ctrl Pts',(-2.12499752307,-1.,0.10769043523109));
#29699=CARTESIAN_POINT('Ctrl Pts',(-2.12499752307,1.,0.10769043523109));
#29700=CARTESIAN_POINT('Ctrl Pts',(-2.11926155590865,-1.,0.110350236135025));
#29701=CARTESIAN_POINT('Ctrl Pts',(-2.11926155590865,1.,0.110350236135025));
#29702=CARTESIAN_POINT('Ctrl Pts',(-2.11351924490306,-1.,0.112968534419737));
#29703=CARTESIAN_POINT('Ctrl Pts',(-2.11351924490306,1.,0.112968534419737));
#29704=CARTESIAN_POINT('Ctrl Pts',(-2.10777050261309,-1.,0.115544957687926));
#29705=CARTESIAN_POINT('Ctrl Pts',(-2.10777050261309,1.,0.115544957687926));
#29706=CARTESIAN_POINT('Ctrl Pts',(-2.102015121329,-1.,0.118079107988355));
#29707=CARTESIAN_POINT('Ctrl Pts',(-2.102015121329,1.,0.118079107988355));
#29708=CARTESIAN_POINT('Ctrl Pts',(-2.0962529286773,-1.,0.120570567965122));
#29709=CARTESIAN_POINT('Ctrl Pts',(-2.0962529286773,1.,0.120570567965122));
#29710=CARTESIAN_POINT('Ctrl Pts',(-2.09048392424825,-1.,0.123018905621083));
#29711=CARTESIAN_POINT('Ctrl Pts',(-2.09048392424825,1.,0.123018905621083));
#29712=CARTESIAN_POINT('Ctrl Pts',(-2.08470840653643,-1.,0.125423679412061));
#29713=CARTESIAN_POINT('Ctrl Pts',(-2.08470840653643,1.,0.125423679412061));
#29714=CARTESIAN_POINT('Ctrl Pts',(-2.07892715110987,-1.,0.12778444527612));
#29715=CARTESIAN_POINT('Ctrl Pts',(-2.07892715110987,1.,0.12778444527612));
#29716=CARTESIAN_POINT('Ctrl Pts',(-2.07314114713063,-1.,0.130100748328403));
#29717=CARTESIAN_POINT('Ctrl Pts',(-2.07314114713063,1.,0.130100748328403));
#29718=CARTESIAN_POINT('Ctrl Pts',(-2.06735123910326,-1.,0.13237211154771));
#29719=CARTESIAN_POINT('Ctrl Pts',(-2.06735123910326,1.,0.13237211154771));
#29720=CARTESIAN_POINT('Ctrl Pts',(-2.06155781517842,-1.,0.134598026192106));
#29721=CARTESIAN_POINT('Ctrl Pts',(-2.06155781517842,1.,0.134598026192106));
#29722=CARTESIAN_POINT('Ctrl Pts',(-2.05576044414264,-1.,0.136777941218043));
#29723=CARTESIAN_POINT('Ctrl Pts',(-2.05576044414264,1.,0.136777941218043));
#29724=CARTESIAN_POINT('Ctrl Pts',(-2.04995762001328,-1.,0.138911255368966));
#29725=CARTESIAN_POINT('Ctrl Pts',(-2.04995762001328,1.,0.138911255368966));
#29726=CARTESIAN_POINT('Ctrl Pts',(-2.04414757947916,-1.,0.140997332152546));
#29727=CARTESIAN_POINT('Ctrl Pts',(-2.04414757947916,1.,0.140997332152546));
#29728=CARTESIAN_POINT('Ctrl Pts',(-2.03832911025912,-1.,0.143035515058209));
#29729=CARTESIAN_POINT('Ctrl Pts',(-2.03832911025912,1.,0.143035515058209));
#29730=CARTESIAN_POINT('Ctrl Pts',(-2.03250223739942,-1.,0.145025140186057));
#29731=CARTESIAN_POINT('Ctrl Pts',(-2.03250223739942,1.,0.145025140186057));
#29732=CARTESIAN_POINT('Ctrl Pts',(-2.02666926182017,-1.,0.146965557332583));
#29733=CARTESIAN_POINT('Ctrl Pts',(-2.02666926182017,1.,0.146965557332583));
#29734=CARTESIAN_POINT('Ctrl Pts',(-2.02083464969894,-1.,0.148856124775337));
#29735=CARTESIAN_POINT('Ctrl Pts',(-2.02083464969894,1.,0.148856124775337));
#29736=CARTESIAN_POINT('Ctrl Pts',(-2.01500291940238,-1.,0.150696157673078));
#29737=CARTESIAN_POINT('Ctrl Pts',(-2.01500291940238,1.,0.150696157673078));
#29738=CARTESIAN_POINT('Ctrl Pts',(-2.00917680318424,-1.,0.15248488362145));
#29739=CARTESIAN_POINT('Ctrl Pts',(-2.00917680318424,1.,0.15248488362145));
#29740=CARTESIAN_POINT('Ctrl Pts',(-2.00335565310543,-1.,0.154221403049722));
#29741=CARTESIAN_POINT('Ctrl Pts',(-2.00335565310543,1.,0.154221403049722));
#29742=CARTESIAN_POINT('Ctrl Pts',(-1.99753284771497,-1.,0.155904629548783));
#29743=CARTESIAN_POINT('Ctrl Pts',(-1.99753284771497,1.,0.155904629548783));
#29744=CARTESIAN_POINT('Ctrl Pts',(-1.99169810931908,-1.,0.157533331459227));
#29745=CARTESIAN_POINT('Ctrl Pts',(-1.99169810931908,1.,0.157533331459227));
#29746=CARTESIAN_POINT('Ctrl Pts',(-1.98584238283292,-1.,0.159106226437299));
#29747=CARTESIAN_POINT('Ctrl Pts',(-1.98584238283292,1.,0.159106226437299));
#29748=CARTESIAN_POINT('Ctrl Pts',(-1.97996195437559,-1.,0.160622060784611));
#29749=CARTESIAN_POINT('Ctrl Pts',(-1.97996195437559,1.,0.160622060784611));
#29750=CARTESIAN_POINT('Ctrl Pts',(-1.97406280235188,-1.,0.162079693556288));
#29751=CARTESIAN_POINT('Ctrl Pts',(-1.97406280235188,1.,0.162079693556288));
#29752=CARTESIAN_POINT('Ctrl Pts',(-1.96816512677967,-1.,0.163478185457734));
#29753=CARTESIAN_POINT('Ctrl Pts',(-1.96816512677967,1.,0.163478185457734));
#29754=CARTESIAN_POINT('Ctrl Pts',(-1.96229379940136,-1.,0.164816568920269));
#29755=CARTESIAN_POINT('Ctrl Pts',(-1.96229379940136,1.,0.164816568920269));
#29756=CARTESIAN_POINT('Ctrl Pts',(-1.9564675971873,-1.,0.166093592002812));
#29757=CARTESIAN_POINT('Ctrl Pts',(-1.9564675971873,1.,0.166093592002812));
#29758=CARTESIAN_POINT('Ctrl Pts',(-1.95069027794294,-1.,0.167307501784475));
#29759=CARTESIAN_POINT('Ctrl Pts',(-1.95069027794294,1.,0.167307501784475));
#29760=CARTESIAN_POINT('Ctrl Pts',(-1.94493757756931,-1.,0.168455741607556));
#29761=CARTESIAN_POINT('Ctrl Pts',(-1.94493757756931,1.,0.168455741607556));
#29762=CARTESIAN_POINT('Ctrl Pts',(-1.93915639211581,-1.,0.169534904817491));
#29763=CARTESIAN_POINT('Ctrl Pts',(-1.93915639211581,1.,0.169534904817491));
#29764=CARTESIAN_POINT('Ctrl Pts',(-1.93329183155539,-1.,0.170541253116201));
#29765=CARTESIAN_POINT('Ctrl Pts',(-1.93329183155539,1.,0.170541253116201));
#29766=CARTESIAN_POINT('Ctrl Pts',(-1.92731093582036,-1.,0.171471191532988));
#29767=CARTESIAN_POINT('Ctrl Pts',(-1.92731093582036,1.,0.171471191532988));
#29768=CARTESIAN_POINT('Ctrl Pts',(-1.9212233439798,-1.,0.172321621259514));
#29769=CARTESIAN_POINT('Ctrl Pts',(-1.9212233439798,1.,0.172321621259514));
#29770=CARTESIAN_POINT('Ctrl Pts',(-1.91511429159527,-1.,0.173090695383496));
#29771=CARTESIAN_POINT('Ctrl Pts',(-1.91511429159527,1.,0.173090695383496));
#29772=CARTESIAN_POINT('Ctrl Pts',(-1.90911693975267,-1.,0.173776635257817));
#29773=CARTESIAN_POINT('Ctrl Pts',(-1.90911693975267,1.,0.173776635257817));
#29774=CARTESIAN_POINT('Ctrl Pts',(-1.90335253862834,-1.,0.174375518661085));
#29775=CARTESIAN_POINT('Ctrl Pts',(-1.90335253862834,1.,0.174375518661085));
#29776=CARTESIAN_POINT('Ctrl Pts',(-1.89788101117132,-1.,0.174879405091263));
#29777=CARTESIAN_POINT('Ctrl Pts',(-1.89788101117132,1.,0.174879405091263));
#29778=CARTESIAN_POINT('Ctrl Pts',(-1.892646301985,-1.,0.175274276190844));
#29779=CARTESIAN_POINT('Ctrl Pts',(-1.892646301985,1.,0.175274276190844));
#29780=CARTESIAN_POINT('Ctrl Pts',(-1.88742606273259,-1.,0.175538155840648));
#29781=CARTESIAN_POINT('Ctrl Pts',(-1.88742606273259,1.,0.175538155840648));
#29782=CARTESIAN_POINT('Ctrl Pts',(-1.88188663145367,-1.,0.175644148889698));
#29783=CARTESIAN_POINT('Ctrl Pts',(-1.88188663145367,1.,0.175644148889698));
#29784=CARTESIAN_POINT('Ctrl Pts',(-1.87563767773588,-1.,0.175563480746485));
#29785=CARTESIAN_POINT('Ctrl Pts',(-1.87563767773588,1.,0.175563480746485));
#29786=CARTESIAN_POINT('Ctrl Pts',(-1.86828349694799,-1.,0.175268337590758));
#29787=CARTESIAN_POINT('Ctrl Pts',(-1.86828349694799,1.,0.175268337590758));
#29788=CARTESIAN_POINT('Ctrl Pts',(-1.85948367088837,-1.,0.17473525927603));
#29789=CARTESIAN_POINT('Ctrl Pts',(-1.85948367088837,1.,0.17473525927603));
#29790=CARTESIAN_POINT('Ctrl Pts',(-1.8489811319852,-1.,0.173946627587731));
#29791=CARTESIAN_POINT('Ctrl Pts',(-1.8489811319852,1.,0.173946627587731));
#29792=CARTESIAN_POINT('Ctrl Pts',(-1.83658380527692,-1.,0.1728894428919));
#29793=CARTESIAN_POINT('Ctrl Pts',(-1.83658380527692,1.,0.1728894428919));
#29794=CARTESIAN_POINT('Ctrl Pts',(-1.82215766811545,-1.,0.171554770204119));
#29795=CARTESIAN_POINT('Ctrl Pts',(-1.82215766811545,1.,0.171554770204119));
#29796=CARTESIAN_POINT('Ctrl Pts',(-1.80561530629706,-1.,0.169936923904608));
#29797=CARTESIAN_POINT('Ctrl Pts',(-1.80561530629706,1.,0.169936923904608));
#29798=CARTESIAN_POINT('Ctrl Pts',(-1.7869064998507,-1.,0.168032772805197));
#29799=CARTESIAN_POINT('Ctrl Pts',(-1.7869064998507,1.,0.168032772805197));
#29800=CARTESIAN_POINT('Ctrl Pts',(-1.77018771684844,-1.,0.1662793551464));
#29801=CARTESIAN_POINT('Ctrl Pts',(-1.77018771684844,1.,0.1662793551464));
#29802=CARTESIAN_POINT('Ctrl Pts',(-1.75666056638427,-1.,0.164834765707158));
#29803=CARTESIAN_POINT('Ctrl Pts',(-1.75666056638427,1.,0.164834765707158));
#29804=CARTESIAN_POINT('Ctrl Pts',(-1.7472034950333,-1.,0.163814161002002));
#29805=CARTESIAN_POINT('Ctrl Pts',(-1.7472034950333,1.,0.163814161002002));
#29806=CARTESIAN_POINT('Ctrl Pts',(-1.74236521665491,-1.,0.163289472382896));
#29807=CARTESIAN_POINT('Ctrl Pts',(-1.74236521665491,1.,0.163289472382896));
#29808=CARTESIAN_POINT('',(-2.19890268624765,1.,0.069476445021958));
#29809=CARTESIAN_POINT('Ctrl Pts',(-2.19890268624765,1.,0.069476445021958));
#29810=CARTESIAN_POINT('Ctrl Pts',(-2.19777582085423,1.,0.0701143536325489));
#29811=CARTESIAN_POINT('Ctrl Pts',(-2.19552129484002,1.,0.0713863779526153));
#29812=CARTESIAN_POINT('Ctrl Pts',(-2.19213712013662,1.,0.0732830357306724));
#29813=CARTESIAN_POINT('Ctrl Pts',(-2.1876201139953,1.,0.0757891465836146));
#29814=CARTESIAN_POINT('Ctrl Pts',(-2.18196589448887,1.,0.0788837727685241));
#29815=CARTESIAN_POINT('Ctrl Pts',(-2.176303712113,1.,0.0819402680872764));
#29816=CARTESIAN_POINT('Ctrl Pts',(-2.17063357870952,1.,0.0849584620835371));
#29817=CARTESIAN_POINT('Ctrl Pts',(-2.16495552645014,1.,0.0879381291386921));
#29818=CARTESIAN_POINT('Ctrl Pts',(-2.15926961544516,1.,0.0908789888107264));
#29819=CARTESIAN_POINT('Ctrl Pts',(-2.1535759397817,1.,0.0937807218867642));
#29820=CARTESIAN_POINT('Ctrl Pts',(-2.14787463531795,1.,0.0966429852305457));
#29821=CARTESIAN_POINT('Ctrl Pts',(-2.14216588396025,1.,0.0994654261990914));
#29822=CARTESIAN_POINT('Ctrl Pts',(-2.13644992667165,1.,0.1022477005561));
#29823=CARTESIAN_POINT('Ctrl Pts',(-2.13072704887293,1.,0.104989479152739));
#29824=CARTESIAN_POINT('Ctrl Pts',(-2.12499752307,1.,0.10769043523109));
#29825=CARTESIAN_POINT('Ctrl Pts',(-2.11926155590865,1.,0.110350236135025));
#29826=CARTESIAN_POINT('Ctrl Pts',(-2.11351924490306,1.,0.112968534419737));
#29827=CARTESIAN_POINT('Ctrl Pts',(-2.10777050261309,1.,0.115544957687926));
#29828=CARTESIAN_POINT('Ctrl Pts',(-2.102015121329,1.,0.118079107988355));
#29829=CARTESIAN_POINT('Ctrl Pts',(-2.0962529286773,1.,0.120570567965122));
#29830=CARTESIAN_POINT('Ctrl Pts',(-2.09048392424825,1.,0.123018905621083));
#29831=CARTESIAN_POINT('Ctrl Pts',(-2.08470840653643,1.,0.125423679412061));
#29832=CARTESIAN_POINT('Ctrl Pts',(-2.07892715110987,1.,0.12778444527612));
#29833=CARTESIAN_POINT('Ctrl Pts',(-2.07314114713063,1.,0.130100748328403));
#29834=CARTESIAN_POINT('Ctrl Pts',(-2.06735123910326,1.,0.13237211154771));
#29835=CARTESIAN_POINT('Ctrl Pts',(-2.06155781517842,1.,0.134598026192106));
#29836=CARTESIAN_POINT('Ctrl Pts',(-2.05576044414264,1.,0.136777941218043));
#29837=CARTESIAN_POINT('Ctrl Pts',(-2.04995762001328,1.,0.138911255368966));
#29838=CARTESIAN_POINT('Ctrl Pts',(-2.04414757947916,1.,0.140997332152546));
#29839=CARTESIAN_POINT('Ctrl Pts',(-2.03832911025912,1.,0.143035515058209));
#29840=CARTESIAN_POINT('Ctrl Pts',(-2.03250223739942,1.,0.145025140186057));
#29841=CARTESIAN_POINT('Ctrl Pts',(-2.02666926182017,1.,0.146965557332583));
#29842=CARTESIAN_POINT('Ctrl Pts',(-2.02083464969894,1.,0.148856124775337));
#29843=CARTESIAN_POINT('Ctrl Pts',(-2.01500291940238,1.,0.150696157673078));
#29844=CARTESIAN_POINT('Ctrl Pts',(-2.00917680318424,1.,0.15248488362145));
#29845=CARTESIAN_POINT('Ctrl Pts',(-2.00335565310543,1.,0.154221403049722));
#29846=CARTESIAN_POINT('Ctrl Pts',(-1.99753284771497,1.,0.155904629548783));
#29847=CARTESIAN_POINT('Ctrl Pts',(-1.99169810931908,1.,0.157533331459227));
#29848=CARTESIAN_POINT('Ctrl Pts',(-1.98584238283292,1.,0.159106226437299));
#29849=CARTESIAN_POINT('Ctrl Pts',(-1.97996195437559,1.,0.160622060784611));
#29850=CARTESIAN_POINT('Ctrl Pts',(-1.97406280235188,1.,0.162079693556288));
#29851=CARTESIAN_POINT('Ctrl Pts',(-1.96816512677967,1.,0.163478185457734));
#29852=CARTESIAN_POINT('Ctrl Pts',(-1.96229379940136,1.,0.164816568920269));
#29853=CARTESIAN_POINT('Ctrl Pts',(-1.9564675971873,1.,0.166093592002812));
#29854=CARTESIAN_POINT('Ctrl Pts',(-1.95069027794294,1.,0.167307501784475));
#29855=CARTESIAN_POINT('Ctrl Pts',(-1.94493757756931,1.,0.168455741607556));
#29856=CARTESIAN_POINT('Ctrl Pts',(-1.93915639211581,1.,0.169534904817491));
#29857=CARTESIAN_POINT('Ctrl Pts',(-1.93329183155539,1.,0.170541253116201));
#29858=CARTESIAN_POINT('Ctrl Pts',(-1.92731093582036,1.,0.171471191532988));
#29859=CARTESIAN_POINT('Ctrl Pts',(-1.9212233439798,1.,0.172321621259514));
#29860=CARTESIAN_POINT('Ctrl Pts',(-1.91511429159527,1.,0.173090695383496));
#29861=CARTESIAN_POINT('Ctrl Pts',(-1.90911693975267,1.,0.173776635257817));
#29862=CARTESIAN_POINT('Ctrl Pts',(-1.90335253862834,1.,0.174375518661085));
#29863=CARTESIAN_POINT('Ctrl Pts',(-1.89788101117132,1.,0.174879405091263));
#29864=CARTESIAN_POINT('Ctrl Pts',(-1.892646301985,1.,0.175274276190844));
#29865=CARTESIAN_POINT('Ctrl Pts',(-1.88742606273259,1.,0.175538155840648));
#29866=CARTESIAN_POINT('Ctrl Pts',(-1.88188663145367,1.,0.175644148889698));
#29867=CARTESIAN_POINT('Ctrl Pts',(-1.87563767773588,1.,0.175563480746485));
#29868=CARTESIAN_POINT('Ctrl Pts',(-1.86828349694799,1.,0.175268337590758));
#29869=CARTESIAN_POINT('Ctrl Pts',(-1.85948367088837,1.,0.17473525927603));
#29870=CARTESIAN_POINT('Ctrl Pts',(-1.8489811319852,1.,0.173946627587731));
#29871=CARTESIAN_POINT('Ctrl Pts',(-1.83658380527692,1.,0.1728894428919));
#29872=CARTESIAN_POINT('Ctrl Pts',(-1.82215766811545,1.,0.171554770204119));
#29873=CARTESIAN_POINT('Ctrl Pts',(-1.80561530629706,1.,0.169936923904608));
#29874=CARTESIAN_POINT('Ctrl Pts',(-1.7869064998507,1.,0.168032772805197));
#29875=CARTESIAN_POINT('Ctrl Pts',(-1.77018771684844,1.,0.1662793551464));
#29876=CARTESIAN_POINT('Ctrl Pts',(-1.75666056638427,1.,0.164834765707158));
#29877=CARTESIAN_POINT('Ctrl Pts',(-1.7472034950333,1.,0.163814161002002));
#29878=CARTESIAN_POINT('Ctrl Pts',(-1.74236521665491,1.,0.163289472382896));
#29879=CARTESIAN_POINT('',(-2.19890268624765,0.,0.069476445021958));
#29880=CARTESIAN_POINT('Origin',(-2.19890268624765,0.,-0.0694764450219585));
#29881=CARTESIAN_POINT('',(-2.19890268624765,1.,-0.0694764450219585));
#29882=CARTESIAN_POINT('',(-2.19890268624765,1.,0.069476445021958));
#29883=CARTESIAN_POINT('',(-2.19890268624765,0.,-0.0694764450219585));
#29884=CARTESIAN_POINT('Ctrl Pts',(-1.74236521665491,-1.,-0.163289472382896));
#29885=CARTESIAN_POINT('Ctrl Pts',(-1.74236521665491,1.,-0.163289472382896));
#29886=CARTESIAN_POINT('Ctrl Pts',(-1.74720349503904,-1.,-0.163814161002474));
#29887=CARTESIAN_POINT('Ctrl Pts',(-1.74720349503904,1.,-0.163814161002474));
#29888=CARTESIAN_POINT('Ctrl Pts',(-1.75666056640041,-1.,-0.164834765708484));
#29889=CARTESIAN_POINT('Ctrl Pts',(-1.75666056640041,1.,-0.164834765708484));
#29890=CARTESIAN_POINT('Ctrl Pts',(-1.77018771687692,-1.,-0.166279355148738));
#29891=CARTESIAN_POINT('Ctrl Pts',(-1.77018771687692,1.,-0.166279355148738));
#29892=CARTESIAN_POINT('Ctrl Pts',(-1.78690649988931,-1.,-0.16803277280837));
#29893=CARTESIAN_POINT('Ctrl Pts',(-1.78690649988931,1.,-0.16803277280837));
#29894=CARTESIAN_POINT('Ctrl Pts',(-1.80561530633924,-1.,-0.169936923908078));
#29895=CARTESIAN_POINT('Ctrl Pts',(-1.80561530633924,1.,-0.169936923908078));
#29896=CARTESIAN_POINT('Ctrl Pts',(-1.82215766815414,-1.,-0.171554770207306));
#29897=CARTESIAN_POINT('Ctrl Pts',(-1.82215766815414,1.,-0.171554770207306));
#29898=CARTESIAN_POINT('Ctrl Pts',(-1.83658380530747,-1.,-0.17288944289442));
#29899=CARTESIAN_POINT('Ctrl Pts',(-1.83658380530747,1.,-0.17288944289442));
#29900=CARTESIAN_POINT('Ctrl Pts',(-1.84898113200543,-1.,-0.173946627589401));
#29901=CARTESIAN_POINT('Ctrl Pts',(-1.84898113200543,1.,-0.173946627589401));
#29902=CARTESIAN_POINT('Ctrl Pts',(-1.85948367089838,-1.,-0.174735259276856));
#29903=CARTESIAN_POINT('Ctrl Pts',(-1.85948367089838,1.,-0.174735259276856));
#29904=CARTESIAN_POINT('Ctrl Pts',(-1.86828349694972,-1.,-0.175268337590901));
#29905=CARTESIAN_POINT('Ctrl Pts',(-1.86828349694972,1.,-0.175268337590901));
#29906=CARTESIAN_POINT('Ctrl Pts',(-1.87563767773249,-1.,-0.175563480746205));
#29907=CARTESIAN_POINT('Ctrl Pts',(-1.87563767773249,1.,-0.175563480746205));
#29908=CARTESIAN_POINT('Ctrl Pts',(-1.88188663144846,-1.,-0.175644148889271));
#29909=CARTESIAN_POINT('Ctrl Pts',(-1.88188663144846,1.,-0.175644148889271));
#29910=CARTESIAN_POINT('Ctrl Pts',(-1.88742606272818,-1.,-0.175538155840286));
#29911=CARTESIAN_POINT('Ctrl Pts',(-1.88742606272818,1.,-0.175538155840286));
#29912=CARTESIAN_POINT('Ctrl Pts',(-1.89264630198279,-1.,-0.175274276190664));
#29913=CARTESIAN_POINT('Ctrl Pts',(-1.89264630198279,1.,-0.175274276190664));
#29914=CARTESIAN_POINT('Ctrl Pts',(-1.89788101117148,-1.,-0.174879405091277));
#29915=CARTESIAN_POINT('Ctrl Pts',(-1.89788101117148,1.,-0.174879405091277));
#29916=CARTESIAN_POINT('Ctrl Pts',(-1.90335253863003,-1.,-0.174375518661222));
#29917=CARTESIAN_POINT('Ctrl Pts',(-1.90335253863003,1.,-0.174375518661222));
#29918=CARTESIAN_POINT('Ctrl Pts',(-1.90911693975475,-1.,-0.173776635257984));
#29919=CARTESIAN_POINT('Ctrl Pts',(-1.90911693975475,1.,-0.173776635257984));
#29920=CARTESIAN_POINT('Ctrl Pts',(-1.91511429159681,-1.,-0.173090695383619));
#29921=CARTESIAN_POINT('Ctrl Pts',(-1.91511429159681,1.,-0.173090695383619));
#29922=CARTESIAN_POINT('Ctrl Pts',(-1.92122334398034,-1.,-0.172321621259557));
#29923=CARTESIAN_POINT('Ctrl Pts',(-1.92122334398034,1.,-0.172321621259557));
#29924=CARTESIAN_POINT('Ctrl Pts',(-1.92731093582,-1.,-0.17147119153296));
#29925=CARTESIAN_POINT('Ctrl Pts',(-1.92731093582,1.,-0.17147119153296));
#29926=CARTESIAN_POINT('Ctrl Pts',(-1.93329183155455,-1.,-0.170541253116136));
#29927=CARTESIAN_POINT('Ctrl Pts',(-1.93329183155455,1.,-0.170541253116136));
#29928=CARTESIAN_POINT('Ctrl Pts',(-1.93915639211497,-1.,-0.169534904817425));
#29929=CARTESIAN_POINT('Ctrl Pts',(-1.93915639211497,1.,-0.169534904817425));
#29930=CARTESIAN_POINT('Ctrl Pts',(-1.94493757756879,-1.,-0.168455741607516));
#29931=CARTESIAN_POINT('Ctrl Pts',(-1.94493757756879,1.,-0.168455741607516));
#29932=CARTESIAN_POINT('Ctrl Pts',(-1.95069027794286,-1.,-0.167307501784469));
#29933=CARTESIAN_POINT('Ctrl Pts',(-1.95069027794286,1.,-0.167307501784469));
#29934=CARTESIAN_POINT('Ctrl Pts',(-1.95646759718755,-1.,-0.166093592002833));
#29935=CARTESIAN_POINT('Ctrl Pts',(-1.95646759718755,1.,-0.166093592002833));
#29936=CARTESIAN_POINT('Ctrl Pts',(-1.96229379940174,-1.,-0.1648165689203));
#29937=CARTESIAN_POINT('Ctrl Pts',(-1.96229379940174,1.,-0.1648165689203));
#29938=CARTESIAN_POINT('Ctrl Pts',(-1.96816512678,-1.,-0.16347818545776));
#29939=CARTESIAN_POINT('Ctrl Pts',(-1.96816512678,1.,-0.16347818545776));
#29940=CARTESIAN_POINT('Ctrl Pts',(-1.97406280235204,-1.,-0.162079693556302));
#29941=CARTESIAN_POINT('Ctrl Pts',(-1.97406280235204,1.,-0.162079693556302));
#29942=CARTESIAN_POINT('Ctrl Pts',(-1.97996195437557,-1.,-0.16062206078461));
#29943=CARTESIAN_POINT('Ctrl Pts',(-1.97996195437557,1.,-0.16062206078461));
#29944=CARTESIAN_POINT('Ctrl Pts',(-1.98584238283279,-1.,-0.159106226437289));
#29945=CARTESIAN_POINT('Ctrl Pts',(-1.98584238283279,1.,-0.159106226437289));
#29946=CARTESIAN_POINT('Ctrl Pts',(-1.99169810931893,-1.,-0.157533331459215));
#29947=CARTESIAN_POINT('Ctrl Pts',(-1.99169810931893,1.,-0.157533331459215));
#29948=CARTESIAN_POINT('Ctrl Pts',(-1.99753284771487,-1.,-0.155904629548775));
#29949=CARTESIAN_POINT('Ctrl Pts',(-1.99753284771487,1.,-0.155904629548775));
#29950=CARTESIAN_POINT('Ctrl Pts',(-2.00335565310539,-1.,-0.154221403049719));
#29951=CARTESIAN_POINT('Ctrl Pts',(-2.00335565310539,1.,-0.154221403049719));
#29952=CARTESIAN_POINT('Ctrl Pts',(-2.00917680318426,-1.,-0.152484883621452));
#29953=CARTESIAN_POINT('Ctrl Pts',(-2.00917680318426,1.,-0.152484883621452));
#29954=CARTESIAN_POINT('Ctrl Pts',(-2.01500291940243,-1.,-0.150696157673084));
#29955=CARTESIAN_POINT('Ctrl Pts',(-2.01500291940243,1.,-0.150696157673084));
#29956=CARTESIAN_POINT('Ctrl Pts',(-2.02083464969897,-1.,-0.148856124775343));
#29957=CARTESIAN_POINT('Ctrl Pts',(-2.02083464969897,1.,-0.148856124775343));
#29958=CARTESIAN_POINT('Ctrl Pts',(-2.02666926182017,-1.,-0.146965557332586));
#29959=CARTESIAN_POINT('Ctrl Pts',(-2.02666926182017,1.,-0.146965557332586));
#29960=CARTESIAN_POINT('Ctrl Pts',(-2.03250223739941,-1.,-0.145025140186058));
#29961=CARTESIAN_POINT('Ctrl Pts',(-2.03250223739941,1.,-0.145025140186058));
#29962=CARTESIAN_POINT('Ctrl Pts',(-2.03832911025913,-1.,-0.143035515058208));
#29963=CARTESIAN_POINT('Ctrl Pts',(-2.03832911025913,1.,-0.143035515058208));
#29964=CARTESIAN_POINT('Ctrl Pts',(-2.04414757947919,-1.,-0.140997332152545));
#29965=CARTESIAN_POINT('Ctrl Pts',(-2.04414757947919,1.,-0.140997332152545));
#29966=CARTESIAN_POINT('Ctrl Pts',(-2.04995762001333,-1.,-0.138911255368966));
#29967=CARTESIAN_POINT('Ctrl Pts',(-2.04995762001333,1.,-0.138911255368966));
#29968=CARTESIAN_POINT('Ctrl Pts',(-2.0557604441427,-1.,-0.136777941218044));
#29969=CARTESIAN_POINT('Ctrl Pts',(-2.0557604441427,1.,-0.136777941218044));
#29970=CARTESIAN_POINT('Ctrl Pts',(-2.06155781517844,-1.,-0.134598026192107));
#29971=CARTESIAN_POINT('Ctrl Pts',(-2.06155781517844,1.,-0.134598026192107));
#29972=CARTESIAN_POINT('Ctrl Pts',(-2.06735123910319,-1.,-0.13237211154771));
#29973=CARTESIAN_POINT('Ctrl Pts',(-2.06735123910319,1.,-0.13237211154771));
#29974=CARTESIAN_POINT('Ctrl Pts',(-2.07314114713047,-1.,-0.130100748328401));
#29975=CARTESIAN_POINT('Ctrl Pts',(-2.07314114713047,1.,-0.130100748328401));
#29976=CARTESIAN_POINT('Ctrl Pts',(-2.07892715110967,-1.,-0.127784445276116));
#29977=CARTESIAN_POINT('Ctrl Pts',(-2.07892715110967,1.,-0.127784445276116));
#29978=CARTESIAN_POINT('Ctrl Pts',(-2.08470840653628,-1.,-0.125423679412058));
#29979=CARTESIAN_POINT('Ctrl Pts',(-2.08470840653628,1.,-0.125423679412058));
#29980=CARTESIAN_POINT('Ctrl Pts',(-2.09048392424826,-1.,-0.123018905621083));
#29981=CARTESIAN_POINT('Ctrl Pts',(-2.09048392424826,1.,-0.123018905621083));
#29982=CARTESIAN_POINT('Ctrl Pts',(-2.09625292867756,-1.,-0.120570567965129));
#29983=CARTESIAN_POINT('Ctrl Pts',(-2.09625292867756,1.,-0.120570567965129));
#29984=CARTESIAN_POINT('Ctrl Pts',(-2.10201512132945,-1.,-0.118079107988368));
#29985=CARTESIAN_POINT('Ctrl Pts',(-2.10201512132945,1.,-0.118079107988368));
#29986=CARTESIAN_POINT('Ctrl Pts',(-2.10777050261359,-1.,-0.11554495768794));
#29987=CARTESIAN_POINT('Ctrl Pts',(-2.10777050261359,1.,-0.11554495768794));
#29988=CARTESIAN_POINT('Ctrl Pts',(-2.11351924490335,-1.,-0.112968534419746));
#29989=CARTESIAN_POINT('Ctrl Pts',(-2.11351924490335,1.,-0.112968534419746));
#29990=CARTESIAN_POINT('Ctrl Pts',(-2.11926155590849,-1.,-0.11035023613502));
#29991=CARTESIAN_POINT('Ctrl Pts',(-2.11926155590849,1.,-0.11035023613502));
#29992=CARTESIAN_POINT('Ctrl Pts',(-2.12499752306927,-1.,-0.107690435231068));
#29993=CARTESIAN_POINT('Ctrl Pts',(-2.12499752306927,1.,-0.107690435231068));
#29994=CARTESIAN_POINT('Ctrl Pts',(-2.1307270488718,-1.,-0.104989479152703));
#29995=CARTESIAN_POINT('Ctrl Pts',(-2.1307270488718,1.,-0.104989479152703));
#29996=CARTESIAN_POINT('Ctrl Pts',(-2.13644992667052,-1.,-0.102247700556064));
#29997=CARTESIAN_POINT('Ctrl Pts',(-2.13644992667052,1.,-0.102247700556064));
#29998=CARTESIAN_POINT('Ctrl Pts',(-2.14216588395974,-1.,-0.0994654261990744));
#29999=CARTESIAN_POINT('Ctrl Pts',(-2.14216588395974,1.,-0.0994654261990744));
#30000=CARTESIAN_POINT('Ctrl Pts',(-2.14787463531864,-1.,-0.096642985230569));
#30001=CARTESIAN_POINT('Ctrl Pts',(-2.14787463531864,1.,-0.096642985230569));
#30002=CARTESIAN_POINT('Ctrl Pts',(-2.15357593978377,-1.,-0.0937807218868346));
#30003=CARTESIAN_POINT('Ctrl Pts',(-2.15357593978377,1.,-0.0937807218868346));
#30004=CARTESIAN_POINT('Ctrl Pts',(-2.15926961544808,-1.,-0.0908789888108267));
#30005=CARTESIAN_POINT('Ctrl Pts',(-2.15926961544808,1.,-0.0908789888108267));
#30006=CARTESIAN_POINT('Ctrl Pts',(-2.16495552645275,-1.,-0.0879381291387824));
#30007=CARTESIAN_POINT('Ctrl Pts',(-2.16495552645275,1.,-0.0879381291387824));
#30008=CARTESIAN_POINT('Ctrl Pts',(-2.17063357871031,-1.,-0.0849584620835644));
#30009=CARTESIAN_POINT('Ctrl Pts',(-2.17063357871031,1.,-0.0849584620835644));
#30010=CARTESIAN_POINT('Ctrl Pts',(-2.1763037121106,-1.,-0.0819402680871941));
#30011=CARTESIAN_POINT('Ctrl Pts',(-2.1763037121106,1.,-0.0819402680871941));
#30012=CARTESIAN_POINT('Ctrl Pts',(-2.18196589448304,-1.,-0.0788837727683229));
#30013=CARTESIAN_POINT('Ctrl Pts',(-2.18196589448304,1.,-0.0788837727683229));
#30014=CARTESIAN_POINT('Ctrl Pts',(-2.1876201139874,-1.,-0.0757891465833413));
#30015=CARTESIAN_POINT('Ctrl Pts',(-2.1876201139874,1.,-0.0757891465833413));
#30016=CARTESIAN_POINT('Ctrl Pts',(-2.19213712012956,-1.,-0.0732830357304277));
#30017=CARTESIAN_POINT('Ctrl Pts',(-2.19213712012956,1.,-0.0732830357304277));
#30018=CARTESIAN_POINT('Ctrl Pts',(-2.19552129483562,-1.,-0.0713863779524629));
#30019=CARTESIAN_POINT('Ctrl Pts',(-2.19552129483562,1.,-0.0713863779524629));
#30020=CARTESIAN_POINT('Ctrl Pts',(-2.19777582085261,-1.,-0.0701143536324927));
#30021=CARTESIAN_POINT('Ctrl Pts',(-2.19777582085261,1.,-0.0701143536324927));
#30022=CARTESIAN_POINT('Ctrl Pts',(-2.19890268624765,-1.,-0.0694764450219585));
#30023=CARTESIAN_POINT('Ctrl Pts',(-2.19890268624765,1.,-0.0694764450219585));
#30024=CARTESIAN_POINT('',(-1.74236521665491,1.,-0.163289472382896));
#30025=CARTESIAN_POINT('Ctrl Pts',(-1.74236521665491,1.,-0.163289472382896));
#30026=CARTESIAN_POINT('Ctrl Pts',(-1.74720349503904,1.,-0.163814161002474));
#30027=CARTESIAN_POINT('Ctrl Pts',(-1.75666056640041,1.,-0.164834765708484));
#30028=CARTESIAN_POINT('Ctrl Pts',(-1.77018771687692,1.,-0.166279355148738));
#30029=CARTESIAN_POINT('Ctrl Pts',(-1.78690649988931,1.,-0.16803277280837));
#30030=CARTESIAN_POINT('Ctrl Pts',(-1.80561530633924,1.,-0.169936923908078));
#30031=CARTESIAN_POINT('Ctrl Pts',(-1.82215766815414,1.,-0.171554770207306));
#30032=CARTESIAN_POINT('Ctrl Pts',(-1.83658380530747,1.,-0.17288944289442));
#30033=CARTESIAN_POINT('Ctrl Pts',(-1.84898113200543,1.,-0.173946627589401));
#30034=CARTESIAN_POINT('Ctrl Pts',(-1.85948367089838,1.,-0.174735259276856));
#30035=CARTESIAN_POINT('Ctrl Pts',(-1.86828349694972,1.,-0.175268337590901));
#30036=CARTESIAN_POINT('Ctrl Pts',(-1.87563767773249,1.,-0.175563480746205));
#30037=CARTESIAN_POINT('Ctrl Pts',(-1.88188663144846,1.,-0.175644148889271));
#30038=CARTESIAN_POINT('Ctrl Pts',(-1.88742606272818,1.,-0.175538155840286));
#30039=CARTESIAN_POINT('Ctrl Pts',(-1.89264630198279,1.,-0.175274276190664));
#30040=CARTESIAN_POINT('Ctrl Pts',(-1.89788101117148,1.,-0.174879405091277));
#30041=CARTESIAN_POINT('Ctrl Pts',(-1.90335253863003,1.,-0.174375518661222));
#30042=CARTESIAN_POINT('Ctrl Pts',(-1.90911693975475,1.,-0.173776635257984));
#30043=CARTESIAN_POINT('Ctrl Pts',(-1.91511429159681,1.,-0.173090695383619));
#30044=CARTESIAN_POINT('Ctrl Pts',(-1.92122334398034,1.,-0.172321621259557));
#30045=CARTESIAN_POINT('Ctrl Pts',(-1.92731093582,1.,-0.17147119153296));
#30046=CARTESIAN_POINT('Ctrl Pts',(-1.93329183155455,1.,-0.170541253116136));
#30047=CARTESIAN_POINT('Ctrl Pts',(-1.93915639211497,1.,-0.169534904817425));
#30048=CARTESIAN_POINT('Ctrl Pts',(-1.94493757756879,1.,-0.168455741607516));
#30049=CARTESIAN_POINT('Ctrl Pts',(-1.95069027794286,1.,-0.167307501784469));
#30050=CARTESIAN_POINT('Ctrl Pts',(-1.95646759718755,1.,-0.166093592002833));
#30051=CARTESIAN_POINT('Ctrl Pts',(-1.96229379940174,1.,-0.1648165689203));
#30052=CARTESIAN_POINT('Ctrl Pts',(-1.96816512678,1.,-0.16347818545776));
#30053=CARTESIAN_POINT('Ctrl Pts',(-1.97406280235204,1.,-0.162079693556302));
#30054=CARTESIAN_POINT('Ctrl Pts',(-1.97996195437557,1.,-0.16062206078461));
#30055=CARTESIAN_POINT('Ctrl Pts',(-1.98584238283279,1.,-0.159106226437289));
#30056=CARTESIAN_POINT('Ctrl Pts',(-1.99169810931893,1.,-0.157533331459215));
#30057=CARTESIAN_POINT('Ctrl Pts',(-1.99753284771487,1.,-0.155904629548775));
#30058=CARTESIAN_POINT('Ctrl Pts',(-2.00335565310539,1.,-0.154221403049719));
#30059=CARTESIAN_POINT('Ctrl Pts',(-2.00917680318426,1.,-0.152484883621452));
#30060=CARTESIAN_POINT('Ctrl Pts',(-2.01500291940243,1.,-0.150696157673084));
#30061=CARTESIAN_POINT('Ctrl Pts',(-2.02083464969897,1.,-0.148856124775343));
#30062=CARTESIAN_POINT('Ctrl Pts',(-2.02666926182017,1.,-0.146965557332586));
#30063=CARTESIAN_POINT('Ctrl Pts',(-2.03250223739941,1.,-0.145025140186058));
#30064=CARTESIAN_POINT('Ctrl Pts',(-2.03832911025913,1.,-0.143035515058208));
#30065=CARTESIAN_POINT('Ctrl Pts',(-2.04414757947919,1.,-0.140997332152545));
#30066=CARTESIAN_POINT('Ctrl Pts',(-2.04995762001333,1.,-0.138911255368966));
#30067=CARTESIAN_POINT('Ctrl Pts',(-2.0557604441427,1.,-0.136777941218044));
#30068=CARTESIAN_POINT('Ctrl Pts',(-2.06155781517844,1.,-0.134598026192107));
#30069=CARTESIAN_POINT('Ctrl Pts',(-2.06735123910319,1.,-0.13237211154771));
#30070=CARTESIAN_POINT('Ctrl Pts',(-2.07314114713047,1.,-0.130100748328401));
#30071=CARTESIAN_POINT('Ctrl Pts',(-2.07892715110967,1.,-0.127784445276116));
#30072=CARTESIAN_POINT('Ctrl Pts',(-2.08470840653628,1.,-0.125423679412058));
#30073=CARTESIAN_POINT('Ctrl Pts',(-2.09048392424826,1.,-0.123018905621083));
#30074=CARTESIAN_POINT('Ctrl Pts',(-2.09625292867756,1.,-0.120570567965129));
#30075=CARTESIAN_POINT('Ctrl Pts',(-2.10201512132945,1.,-0.118079107988368));
#30076=CARTESIAN_POINT('Ctrl Pts',(-2.10777050261359,1.,-0.11554495768794));
#30077=CARTESIAN_POINT('Ctrl Pts',(-2.11351924490335,1.,-0.112968534419746));
#30078=CARTESIAN_POINT('Ctrl Pts',(-2.11926155590849,1.,-0.11035023613502));
#30079=CARTESIAN_POINT('Ctrl Pts',(-2.12499752306927,1.,-0.107690435231068));
#30080=CARTESIAN_POINT('Ctrl Pts',(-2.1307270488718,1.,-0.104989479152703));
#30081=CARTESIAN_POINT('Ctrl Pts',(-2.13644992667052,1.,-0.102247700556064));
#30082=CARTESIAN_POINT('Ctrl Pts',(-2.14216588395974,1.,-0.0994654261990744));
#30083=CARTESIAN_POINT('Ctrl Pts',(-2.14787463531864,1.,-0.096642985230569));
#30084=CARTESIAN_POINT('Ctrl Pts',(-2.15357593978377,1.,-0.0937807218868346));
#30085=CARTESIAN_POINT('Ctrl Pts',(-2.15926961544808,1.,-0.0908789888108267));
#30086=CARTESIAN_POINT('Ctrl Pts',(-2.16495552645275,1.,-0.0879381291387824));
#30087=CARTESIAN_POINT('Ctrl Pts',(-2.17063357871031,1.,-0.0849584620835644));
#30088=CARTESIAN_POINT('Ctrl Pts',(-2.1763037121106,1.,-0.0819402680871941));
#30089=CARTESIAN_POINT('Ctrl Pts',(-2.18196589448304,1.,-0.0788837727683229));
#30090=CARTESIAN_POINT('Ctrl Pts',(-2.1876201139874,1.,-0.0757891465833413));
#30091=CARTESIAN_POINT('Ctrl Pts',(-2.19213712012956,1.,-0.0732830357304277));
#30092=CARTESIAN_POINT('Ctrl Pts',(-2.19552129483562,1.,-0.0713863779524629));
#30093=CARTESIAN_POINT('Ctrl Pts',(-2.19777582085261,1.,-0.0701143536324927));
#30094=CARTESIAN_POINT('Ctrl Pts',(-2.19890268624765,1.,-0.0694764450219585));
#30095=CARTESIAN_POINT('',(-1.74236521665491,0.,-0.163289472382896));
#30096=CARTESIAN_POINT('Origin',(0.,0.,0.));
#30097=CARTESIAN_POINT('',(-1.7075470150345,1.,-0.383122945602004));
#30098=CARTESIAN_POINT('Origin',(0.,1.,0.));
#30099=CARTESIAN_POINT('',(-1.7075470150345,0.,-0.383122945602004));
#30100=CARTESIAN_POINT('Ctrl Pts',(-2.11275013067528,-1.,-0.61342227326009));
#30101=CARTESIAN_POINT('Ctrl Pts',(-2.11275013067528,1.,-0.61342227326009));
#30102=CARTESIAN_POINT('Ctrl Pts',(-2.11187554260142,-1.,-0.61246736556225));
#30103=CARTESIAN_POINT('Ctrl Pts',(-2.11187554260142,1.,-0.61246736556225));
#30104=CARTESIAN_POINT('Ctrl Pts',(-2.11012443807661,-1.,-0.610560911691113));
#30105=CARTESIAN_POINT('Ctrl Pts',(-2.11012443807661,1.,-0.610560911691113));
#30106=CARTESIAN_POINT('Ctrl Pts',(-2.10749199615859,-1.,-0.607711315456826));
#30107=CARTESIAN_POINT('Ctrl Pts',(-2.10749199615859,1.,-0.607711315456826));
#30108=CARTESIAN_POINT('Ctrl Pts',(-2.10397049887709,-1.,-0.603932030738212));
#30109=CARTESIAN_POINT('Ctrl Pts',(-2.10397049887709,1.,-0.603932030738212));
#30110=CARTESIAN_POINT('Ctrl Pts',(-2.09954930865331,-1.,-0.599241616422144));
#30111=CARTESIAN_POINT('Ctrl Pts',(-2.09954930865331,1.,-0.599241616422144));
#30112=CARTESIAN_POINT('Ctrl Pts',(-2.09510876220501,-1.,-0.594585006052823));
#30113=CARTESIAN_POINT('Ctrl Pts',(-2.09510876220501,1.,-0.594585006052823));
#30114=CARTESIAN_POINT('Ctrl Pts',(-2.09064881812053,-1.,-0.589962365403189));
#30115=CARTESIAN_POINT('Ctrl Pts',(-2.09064881812053,1.,-0.589962365403189));
#30116=CARTESIAN_POINT('Ctrl Pts',(-2.086169437277,-1.,-0.585373918990895));
#30117=CARTESIAN_POINT('Ctrl Pts',(-2.086169437277,1.,-0.585373918990895));
#30118=CARTESIAN_POINT('Ctrl Pts',(-2.08167059018138,-1.,-0.580819952107257));
#30119=CARTESIAN_POINT('Ctrl Pts',(-2.08167059018138,1.,-0.580819952107257));
#30120=CARTESIAN_POINT('Ctrl Pts',(-2.07715226767361,-1.,-0.576300797416274));
#30121=CARTESIAN_POINT('Ctrl Pts',(-2.07715226767361,1.,-0.576300797416274));
#30122=CARTESIAN_POINT('Ctrl Pts',(-2.07261449292757,-1.,-0.571816823242411));
#30123=CARTESIAN_POINT('Ctrl Pts',(-2.07261449292757,1.,-0.571816823242411));
#30124=CARTESIAN_POINT('Ctrl Pts',(-2.06805732997383,-1.,-0.567368421181229));
#30125=CARTESIAN_POINT('Ctrl Pts',(-2.06805732997383,1.,-0.567368421181229));
#30126=CARTESIAN_POINT('Ctrl Pts',(-2.06348090160697,-1.,-0.562955993082574));
#30127=CARTESIAN_POINT('Ctrl Pts',(-2.06348090160697,1.,-0.562955993082574));
#30128=CARTESIAN_POINT('Ctrl Pts',(-2.05888537756571,-1.,-0.558579940185467));
#30129=CARTESIAN_POINT('Ctrl Pts',(-2.05888537756571,1.,-0.558579940185467));
#30130=CARTESIAN_POINT('Ctrl Pts',(-2.05427091604482,-1.,-0.554240657464109));
#30131=CARTESIAN_POINT('Ctrl Pts',(-2.05427091604482,1.,-0.554240657464109));
#30132=CARTESIAN_POINT('Ctrl Pts',(-2.04963761077974,-1.,-0.549938525150342));
#30133=CARTESIAN_POINT('Ctrl Pts',(-2.04963761077974,1.,-0.549938525150342));
#30134=CARTESIAN_POINT('Ctrl Pts',(-2.0449854471456,-1.,-0.545673903817348));
#30135=CARTESIAN_POINT('Ctrl Pts',(-2.0449854471456,1.,-0.545673903817348));
#30136=CARTESIAN_POINT('Ctrl Pts',(-2.0403142269048,-1.,-0.54144712061552));
#30137=CARTESIAN_POINT('Ctrl Pts',(-2.0403142269048,1.,-0.54144712061552));
#30138=CARTESIAN_POINT('Ctrl Pts',(-2.03562362953993,-1.,-0.537258489833134));
#30139=CARTESIAN_POINT('Ctrl Pts',(-2.03562362953993,1.,-0.537258489833134));
#30140=CARTESIAN_POINT('Ctrl Pts',(-2.03091336214401,-1.,-0.533108355132905));
#30141=CARTESIAN_POINT('Ctrl Pts',(-2.03091336214401,1.,-0.533108355132905));
#30142=CARTESIAN_POINT('Ctrl Pts',(-2.02618329083289,-1.,-0.52899712724191));
#30143=CARTESIAN_POINT('Ctrl Pts',(-2.02618329083289,1.,-0.52899712724191));
#30144=CARTESIAN_POINT('Ctrl Pts',(-2.02143356304712,-1.,-0.524925318333518));
#30145=CARTESIAN_POINT('Ctrl Pts',(-2.02143356304712,1.,-0.524925318333518));
#30146=CARTESIAN_POINT('Ctrl Pts',(-2.01666477917305,-1.,-0.520893590399428));
#30147=CARTESIAN_POINT('Ctrl Pts',(-2.01666477917305,1.,-0.520893590399428));
#30148=CARTESIAN_POINT('Ctrl Pts',(-2.01187773939257,-1.,-0.516902681728733));
#30149=CARTESIAN_POINT('Ctrl Pts',(-2.01187773939257,1.,-0.516902681728733));
#30150=CARTESIAN_POINT('Ctrl Pts',(-2.00707309946955,-1.,-0.512953306961813));
#30151=CARTESIAN_POINT('Ctrl Pts',(-2.00707309946955,1.,-0.512953306961813));
#30152=CARTESIAN_POINT('Ctrl Pts',(-2.00225107134733,-1.,-0.509046069886152));
#30153=CARTESIAN_POINT('Ctrl Pts',(-2.00225107134733,1.,-0.509046069886152));
#30154=CARTESIAN_POINT('Ctrl Pts',(-1.99741107463567,-1.,-0.505181361323011));
#30155=CARTESIAN_POINT('Ctrl Pts',(-1.99741107463567,1.,-0.505181361323011));
#30156=CARTESIAN_POINT('Ctrl Pts',(-1.9925514912615,-1.,-0.501359287727129));
#30157=CARTESIAN_POINT('Ctrl Pts',(-1.9925514912615,1.,-0.501359287727129));
#30158=CARTESIAN_POINT('Ctrl Pts',(-1.98767044752929,-1.,-0.497579909545564));
#30159=CARTESIAN_POINT('Ctrl Pts',(-1.98767044752929,1.,-0.497579909545564));
#30160=CARTESIAN_POINT('Ctrl Pts',(-1.9827665876182,-1.,-0.493843476541492));
#30161=CARTESIAN_POINT('Ctrl Pts',(-1.9827665876182,1.,-0.493843476541492));
#30162=CARTESIAN_POINT('Ctrl Pts',(-1.97783973019229,-1.,-0.490150627860955));
#30163=CARTESIAN_POINT('Ctrl Pts',(-1.97783973019229,1.,-0.490150627860955));
#30164=CARTESIAN_POINT('Ctrl Pts',(-1.97289186263272,-1.,-0.486502692907661));
#30165=CARTESIAN_POINT('Ctrl Pts',(-1.97289186263272,1.,-0.486502692907661));
#30166=CARTESIAN_POINT('Ctrl Pts',(-1.96792703422358,-1.,-0.482901662120686));
#30167=CARTESIAN_POINT('Ctrl Pts',(-1.96792703422358,1.,-0.482901662120686));
#30168=CARTESIAN_POINT('Ctrl Pts',(-1.96294933055938,-1.,-0.479349583074846));
#30169=CARTESIAN_POINT('Ctrl Pts',(-1.96294933055938,1.,-0.479349583074846));
#30170=CARTESIAN_POINT('Ctrl Pts',(-1.95796111148175,-1.,-0.475848034683171));
#30171=CARTESIAN_POINT('Ctrl Pts',(-1.95796111148175,1.,-0.475848034683171));
#30172=CARTESIAN_POINT('Ctrl Pts',(-1.95296148278136,-1.,-0.472397672264079));
#30173=CARTESIAN_POINT('Ctrl Pts',(-1.95296148278136,1.,-0.472397672264079));
#30174=CARTESIAN_POINT('Ctrl Pts',(-1.94794381136524,-1.,-0.468997482913158));
#30175=CARTESIAN_POINT('Ctrl Pts',(-1.94794381136524,1.,-0.468997482913158));
#30176=CARTESIAN_POINT('Ctrl Pts',(-1.94289794196205,-1.,-0.465645462026064));
#30177=CARTESIAN_POINT('Ctrl Pts',(-1.94289794196205,1.,-0.465645462026064));
#30178=CARTESIAN_POINT('Ctrl Pts',(-1.93781486640834,-1.,-0.462340031009087));
#30179=CARTESIAN_POINT('Ctrl Pts',(-1.93781486640834,1.,-0.462340031009087));
#30180=CARTESIAN_POINT('Ctrl Pts',(-1.93269066517936,-1.,-0.459081234547931));
#30181=CARTESIAN_POINT('Ctrl Pts',(-1.93269066517936,1.,-0.459081234547931));
#30182=CARTESIAN_POINT('Ctrl Pts',(-1.92753067150461,-1.,-0.455872005174335));
#30183=CARTESIAN_POINT('Ctrl Pts',(-1.92753067150461,1.,-0.455872005174335));
#30184=CARTESIAN_POINT('Ctrl Pts',(-1.9223538064847,-1.,-0.452719478359356));
#30185=CARTESIAN_POINT('Ctrl Pts',(-1.9223538064847,1.,-0.452719478359356));
#30186=CARTESIAN_POINT('Ctrl Pts',(-1.91718342555717,-1.,-0.449632260106572));
#30187=CARTESIAN_POINT('Ctrl Pts',(-1.91718342555717,1.,-0.449632260106572));
#30188=CARTESIAN_POINT('Ctrl Pts',(-1.91203699981095,-1.,-0.446617343485651));
#30189=CARTESIAN_POINT('Ctrl Pts',(-1.91203699981095,1.,-0.446617343485651));
#30190=CARTESIAN_POINT('Ctrl Pts',(-1.90691756144906,-1.,-0.44367755684917));
#30191=CARTESIAN_POINT('Ctrl Pts',(-1.90691756144906,1.,-0.44367755684917));
#30192=CARTESIAN_POINT('Ctrl Pts',(-1.90180124389137,-1.,-0.44080783370416));
#30193=CARTESIAN_POINT('Ctrl Pts',(-1.90180124389137,1.,-0.44080783370416));
#30194=CARTESIAN_POINT('Ctrl Pts',(-1.89663648956549,-1.,-0.437995003948443));
#30195=CARTESIAN_POINT('Ctrl Pts',(-1.89663648956549,1.,-0.437995003948443));
#30196=CARTESIAN_POINT('Ctrl Pts',(-1.89136993975585,-1.,-0.43522566096358));
#30197=CARTESIAN_POINT('Ctrl Pts',(-1.89136993975585,1.,-0.43522566096358));
#30198=CARTESIAN_POINT('Ctrl Pts',(-1.88596913666828,-1.,-0.432493038548833));
#30199=CARTESIAN_POINT('Ctrl Pts',(-1.88596913666828,1.,-0.432493038548833));
#30200=CARTESIAN_POINT('Ctrl Pts',(-1.88044229001778,-1.,-0.429803062482217));
#30201=CARTESIAN_POINT('Ctrl Pts',(-1.88044229001778,1.,-0.429803062482217));
#30202=CARTESIAN_POINT('Ctrl Pts',(-1.87486989291333,-1.,-0.427183828518743));
#30203=CARTESIAN_POINT('Ctrl Pts',(-1.87486989291333,1.,-0.427183828518743));
#30204=CARTESIAN_POINT('Ctrl Pts',(-1.8693780394412,-1.,-0.424678177290876));
#30205=CARTESIAN_POINT('Ctrl Pts',(-1.8693780394412,1.,-0.424678177290876));
#30206=CARTESIAN_POINT('Ctrl Pts',(-1.86408083333863,-1.,-0.422327307417884));
#30207=CARTESIAN_POINT('Ctrl Pts',(-1.86408083333863,1.,-0.422327307417884));
#30208=CARTESIAN_POINT('Ctrl Pts',(-1.8590328109667,-1.,-0.420157287975583));
#30209=CARTESIAN_POINT('Ctrl Pts',(-1.8590328109667,1.,-0.420157287975583));
#30210=CARTESIAN_POINT('Ctrl Pts',(-1.8541763285645,-1.,-0.418164129144045));
#30211=CARTESIAN_POINT('Ctrl Pts',(-1.8541763285645,1.,-0.418164129144045));
#30212=CARTESIAN_POINT('Ctrl Pts',(-1.84929312930314,-1.,-0.416300022039885));
#30213=CARTESIAN_POINT('Ctrl Pts',(-1.84929312930314,1.,-0.416300022039885));
#30214=CARTESIAN_POINT('Ctrl Pts',(-1.84405757074218,-1.,-0.414487438255542));
#30215=CARTESIAN_POINT('Ctrl Pts',(-1.84405757074218,1.,-0.414487438255542));
#30216=CARTESIAN_POINT('Ctrl Pts',(-1.8380895347617,-1.,-0.412633125322945));
#30217=CARTESIAN_POINT('Ctrl Pts',(-1.8380895347617,1.,-0.412633125322945));
#30218=CARTESIAN_POINT('Ctrl Pts',(-1.83100408895047,-1.,-0.410641256301276));
#30219=CARTESIAN_POINT('Ctrl Pts',(-1.83100408895047,1.,-0.410641256301276));
#30220=CARTESIAN_POINT('Ctrl Pts',(-1.82247022677562,-1.,-0.408428948106227));
#30221=CARTESIAN_POINT('Ctrl Pts',(-1.82247022677562,1.,-0.408428948106227));
#30222=CARTESIAN_POINT('Ctrl Pts',(-1.81223801812013,-1.,-0.405933518407175));
#30223=CARTESIAN_POINT('Ctrl Pts',(-1.81223801812013,1.,-0.405933518407175));
#30224=CARTESIAN_POINT('Ctrl Pts',(-1.80012077173238,-1.,-0.403107976163396));
#30225=CARTESIAN_POINT('Ctrl Pts',(-1.80012077173238,1.,-0.403107976163396));
#30226=CARTESIAN_POINT('Ctrl Pts',(-1.78598826343754,-1.,-0.399919403774155));
#30227=CARTESIAN_POINT('Ctrl Pts',(-1.78598826343754,1.,-0.399919403774155));
#30228=CARTESIAN_POINT('Ctrl Pts',(-1.76975560043442,-1.,-0.396346196110688));
#30229=CARTESIAN_POINT('Ctrl Pts',(-1.76975560043442,1.,-0.396346196110688));
#30230=CARTESIAN_POINT('Ctrl Pts',(-1.75137405310193,-1.,-0.392375812285395));
#30231=CARTESIAN_POINT('Ctrl Pts',(-1.75137405310193,1.,-0.392375812285395));
#30232=CARTESIAN_POINT('Ctrl Pts',(-1.73493170972829,-1.,-0.388877023502615));
#30233=CARTESIAN_POINT('Ctrl Pts',(-1.73493170972829,1.,-0.388877023502615));
#30234=CARTESIAN_POINT('Ctrl Pts',(-1.72162022244582,-1.,-0.386070790323281));
#30235=CARTESIAN_POINT('Ctrl Pts',(-1.72162022244582,1.,-0.386070790323281));
#30236=CARTESIAN_POINT('Ctrl Pts',(-1.71231062891398,-1.,-0.384119047314215));
#30237=CARTESIAN_POINT('Ctrl Pts',(-1.71231062891398,1.,-0.384119047314215));
#30238=CARTESIAN_POINT('Ctrl Pts',(-1.7075470150345,-1.,-0.383122945602004));
#30239=CARTESIAN_POINT('Ctrl Pts',(-1.7075470150345,1.,-0.383122945602004));
#30240=CARTESIAN_POINT('',(-2.11275013067528,1.,-0.61342227326009));
#30241=CARTESIAN_POINT('Ctrl Pts',(-2.11275013067528,1.,-0.61342227326009));
#30242=CARTESIAN_POINT('Ctrl Pts',(-2.11187554260142,1.,-0.61246736556225));
#30243=CARTESIAN_POINT('Ctrl Pts',(-2.11012443807661,1.,-0.610560911691113));
#30244=CARTESIAN_POINT('Ctrl Pts',(-2.10749199615859,1.,-0.607711315456826));
#30245=CARTESIAN_POINT('Ctrl Pts',(-2.10397049887709,1.,-0.603932030738212));
#30246=CARTESIAN_POINT('Ctrl Pts',(-2.09954930865331,1.,-0.599241616422144));
#30247=CARTESIAN_POINT('Ctrl Pts',(-2.09510876220501,1.,-0.594585006052823));
#30248=CARTESIAN_POINT('Ctrl Pts',(-2.09064881812053,1.,-0.589962365403189));
#30249=CARTESIAN_POINT('Ctrl Pts',(-2.086169437277,1.,-0.585373918990895));
#30250=CARTESIAN_POINT('Ctrl Pts',(-2.08167059018138,1.,-0.580819952107257));
#30251=CARTESIAN_POINT('Ctrl Pts',(-2.07715226767361,1.,-0.576300797416274));
#30252=CARTESIAN_POINT('Ctrl Pts',(-2.07261449292757,1.,-0.571816823242411));
#30253=CARTESIAN_POINT('Ctrl Pts',(-2.06805732997383,1.,-0.567368421181229));
#30254=CARTESIAN_POINT('Ctrl Pts',(-2.06348090160697,1.,-0.562955993082574));
#30255=CARTESIAN_POINT('Ctrl Pts',(-2.05888537756571,1.,-0.558579940185467));
#30256=CARTESIAN_POINT('Ctrl Pts',(-2.05427091604482,1.,-0.554240657464109));
#30257=CARTESIAN_POINT('Ctrl Pts',(-2.04963761077974,1.,-0.549938525150342));
#30258=CARTESIAN_POINT('Ctrl Pts',(-2.0449854471456,1.,-0.545673903817348));
#30259=CARTESIAN_POINT('Ctrl Pts',(-2.0403142269048,1.,-0.54144712061552));
#30260=CARTESIAN_POINT('Ctrl Pts',(-2.03562362953993,1.,-0.537258489833134));
#30261=CARTESIAN_POINT('Ctrl Pts',(-2.03091336214401,1.,-0.533108355132905));
#30262=CARTESIAN_POINT('Ctrl Pts',(-2.02618329083289,1.,-0.52899712724191));
#30263=CARTESIAN_POINT('Ctrl Pts',(-2.02143356304712,1.,-0.524925318333518));
#30264=CARTESIAN_POINT('Ctrl Pts',(-2.01666477917305,1.,-0.520893590399428));
#30265=CARTESIAN_POINT('Ctrl Pts',(-2.01187773939257,1.,-0.516902681728733));
#30266=CARTESIAN_POINT('Ctrl Pts',(-2.00707309946955,1.,-0.512953306961813));
#30267=CARTESIAN_POINT('Ctrl Pts',(-2.00225107134733,1.,-0.509046069886152));
#30268=CARTESIAN_POINT('Ctrl Pts',(-1.99741107463567,1.,-0.505181361323011));
#30269=CARTESIAN_POINT('Ctrl Pts',(-1.9925514912615,1.,-0.501359287727129));
#30270=CARTESIAN_POINT('Ctrl Pts',(-1.98767044752929,1.,-0.497579909545564));
#30271=CARTESIAN_POINT('Ctrl Pts',(-1.9827665876182,1.,-0.493843476541492));
#30272=CARTESIAN_POINT('Ctrl Pts',(-1.97783973019229,1.,-0.490150627860955));
#30273=CARTESIAN_POINT('Ctrl Pts',(-1.97289186263272,1.,-0.486502692907661));
#30274=CARTESIAN_POINT('Ctrl Pts',(-1.96792703422358,1.,-0.482901662120686));
#30275=CARTESIAN_POINT('Ctrl Pts',(-1.96294933055938,1.,-0.479349583074846));
#30276=CARTESIAN_POINT('Ctrl Pts',(-1.95796111148175,1.,-0.475848034683171));
#30277=CARTESIAN_POINT('Ctrl Pts',(-1.95296148278136,1.,-0.472397672264079));
#30278=CARTESIAN_POINT('Ctrl Pts',(-1.94794381136524,1.,-0.468997482913158));
#30279=CARTESIAN_POINT('Ctrl Pts',(-1.94289794196205,1.,-0.465645462026064));
#30280=CARTESIAN_POINT('Ctrl Pts',(-1.93781486640834,1.,-0.462340031009087));
#30281=CARTESIAN_POINT('Ctrl Pts',(-1.93269066517936,1.,-0.459081234547931));
#30282=CARTESIAN_POINT('Ctrl Pts',(-1.92753067150461,1.,-0.455872005174335));
#30283=CARTESIAN_POINT('Ctrl Pts',(-1.9223538064847,1.,-0.452719478359356));
#30284=CARTESIAN_POINT('Ctrl Pts',(-1.91718342555717,1.,-0.449632260106572));
#30285=CARTESIAN_POINT('Ctrl Pts',(-1.91203699981095,1.,-0.446617343485651));
#30286=CARTESIAN_POINT('Ctrl Pts',(-1.90691756144906,1.,-0.44367755684917));
#30287=CARTESIAN_POINT('Ctrl Pts',(-1.90180124389137,1.,-0.44080783370416));
#30288=CARTESIAN_POINT('Ctrl Pts',(-1.89663648956549,1.,-0.437995003948443));
#30289=CARTESIAN_POINT('Ctrl Pts',(-1.89136993975585,1.,-0.43522566096358));
#30290=CARTESIAN_POINT('Ctrl Pts',(-1.88596913666828,1.,-0.432493038548833));
#30291=CARTESIAN_POINT('Ctrl Pts',(-1.88044229001778,1.,-0.429803062482217));
#30292=CARTESIAN_POINT('Ctrl Pts',(-1.87486989291333,1.,-0.427183828518743));
#30293=CARTESIAN_POINT('Ctrl Pts',(-1.8693780394412,1.,-0.424678177290876));
#30294=CARTESIAN_POINT('Ctrl Pts',(-1.86408083333863,1.,-0.422327307417884));
#30295=CARTESIAN_POINT('Ctrl Pts',(-1.8590328109667,1.,-0.420157287975583));
#30296=CARTESIAN_POINT('Ctrl Pts',(-1.8541763285645,1.,-0.418164129144045));
#30297=CARTESIAN_POINT('Ctrl Pts',(-1.84929312930314,1.,-0.416300022039885));
#30298=CARTESIAN_POINT('Ctrl Pts',(-1.84405757074218,1.,-0.414487438255542));
#30299=CARTESIAN_POINT('Ctrl Pts',(-1.8380895347617,1.,-0.412633125322945));
#30300=CARTESIAN_POINT('Ctrl Pts',(-1.83100408895047,1.,-0.410641256301276));
#30301=CARTESIAN_POINT('Ctrl Pts',(-1.82247022677562,1.,-0.408428948106227));
#30302=CARTESIAN_POINT('Ctrl Pts',(-1.81223801812013,1.,-0.405933518407175));
#30303=CARTESIAN_POINT('Ctrl Pts',(-1.80012077173238,1.,-0.403107976163396));
#30304=CARTESIAN_POINT('Ctrl Pts',(-1.78598826343754,1.,-0.399919403774155));
#30305=CARTESIAN_POINT('Ctrl Pts',(-1.76975560043442,1.,-0.396346196110688));
#30306=CARTESIAN_POINT('Ctrl Pts',(-1.75137405310193,1.,-0.392375812285395));
#30307=CARTESIAN_POINT('Ctrl Pts',(-1.73493170972829,1.,-0.388877023502615));
#30308=CARTESIAN_POINT('Ctrl Pts',(-1.72162022244582,1.,-0.386070790323281));
#30309=CARTESIAN_POINT('Ctrl Pts',(-1.71231062891398,1.,-0.384119047314215));
#30310=CARTESIAN_POINT('Ctrl Pts',(-1.7075470150345,1.,-0.383122945602004));
#30311=CARTESIAN_POINT('',(-2.11275013067528,0.,-0.61342227326009));
#30312=CARTESIAN_POINT('Origin',(-2.0698113262342,0.,-0.745574324794401));
#30313=CARTESIAN_POINT('',(-2.0698113262342,1.,-0.745574324794401));
#30314=CARTESIAN_POINT('',(-2.11275013067528,1.,-0.61342227326009));
#30315=CARTESIAN_POINT('',(-2.0698113262342,0.,-0.745574324794401));
#30316=CARTESIAN_POINT('Ctrl Pts',(-1.60662857109684,-1.,-0.693717979106306));
#30317=CARTESIAN_POINT('Ctrl Pts',(-1.60662857109684,1.,-0.693717979106306));
#30318=CARTESIAN_POINT('Ctrl Pts',(-1.61106790958151,-1.,-0.695712097881194));
#30319=CARTESIAN_POINT('Ctrl Pts',(-1.61106790958151,1.,-0.695712097881194));
#30320=CARTESIAN_POINT('Ctrl Pts',(-1.61974673472612,-1.,-0.699605146405088));
#30321=CARTESIAN_POINT('Ctrl Pts',(-1.61974673472612,1.,-0.699605146405088));
#30322=CARTESIAN_POINT('Ctrl Pts',(-1.63216541664676,-1.,-0.705159151988319));
#30323=CARTESIAN_POINT('Ctrl Pts',(-1.63216541664676,1.,-0.705159151988319));
#30324=CARTESIAN_POINT('Ctrl Pts',(-1.64752408832016,-1.,-0.711993139355394));
#30325=CARTESIAN_POINT('Ctrl Pts',(-1.64752408832016,1.,-0.711993139355394));
#30326=CARTESIAN_POINT('Ctrl Pts',(-1.6647288055568,-1.,-0.719585433804282));
#30327=CARTESIAN_POINT('Ctrl Pts',(-1.6647288055568,1.,-0.719585433804282));
#30328=CARTESIAN_POINT('Ctrl Pts',(-1.67996158455503,-1.,-0.726235967997433));
#30329=CARTESIAN_POINT('Ctrl Pts',(-1.67996158455503,1.,-0.726235967997433));
#30330=CARTESIAN_POINT('Ctrl Pts',(-1.69326921975743,-1.,-0.731963238697195));
#30331=CARTESIAN_POINT('Ctrl Pts',(-1.69326921975743,1.,-0.731963238697195));
#30332=CARTESIAN_POINT('Ctrl Pts',(-1.70473309006121,-1.,-0.736799665724771));
#30333=CARTESIAN_POINT('Ctrl Pts',(-1.70473309006121,1.,-0.736799665724771));
#30334=CARTESIAN_POINT('Ctrl Pts',(-1.71447789751927,-1.,-0.740795162032087));
#30335=CARTESIAN_POINT('Ctrl Pts',(-1.71447789751927,1.,-0.740795162032087));
#30336=CARTESIAN_POINT('Ctrl Pts',(-1.7226822991693,-1.,-0.744021445433764));
#30337=CARTESIAN_POINT('Ctrl Pts',(-1.7226822991693,1.,-0.744021445433764));
#30338=CARTESIAN_POINT('Ctrl Pts',(-1.72958533647399,-1.,-0.746574710096436));
#30339=CARTESIAN_POINT('Ctrl Pts',(-1.72958533647399,1.,-0.746574710096436));
#30340=CARTESIAN_POINT('Ctrl Pts',(-1.73550351679848,-1.,-0.748582462954854));
#30341=CARTESIAN_POINT('Ctrl Pts',(-1.73550351679848,1.,-0.748582462954854));
#30342=CARTESIAN_POINT('Ctrl Pts',(-1.74080458266705,-1.,-0.75019343597954));
#30343=CARTESIAN_POINT('Ctrl Pts',(-1.74080458266705,1.,-0.75019343597954));
#30344=CARTESIAN_POINT('Ctrl Pts',(-1.74585086852298,-1.,-0.751555614163629));
#30345=CARTESIAN_POINT('Ctrl Pts',(-1.74585086852298,1.,-0.751555614163629));
#30346=CARTESIAN_POINT('Ctrl Pts',(-1.75095139468809,-1.,-0.752797683531377));
#30347=CARTESIAN_POINT('Ctrl Pts',(-1.75095139468809,1.,-0.752797683531377));
#30348=CARTESIAN_POINT('Ctrl Pts',(-1.75631083600175,-1.,-0.75400925402848));
#30349=CARTESIAN_POINT('Ctrl Pts',(-1.75631083600175,1.,-0.75400925402848));
#30350=CARTESIAN_POINT('Ctrl Pts',(-1.7619781724032,-1.,-0.755220979975262));
#30351=CARTESIAN_POINT('Ctrl Pts',(-1.7619781724032,1.,-0.755220979975262));
#30352=CARTESIAN_POINT('Ctrl Pts',(-1.76789396003141,-1.,-0.756421896028403));
#30353=CARTESIAN_POINT('Ctrl Pts',(-1.76789396003141,1.,-0.756421896028403));
#30354=CARTESIAN_POINT('Ctrl Pts',(-1.77394167108342,-1.,-0.757578264077238));
#30355=CARTESIAN_POINT('Ctrl Pts',(-1.77394167108342,1.,-0.757578264077238));
#30356=CARTESIAN_POINT('Ctrl Pts',(-1.77999411220912,-1.,-0.75865062667738));
#30357=CARTESIAN_POINT('Ctrl Pts',(-1.77999411220912,1.,-0.75865062667738));
#30358=CARTESIAN_POINT('Ctrl Pts',(-1.78596964884526,-1.,-0.759614401109868));
#30359=CARTESIAN_POINT('Ctrl Pts',(-1.78596964884526,1.,-0.759614401109868));
#30360=CARTESIAN_POINT('Ctrl Pts',(-1.79185815610802,-1.,-0.760469555880425));
#30361=CARTESIAN_POINT('Ctrl Pts',(-1.79185815610802,1.,-0.760469555880425));
#30362=CARTESIAN_POINT('Ctrl Pts',(-1.79768986997735,-1.,-0.761229695230359));
#30363=CARTESIAN_POINT('Ctrl Pts',(-1.79768986997735,1.,-0.761229695230359));
#30364=CARTESIAN_POINT('Ctrl Pts',(-1.80351583877334,-1.,-0.761915336443515));
#30365=CARTESIAN_POINT('Ctrl Pts',(-1.80351583877334,1.,-0.761915336443515));
#30366=CARTESIAN_POINT('Ctrl Pts',(-1.80938551463989,-1.,-0.762546129464036));
#30367=CARTESIAN_POINT('Ctrl Pts',(-1.80938551463989,1.,-0.762546129464036));
#30368=CARTESIAN_POINT('Ctrl Pts',(-1.81532118405566,-1.,-0.763132003836783));
#30369=CARTESIAN_POINT('Ctrl Pts',(-1.81532118405566,1.,-0.763132003836783));
#30370=CARTESIAN_POINT('Ctrl Pts',(-1.82131873145297,-1.,-0.763673465462854));
#30371=CARTESIAN_POINT('Ctrl Pts',(-1.82131873145297,1.,-0.763673465462854));
#30372=CARTESIAN_POINT('Ctrl Pts',(-1.8273599120008,-1.,-0.764165902606055));
#30373=CARTESIAN_POINT('Ctrl Pts',(-1.8273599120008,1.,-0.764165902606055));
#30374=CARTESIAN_POINT('Ctrl Pts',(-1.8334207722714,-1.,-0.764602549687845));
#30375=CARTESIAN_POINT('Ctrl Pts',(-1.8334207722714,1.,-0.764602549687845));
#30376=CARTESIAN_POINT('Ctrl Pts',(-1.83948181064823,-1.,-0.764978057881687));
#30377=CARTESIAN_POINT('Ctrl Pts',(-1.83948181064823,1.,-0.764978057881687));
#30378=CARTESIAN_POINT('Ctrl Pts',(-1.8455369887591,-1.,-0.765291664861971));
#30379=CARTESIAN_POINT('Ctrl Pts',(-1.8455369887591,1.,-0.765291664861971));
#30380=CARTESIAN_POINT('Ctrl Pts',(-1.85158945130054,-1.,-0.765545710619023));
#30381=CARTESIAN_POINT('Ctrl Pts',(-1.85158945130054,1.,-0.765545710619023));
#30382=CARTESIAN_POINT('Ctrl Pts',(-1.85764741390391,-1.,-0.765744212909305));
#30383=CARTESIAN_POINT('Ctrl Pts',(-1.85764741390391,1.,-0.765744212909305));
#30384=CARTESIAN_POINT('Ctrl Pts',(-1.86372027063314,-1.,-0.765891519092557));
#30385=CARTESIAN_POINT('Ctrl Pts',(-1.86372027063314,1.,-0.765891519092557));
#30386=CARTESIAN_POINT('Ctrl Pts',(-1.86981398314345,-1.,-0.765990708546111));
#30387=CARTESIAN_POINT('Ctrl Pts',(-1.86981398314345,1.,-0.765990708546111));
#30388=CARTESIAN_POINT('Ctrl Pts',(-1.87592888967886,-1.,-0.766042837036759));
#30389=CARTESIAN_POINT('Ctrl Pts',(-1.87592888967886,1.,-0.766042837036759));
#30390=CARTESIAN_POINT('Ctrl Pts',(-1.88206215302561,-1.,-0.766047794851868));
#30391=CARTESIAN_POINT('Ctrl Pts',(-1.88206215302561,1.,-0.766047794851868));
#30392=CARTESIAN_POINT('Ctrl Pts',(-1.88820926433409,-1.,-0.76600483706209));
#30393=CARTESIAN_POINT('Ctrl Pts',(-1.88820926433409,1.,-0.76600483706209));
#30394=CARTESIAN_POINT('Ctrl Pts',(-1.89436577771389,-1.,-0.765913193856979));
#30395=CARTESIAN_POINT('Ctrl Pts',(-1.89436577771389,1.,-0.765913193856979));
#30396=CARTESIAN_POINT('Ctrl Pts',(-1.90052930393599,-1.,-0.765772772593395));
#30397=CARTESIAN_POINT('Ctrl Pts',(-1.90052930393599,1.,-0.765772772593395));
#30398=CARTESIAN_POINT('Ctrl Pts',(-1.90669961402362,-1.,-0.765584196937936));
#30399=CARTESIAN_POINT('Ctrl Pts',(-1.90669961402362,1.,-0.765584196937936));
#30400=CARTESIAN_POINT('Ctrl Pts',(-1.91287765805174,-1.,-0.765348465884739));
#30401=CARTESIAN_POINT('Ctrl Pts',(-1.91287765805174,1.,-0.765348465884739));
#30402=CARTESIAN_POINT('Ctrl Pts',(-1.91906491634197,-1.,-0.765066729667095));
#30403=CARTESIAN_POINT('Ctrl Pts',(-1.91906491634197,1.,-0.765066729667095));
#30404=CARTESIAN_POINT('Ctrl Pts',(-1.92526263537041,-1.,-0.764740025488189));
#30405=CARTESIAN_POINT('Ctrl Pts',(-1.92526263537041,1.,-0.764740025488189));
#30406=CARTESIAN_POINT('Ctrl Pts',(-1.93147105496367,-1.,-0.764369010673889));
#30407=CARTESIAN_POINT('Ctrl Pts',(-1.93147105496367,1.,-0.764369010673889));
#30408=CARTESIAN_POINT('Ctrl Pts',(-1.93768964875867,-1.,-0.763954049121393));
#30409=CARTESIAN_POINT('Ctrl Pts',(-1.93768964875867,1.,-0.763954049121393));
#30410=CARTESIAN_POINT('Ctrl Pts',(-1.94391746617626,-1.,-0.76349533353858));
#30411=CARTESIAN_POINT('Ctrl Pts',(-1.94391746617626,1.,-0.76349533353858));
#30412=CARTESIAN_POINT('Ctrl Pts',(-1.95015342590025,-1.,-0.762992990878774));
#30413=CARTESIAN_POINT('Ctrl Pts',(-1.95015342590025,1.,-0.762992990878774));
#30414=CARTESIAN_POINT('Ctrl Pts',(-1.95639665309893,-1.,-0.762447203806263));
#30415=CARTESIAN_POINT('Ctrl Pts',(-1.95639665309893,1.,-0.762447203806263));
#30416=CARTESIAN_POINT('Ctrl Pts',(-1.96264672744229,-1.,-0.761858300014575));
#30417=CARTESIAN_POINT('Ctrl Pts',(-1.96264672744229,1.,-0.761858300014575));
#30418=CARTESIAN_POINT('Ctrl Pts',(-1.96890351582545,-1.,-0.761226690483986));
#30419=CARTESIAN_POINT('Ctrl Pts',(-1.96890351582545,1.,-0.761226690483986));
#30420=CARTESIAN_POINT('Ctrl Pts',(-1.97516705321521,-1.,-0.760552825409855));
#30421=CARTESIAN_POINT('Ctrl Pts',(-1.97516705321521,1.,-0.760552825409855));
#30422=CARTESIAN_POINT('Ctrl Pts',(-1.98143741418156,-1.,-0.759837147452135));
#30423=CARTESIAN_POINT('Ctrl Pts',(-1.98143741418156,1.,-0.759837147452135));
#30424=CARTESIAN_POINT('Ctrl Pts',(-1.98771456680806,-1.,-0.759080037802242));
#30425=CARTESIAN_POINT('Ctrl Pts',(-1.98771456680806,1.,-0.759080037802242));
#30426=CARTESIAN_POINT('Ctrl Pts',(-1.9939983109871,-1.,-0.758281796766377));
#30427=CARTESIAN_POINT('Ctrl Pts',(-1.9939983109871,1.,-0.758281796766377));
#30428=CARTESIAN_POINT('Ctrl Pts',(-2.00028834739072,-1.,-0.757442676862341));
#30429=CARTESIAN_POINT('Ctrl Pts',(-2.00028834739072,1.,-0.757442676862341));
#30430=CARTESIAN_POINT('Ctrl Pts',(-2.00658431587682,-1.,-0.756562904646496));
#30431=CARTESIAN_POINT('Ctrl Pts',(-2.00658431587682,1.,-0.756562904646496));
#30432=CARTESIAN_POINT('Ctrl Pts',(-2.01288584328149,-1.,-0.7556427049581));
#30433=CARTESIAN_POINT('Ctrl Pts',(-2.01288584328149,1.,-0.7556427049581));
#30434=CARTESIAN_POINT('Ctrl Pts',(-2.01919259406003,-1.,-0.75468233072352));
#30435=CARTESIAN_POINT('Ctrl Pts',(-2.01919259406003,1.,-0.75468233072352));
#30436=CARTESIAN_POINT('Ctrl Pts',(-2.02550428623587,-1.,-0.753682061113765));
#30437=CARTESIAN_POINT('Ctrl Pts',(-2.02550428623587,1.,-0.753682061113765));
#30438=CARTESIAN_POINT('Ctrl Pts',(-2.03182068456467,-1.,-0.752642180488104));
#30439=CARTESIAN_POINT('Ctrl Pts',(-2.03182068456467,1.,-0.752642180488104));
#30440=CARTESIAN_POINT('Ctrl Pts',(-2.03814160092173,-1.,-0.751562963361383));
#30441=CARTESIAN_POINT('Ctrl Pts',(-2.03814160092173,1.,-0.751562963361383));
#30442=CARTESIAN_POINT('Ctrl Pts',(-2.04446689147754,-1.,-0.750444657874758));
#30443=CARTESIAN_POINT('Ctrl Pts',(-2.04446689147754,1.,-0.750444657874758));
#30444=CARTESIAN_POINT('Ctrl Pts',(-2.05079645591606,-1.,-0.749287468663053));
#30445=CARTESIAN_POINT('Ctrl Pts',(-2.05079645591606,1.,-0.749287468663053));
#30446=CARTESIAN_POINT('Ctrl Pts',(-2.05713023030263,-1.,-0.748091554181101));
#30447=CARTESIAN_POINT('Ctrl Pts',(-2.05713023030263,1.,-0.748091554181101));
#30448=CARTESIAN_POINT('Ctrl Pts',(-2.06220058927162,-1.,-0.747103932785504));
#30449=CARTESIAN_POINT('Ctrl Pts',(-2.06220058927162,1.,-0.747103932785504));
#30450=CARTESIAN_POINT('Ctrl Pts',(-2.06600523016401,-1.,-0.746345871542695));
#30451=CARTESIAN_POINT('Ctrl Pts',(-2.06600523016401,1.,-0.746345871542695));
#30452=CARTESIAN_POINT('Ctrl Pts',(-2.06854248895575,-1.,-0.74583279137781));
#30453=CARTESIAN_POINT('Ctrl Pts',(-2.06854248895575,1.,-0.74583279137781));
#30454=CARTESIAN_POINT('Ctrl Pts',(-2.0698113262342,-1.,-0.745574324794401));
#30455=CARTESIAN_POINT('Ctrl Pts',(-2.0698113262342,1.,-0.745574324794401));
#30456=CARTESIAN_POINT('',(-1.60662857109684,1.,-0.693717979106306));
#30457=CARTESIAN_POINT('Ctrl Pts',(-1.60662857109684,1.,-0.693717979106306));
#30458=CARTESIAN_POINT('Ctrl Pts',(-1.61106790958151,1.,-0.695712097881194));
#30459=CARTESIAN_POINT('Ctrl Pts',(-1.61974673472612,1.,-0.699605146405088));
#30460=CARTESIAN_POINT('Ctrl Pts',(-1.63216541664676,1.,-0.705159151988319));
#30461=CARTESIAN_POINT('Ctrl Pts',(-1.64752408832016,1.,-0.711993139355394));
#30462=CARTESIAN_POINT('Ctrl Pts',(-1.6647288055568,1.,-0.719585433804282));
#30463=CARTESIAN_POINT('Ctrl Pts',(-1.67996158455503,1.,-0.726235967997433));
#30464=CARTESIAN_POINT('Ctrl Pts',(-1.69326921975743,1.,-0.731963238697195));
#30465=CARTESIAN_POINT('Ctrl Pts',(-1.70473309006121,1.,-0.736799665724771));
#30466=CARTESIAN_POINT('Ctrl Pts',(-1.71447789751927,1.,-0.740795162032087));
#30467=CARTESIAN_POINT('Ctrl Pts',(-1.7226822991693,1.,-0.744021445433764));
#30468=CARTESIAN_POINT('Ctrl Pts',(-1.72958533647399,1.,-0.746574710096436));
#30469=CARTESIAN_POINT('Ctrl Pts',(-1.73550351679848,1.,-0.748582462954854));
#30470=CARTESIAN_POINT('Ctrl Pts',(-1.74080458266705,1.,-0.75019343597954));
#30471=CARTESIAN_POINT('Ctrl Pts',(-1.74585086852298,1.,-0.751555614163629));
#30472=CARTESIAN_POINT('Ctrl Pts',(-1.75095139468809,1.,-0.752797683531377));
#30473=CARTESIAN_POINT('Ctrl Pts',(-1.75631083600175,1.,-0.75400925402848));
#30474=CARTESIAN_POINT('Ctrl Pts',(-1.7619781724032,1.,-0.755220979975262));
#30475=CARTESIAN_POINT('Ctrl Pts',(-1.76789396003141,1.,-0.756421896028403));
#30476=CARTESIAN_POINT('Ctrl Pts',(-1.77394167108342,1.,-0.757578264077238));
#30477=CARTESIAN_POINT('Ctrl Pts',(-1.77999411220912,1.,-0.75865062667738));
#30478=CARTESIAN_POINT('Ctrl Pts',(-1.78596964884526,1.,-0.759614401109868));
#30479=CARTESIAN_POINT('Ctrl Pts',(-1.79185815610802,1.,-0.760469555880425));
#30480=CARTESIAN_POINT('Ctrl Pts',(-1.79768986997735,1.,-0.761229695230359));
#30481=CARTESIAN_POINT('Ctrl Pts',(-1.80351583877334,1.,-0.761915336443515));
#30482=CARTESIAN_POINT('Ctrl Pts',(-1.80938551463989,1.,-0.762546129464036));
#30483=CARTESIAN_POINT('Ctrl Pts',(-1.81532118405566,1.,-0.763132003836783));
#30484=CARTESIAN_POINT('Ctrl Pts',(-1.82131873145297,1.,-0.763673465462854));
#30485=CARTESIAN_POINT('Ctrl Pts',(-1.8273599120008,1.,-0.764165902606055));
#30486=CARTESIAN_POINT('Ctrl Pts',(-1.8334207722714,1.,-0.764602549687845));
#30487=CARTESIAN_POINT('Ctrl Pts',(-1.83948181064823,1.,-0.764978057881687));
#30488=CARTESIAN_POINT('Ctrl Pts',(-1.8455369887591,1.,-0.765291664861971));
#30489=CARTESIAN_POINT('Ctrl Pts',(-1.85158945130054,1.,-0.765545710619023));
#30490=CARTESIAN_POINT('Ctrl Pts',(-1.85764741390391,1.,-0.765744212909305));
#30491=CARTESIAN_POINT('Ctrl Pts',(-1.86372027063314,1.,-0.765891519092557));
#30492=CARTESIAN_POINT('Ctrl Pts',(-1.86981398314345,1.,-0.765990708546111));
#30493=CARTESIAN_POINT('Ctrl Pts',(-1.87592888967886,1.,-0.766042837036759));
#30494=CARTESIAN_POINT('Ctrl Pts',(-1.88206215302561,1.,-0.766047794851868));
#30495=CARTESIAN_POINT('Ctrl Pts',(-1.88820926433409,1.,-0.76600483706209));
#30496=CARTESIAN_POINT('Ctrl Pts',(-1.89436577771389,1.,-0.765913193856979));
#30497=CARTESIAN_POINT('Ctrl Pts',(-1.90052930393599,1.,-0.765772772593395));
#30498=CARTESIAN_POINT('Ctrl Pts',(-1.90669961402362,1.,-0.765584196937936));
#30499=CARTESIAN_POINT('Ctrl Pts',(-1.91287765805174,1.,-0.765348465884739));
#30500=CARTESIAN_POINT('Ctrl Pts',(-1.91906491634197,1.,-0.765066729667095));
#30501=CARTESIAN_POINT('Ctrl Pts',(-1.92526263537041,1.,-0.764740025488189));
#30502=CARTESIAN_POINT('Ctrl Pts',(-1.93147105496367,1.,-0.764369010673889));
#30503=CARTESIAN_POINT('Ctrl Pts',(-1.93768964875867,1.,-0.763954049121393));
#30504=CARTESIAN_POINT('Ctrl Pts',(-1.94391746617626,1.,-0.76349533353858));
#30505=CARTESIAN_POINT('Ctrl Pts',(-1.95015342590025,1.,-0.762992990878774));
#30506=CARTESIAN_POINT('Ctrl Pts',(-1.95639665309893,1.,-0.762447203806263));
#30507=CARTESIAN_POINT('Ctrl Pts',(-1.96264672744229,1.,-0.761858300014575));
#30508=CARTESIAN_POINT('Ctrl Pts',(-1.96890351582545,1.,-0.761226690483986));
#30509=CARTESIAN_POINT('Ctrl Pts',(-1.97516705321521,1.,-0.760552825409855));
#30510=CARTESIAN_POINT('Ctrl Pts',(-1.98143741418156,1.,-0.759837147452135));
#30511=CARTESIAN_POINT('Ctrl Pts',(-1.98771456680806,1.,-0.759080037802242));
#30512=CARTESIAN_POINT('Ctrl Pts',(-1.9939983109871,1.,-0.758281796766377));
#30513=CARTESIAN_POINT('Ctrl Pts',(-2.00028834739072,1.,-0.757442676862341));
#30514=CARTESIAN_POINT('Ctrl Pts',(-2.00658431587682,1.,-0.756562904646496));
#30515=CARTESIAN_POINT('Ctrl Pts',(-2.01288584328149,1.,-0.7556427049581));
#30516=CARTESIAN_POINT('Ctrl Pts',(-2.01919259406003,1.,-0.75468233072352));
#30517=CARTESIAN_POINT('Ctrl Pts',(-2.02550428623587,1.,-0.753682061113765));
#30518=CARTESIAN_POINT('Ctrl Pts',(-2.03182068456467,1.,-0.752642180488104));
#30519=CARTESIAN_POINT('Ctrl Pts',(-2.03814160092173,1.,-0.751562963361383));
#30520=CARTESIAN_POINT('Ctrl Pts',(-2.04446689147754,1.,-0.750444657874758));
#30521=CARTESIAN_POINT('Ctrl Pts',(-2.05079645591606,1.,-0.749287468663053));
#30522=CARTESIAN_POINT('Ctrl Pts',(-2.05713023030263,1.,-0.748091554181101));
#30523=CARTESIAN_POINT('Ctrl Pts',(-2.06220058927162,1.,-0.747103932785504));
#30524=CARTESIAN_POINT('Ctrl Pts',(-2.06600523016401,1.,-0.746345871542695));
#30525=CARTESIAN_POINT('Ctrl Pts',(-2.06854248895575,1.,-0.74583279137781));
#30526=CARTESIAN_POINT('Ctrl Pts',(-2.0698113262342,1.,-0.745574324794401));
#30527=CARTESIAN_POINT('',(-1.60662857109684,0.,-0.693717979106306));
#30528=CARTESIAN_POINT('Origin',(0.,0.,0.));
#30529=CARTESIAN_POINT('',(-1.5055822144029,1.,-0.892032620296855));
#30530=CARTESIAN_POINT('Origin',(0.,1.,0.));
#30531=CARTESIAN_POINT('',(-1.5055822144029,0.,-0.892032620296855));
#30532=CARTESIAN_POINT('Ctrl Pts',(-1.81978687191668,-1.,-1.23627494547115));
#30533=CARTESIAN_POINT('Ctrl Pts',(-1.81978687191668,1.,-1.23627494547115));
#30534=CARTESIAN_POINT('Ctrl Pts',(-1.81925017193666,-1.,-1.23509651170476));
#30535=CARTESIAN_POINT('Ctrl Pts',(-1.81925017193666,1.,-1.23509651170476));
#30536=CARTESIAN_POINT('Ctrl Pts',(-1.81817389921279,-1.,-1.2327422452705));
#30537=CARTESIAN_POINT('Ctrl Pts',(-1.81817389921279,1.,-1.2327422452705));
#30538=CARTESIAN_POINT('Ctrl Pts',(-1.8165508718364,-1.,-1.2292186489137));
#30539=CARTESIAN_POINT('Ctrl Pts',(-1.8165508718364,1.,-1.2292186489137));
#30540=CARTESIAN_POINT('Ctrl Pts',(-1.81436959210434,-1.,-1.2245361330495));
#30541=CARTESIAN_POINT('Ctrl Pts',(-1.81436959210434,1.,-1.2245361330495));
#30542=CARTESIAN_POINT('Ctrl Pts',(-1.81161420806656,-1.,-1.21870906103557));
#30543=CARTESIAN_POINT('Ctrl Pts',(-1.81161420806656,1.,-1.21870906103557));
#30544=CARTESIAN_POINT('Ctrl Pts',(-1.80882996917129,-1.,-1.21290815708314));
#30545=CARTESIAN_POINT('Ctrl Pts',(-1.80882996917129,1.,-1.21290815708314));
#30546=CARTESIAN_POINT('Ctrl Pts',(-1.80601678480707,-1.,-1.20713356605475));
#30547=CARTESIAN_POINT('Ctrl Pts',(-1.80601678480707,1.,-1.20713356605475));
#30548=CARTESIAN_POINT('Ctrl Pts',(-1.80317454838603,-1.,-1.20138548938974));
#30549=CARTESIAN_POINT('Ctrl Pts',(-1.80317454838603,1.,-1.20138548938974));
#30550=CARTESIAN_POINT('Ctrl Pts',(-1.80030314369879,-1.,-1.19566418930242));
#30551=CARTESIAN_POINT('Ctrl Pts',(-1.80030314369879,1.,-1.19566418930242));
#30552=CARTESIAN_POINT('Ctrl Pts',(-1.79740245923478,-1.,-1.18996997934445));
#30553=CARTESIAN_POINT('Ctrl Pts',(-1.79740245923478,1.,-1.18996997934445));
#30554=CARTESIAN_POINT('Ctrl Pts',(-1.79447240321515,-1.,-1.18430321697432));
#30555=CARTESIAN_POINT('Ctrl Pts',(-1.79447240321515,1.,-1.18430321697432));
#30556=CARTESIAN_POINT('Ctrl Pts',(-1.79151291552689,-1.,-1.17866429440809));
#30557=CARTESIAN_POINT('Ctrl Pts',(-1.79151291552689,1.,-1.17866429440809));
#30558=CARTESIAN_POINT('Ctrl Pts',(-1.78852398877616,-1.,-1.17305363177328));
#30559=CARTESIAN_POINT('Ctrl Pts',(-1.78852398877616,1.,-1.17305363177328));
#30560=CARTESIAN_POINT('Ctrl Pts',(-1.78550566040443,-1.,-1.16747166312303));
#30561=CARTESIAN_POINT('Ctrl Pts',(-1.78550566040443,1.,-1.16747166312303));
#30562=CARTESIAN_POINT('Ctrl Pts',(-1.78245795881009,-1.,-1.16191881298499));
#30563=CARTESIAN_POINT('Ctrl Pts',(-1.78245795881009,1.,-1.16191881298499));
#30564=CARTESIAN_POINT('Ctrl Pts',(-1.77938085564275,-1.,-1.15639547194698));
#30565=CARTESIAN_POINT('Ctrl Pts',(-1.77938085564275,1.,-1.15639547194698));
#30566=CARTESIAN_POINT('Ctrl Pts',(-1.7762742255701,-1.,-1.15090197841515));
#30567=CARTESIAN_POINT('Ctrl Pts',(-1.7762742255701,1.,-1.15090197841515));
#30568=CARTESIAN_POINT('Ctrl Pts',(-1.77313777896194,-1.,-1.1454385822692));
#30569=CARTESIAN_POINT('Ctrl Pts',(-1.77313777896194,1.,-1.1454385822692));
#30570=CARTESIAN_POINT('Ctrl Pts',(-1.76997111386769,-1.,-1.14000548336975));
#30571=CARTESIAN_POINT('Ctrl Pts',(-1.76997111386769,1.,-1.14000548336975));
#30572=CARTESIAN_POINT('Ctrl Pts',(-1.76677384551862,-1.,-1.1346029180462));
#30573=CARTESIAN_POINT('Ctrl Pts',(-1.76677384551862,1.,-1.1346029180462));
#30574=CARTESIAN_POINT('Ctrl Pts',(-1.7635457196617,-1.,-1.12923123555075));
#30575=CARTESIAN_POINT('Ctrl Pts',(-1.7635457196617,1.,-1.12923123555075));
#30576=CARTESIAN_POINT('Ctrl Pts',(-1.76028671825096,-1.,-1.12389096855086));
#30577=CARTESIAN_POINT('Ctrl Pts',(-1.76028671825096,1.,-1.12389096855086));
#30578=CARTESIAN_POINT('Ctrl Pts',(-1.75699720772105,-1.,-1.11858293216763));
#30579=CARTESIAN_POINT('Ctrl Pts',(-1.75699720772105,1.,-1.11858293216763));
#30580=CARTESIAN_POINT('Ctrl Pts',(-1.7536777209463,-1.,-1.11330807582551));
#30581=CARTESIAN_POINT('Ctrl Pts',(-1.7536777209463,1.,-1.11330807582551));
#30582=CARTESIAN_POINT('Ctrl Pts',(-1.7503286607592,-1.,-1.10806728183007));
#30583=CARTESIAN_POINT('Ctrl Pts',(-1.7503286607592,1.,-1.10806728183007));
#30584=CARTESIAN_POINT('Ctrl Pts',(-1.74695004214923,-1.,-1.10286118991143));
#30585=CARTESIAN_POINT('Ctrl Pts',(-1.74695004214923,1.,-1.10286118991143));
#30586=CARTESIAN_POINT('Ctrl Pts',(-1.74354119236208,-1.,-1.09768999241225));
#30587=CARTESIAN_POINT('Ctrl Pts',(-1.74354119236208,1.,-1.09768999241225));
#30588=CARTESIAN_POINT('Ctrl Pts',(-1.74010053962247,-1.,-1.09255329056493));
#30589=CARTESIAN_POINT('Ctrl Pts',(-1.74010053962247,1.,-1.09255329056493));
#30590=CARTESIAN_POINT('Ctrl Pts',(-1.73662628326091,-1.,-1.08745056285427));
#30591=CARTESIAN_POINT('Ctrl Pts',(-1.73662628326091,1.,-1.08745056285427));
#30592=CARTESIAN_POINT('Ctrl Pts',(-1.73311705663407,-1.,-1.08238162784749));
#30593=CARTESIAN_POINT('Ctrl Pts',(-1.73311705663407,1.,-1.08238162784749));
#30594=CARTESIAN_POINT('Ctrl Pts',(-1.72957248977424,-1.,-1.0773470373727));
#30595=CARTESIAN_POINT('Ctrl Pts',(-1.72957248977424,1.,-1.0773470373727));
#30596=CARTESIAN_POINT('Ctrl Pts',(-1.72599406198488,-1.,-1.07234866990252));
#30597=CARTESIAN_POINT('Ctrl Pts',(-1.72599406198488,1.,-1.07234866990252));
#30598=CARTESIAN_POINT('Ctrl Pts',(-1.72238500928453,-1.,-1.06738966975462));
#30599=CARTESIAN_POINT('Ctrl Pts',(-1.72238500928453,1.,-1.06738966975462));
#30600=CARTESIAN_POINT('Ctrl Pts',(-1.71874858456904,-1.,-1.06247324680647));
#30601=CARTESIAN_POINT('Ctrl Pts',(-1.71874858456904,1.,-1.06247324680647));
#30602=CARTESIAN_POINT('Ctrl Pts',(-1.7150865442702,-1.,-1.05760163192479));
#30603=CARTESIAN_POINT('Ctrl Pts',(-1.7150865442702,1.,-1.05760163192479));
#30604=CARTESIAN_POINT('Ctrl Pts',(-1.71139783543989,-1.,-1.05277517202855));
#30605=CARTESIAN_POINT('Ctrl Pts',(-1.71139783543989,1.,-1.05277517202855));
#30606=CARTESIAN_POINT('Ctrl Pts',(-1.70767646263649,-1.,-1.04799085404995));
#30607=CARTESIAN_POINT('Ctrl Pts',(-1.70767646263649,1.,-1.04799085404995));
#30608=CARTESIAN_POINT('Ctrl Pts',(-1.70391338707982,-1.,-1.04324363334554));
#30609=CARTESIAN_POINT('Ctrl Pts',(-1.70391338707982,1.,-1.04324363334554));
#30610=CARTESIAN_POINT('Ctrl Pts',(-1.70010052930962,-1.,-1.03852922490789));
#30611=CARTESIAN_POINT('Ctrl Pts',(-1.70010052930962,1.,-1.03852922490789));
#30612=CARTESIAN_POINT('Ctrl Pts',(-1.69623414782771,-1.,-1.03384646003588));
#30613=CARTESIAN_POINT('Ctrl Pts',(-1.69623414782771,1.,-1.03384646003588));
#30614=CARTESIAN_POINT('Ctrl Pts',(-1.69231840863458,-1.,-1.02919977579147));
#30615=CARTESIAN_POINT('Ctrl Pts',(-1.69231840863458,1.,-1.02919977579147));
#30616=CARTESIAN_POINT('Ctrl Pts',(-1.68836910178447,-1.,-1.02460180535255));
#30617=CARTESIAN_POINT('Ctrl Pts',(-1.68836910178447,1.,-1.02460180535255));
#30618=CARTESIAN_POINT('Ctrl Pts',(-1.68440578021706,-1.,-1.02006795074201));
#30619=CARTESIAN_POINT('Ctrl Pts',(-1.68440578021706,1.,-1.02006795074201));
#30620=CARTESIAN_POINT('Ctrl Pts',(-1.68044289894798,-1.,-1.01561026162773));
#30621=CARTESIAN_POINT('Ctrl Pts',(-1.68044289894798,1.,-1.01561026162773));
#30622=CARTESIAN_POINT('Ctrl Pts',(-1.67648246776464,-1.,-1.01123236493511));
#30623=CARTESIAN_POINT('Ctrl Pts',(-1.67648246776464,1.,-1.01123236493511));
#30624=CARTESIAN_POINT('Ctrl Pts',(-1.67250335383293,-1.,-1.00692206696414));
#30625=CARTESIAN_POINT('Ctrl Pts',(-1.67250335383293,1.,-1.00692206696414));
#30626=CARTESIAN_POINT('Ctrl Pts',(-1.66846059277303,-1.,-1.00265091003727));
#30627=CARTESIAN_POINT('Ctrl Pts',(-1.66846059277303,1.,-1.00265091003727));
#30628=CARTESIAN_POINT('Ctrl Pts',(-1.66430758030376,-1.,-0.998389654952758));
#30629=CARTESIAN_POINT('Ctrl Pts',(-1.66430758030376,1.,-0.998389654952758));
#30630=CARTESIAN_POINT('Ctrl Pts',(-1.66001553809947,-1.,-0.994121836661306));
#30631=CARTESIAN_POINT('Ctrl Pts',(-1.66001553809947,1.,-0.994121836661306));
#30632=CARTESIAN_POINT('Ctrl Pts',(-1.65559044289699,-1.,-0.989855627854165));
#30633=CARTESIAN_POINT('Ctrl Pts',(-1.65559044289699,1.,-0.989855627854165));
#30634=CARTESIAN_POINT('Ctrl Pts',(-1.65110016612638,-1.,-0.985642622920821));
#30635=CARTESIAN_POINT('Ctrl Pts',(-1.65110016612638,1.,-0.985642622920821));
#30636=CARTESIAN_POINT('Ctrl Pts',(-1.64665139190656,-1.,-0.981562530939489));
#30637=CARTESIAN_POINT('Ctrl Pts',(-1.64665139190656,1.,-0.981562530939489));
#30638=CARTESIAN_POINT('Ctrl Pts',(-1.64233990826687,-1.,-0.977689794119416));
#30639=CARTESIAN_POINT('Ctrl Pts',(-1.64233990826687,1.,-0.977689794119416));
#30640=CARTESIAN_POINT('Ctrl Pts',(-1.63820952658144,-1.,-0.974066058287418));
#30641=CARTESIAN_POINT('Ctrl Pts',(-1.63820952658144,1.,-0.974066058287418));
#30642=CARTESIAN_POINT('Ctrl Pts',(-1.63420665729798,-1.,-0.970669715997509));
#30643=CARTESIAN_POINT('Ctrl Pts',(-1.63420665729798,1.,-0.970669715997509));
#30644=CARTESIAN_POINT('Ctrl Pts',(-1.63013849959461,-1.,-0.967387853230345));
#30645=CARTESIAN_POINT('Ctrl Pts',(-1.63013849959461,1.,-0.967387853230345));
#30646=CARTESIAN_POINT('Ctrl Pts',(-1.62571930670187,-1.,-0.964046107040536));
#30647=CARTESIAN_POINT('Ctrl Pts',(-1.62571930670187,1.,-0.964046107040536));
#30648=CARTESIAN_POINT('Ctrl Pts',(-1.62061638140221,-1.,-0.960438326101729));
#30649=CARTESIAN_POINT('Ctrl Pts',(-1.62061638140221,1.,-0.960438326101729));
#30650=CARTESIAN_POINT('Ctrl Pts',(-1.61449324337085,-1.,-0.956354422920671));
#30651=CARTESIAN_POINT('Ctrl Pts',(-1.61449324337085,1.,-0.956354422920671));
#30652=CARTESIAN_POINT('Ctrl Pts',(-1.60706069896936,-1.,-0.951613284356035));
#30653=CARTESIAN_POINT('Ctrl Pts',(-1.60706069896936,1.,-0.951613284356035));
#30654=CARTESIAN_POINT('Ctrl Pts',(-1.59810042043673,-1.,-0.946078063315257));
#30655=CARTESIAN_POINT('Ctrl Pts',(-1.59810042043673,1.,-0.946078063315257));
#30656=CARTESIAN_POINT('Ctrl Pts',(-1.58744937487176,-1.,-0.939646377893399));
#30657=CARTESIAN_POINT('Ctrl Pts',(-1.58744937487176,1.,-0.939646377893399));
#30658=CARTESIAN_POINT('Ctrl Pts',(-1.57499388382243,-1.,-0.932246680108685));
#30659=CARTESIAN_POINT('Ctrl Pts',(-1.57499388382243,1.,-0.932246680108685));
#30660=CARTESIAN_POINT('Ctrl Pts',(-1.56065988578893,-1.,-0.923832188944341));
#30661=CARTESIAN_POINT('Ctrl Pts',(-1.56065988578893,1.,-0.923832188944341));
#30662=CARTESIAN_POINT('Ctrl Pts',(-1.54440491149498,-1.,-0.914375919026456));
#30663=CARTESIAN_POINT('Ctrl Pts',(-1.54440491149498,1.,-0.914375919026456));
#30664=CARTESIAN_POINT('Ctrl Pts',(-1.52984849887993,-1.,-0.905967409625651));
#30665=CARTESIAN_POINT('Ctrl Pts',(-1.52984849887993,1.,-0.905967409625651));
#30666=CARTESIAN_POINT('Ctrl Pts',(-1.51805569590094,-1.,-0.899185047483511));
#30667=CARTESIAN_POINT('Ctrl Pts',(-1.51805569590094,1.,-0.899185047483511));
#30668=CARTESIAN_POINT('Ctrl Pts',(-1.50980486806688,-1.,-0.894452006964543));
#30669=CARTESIAN_POINT('Ctrl Pts',(-1.50980486806688,1.,-0.894452006964543));
#30670=CARTESIAN_POINT('Ctrl Pts',(-1.5055822144029,-1.,-0.892032620296855));
#30671=CARTESIAN_POINT('Ctrl Pts',(-1.5055822144029,1.,-0.892032620296855));
#30672=CARTESIAN_POINT('',(-1.81978687191668,1.,-1.23627494547115));
#30673=CARTESIAN_POINT('Ctrl Pts',(-1.81978687191668,1.,-1.23627494547115));
#30674=CARTESIAN_POINT('Ctrl Pts',(-1.81925017193666,1.,-1.23509651170476));
#30675=CARTESIAN_POINT('Ctrl Pts',(-1.81817389921279,1.,-1.2327422452705));
#30676=CARTESIAN_POINT('Ctrl Pts',(-1.8165508718364,1.,-1.2292186489137));
#30677=CARTESIAN_POINT('Ctrl Pts',(-1.81436959210434,1.,-1.2245361330495));
#30678=CARTESIAN_POINT('Ctrl Pts',(-1.81161420806656,1.,-1.21870906103557));
#30679=CARTESIAN_POINT('Ctrl Pts',(-1.80882996917129,1.,-1.21290815708314));
#30680=CARTESIAN_POINT('Ctrl Pts',(-1.80601678480707,1.,-1.20713356605475));
#30681=CARTESIAN_POINT('Ctrl Pts',(-1.80317454838603,1.,-1.20138548938974));
#30682=CARTESIAN_POINT('Ctrl Pts',(-1.80030314369879,1.,-1.19566418930242));
#30683=CARTESIAN_POINT('Ctrl Pts',(-1.79740245923478,1.,-1.18996997934445));
#30684=CARTESIAN_POINT('Ctrl Pts',(-1.79447240321515,1.,-1.18430321697432));
#30685=CARTESIAN_POINT('Ctrl Pts',(-1.79151291552689,1.,-1.17866429440809));
#30686=CARTESIAN_POINT('Ctrl Pts',(-1.78852398877616,1.,-1.17305363177328));
#30687=CARTESIAN_POINT('Ctrl Pts',(-1.78550566040443,1.,-1.16747166312303));
#30688=CARTESIAN_POINT('Ctrl Pts',(-1.78245795881009,1.,-1.16191881298499));
#30689=CARTESIAN_POINT('Ctrl Pts',(-1.77938085564275,1.,-1.15639547194698));
#30690=CARTESIAN_POINT('Ctrl Pts',(-1.7762742255701,1.,-1.15090197841515));
#30691=CARTESIAN_POINT('Ctrl Pts',(-1.77313777896194,1.,-1.1454385822692));
#30692=CARTESIAN_POINT('Ctrl Pts',(-1.76997111386769,1.,-1.14000548336975));
#30693=CARTESIAN_POINT('Ctrl Pts',(-1.76677384551862,1.,-1.1346029180462));
#30694=CARTESIAN_POINT('Ctrl Pts',(-1.7635457196617,1.,-1.12923123555075));
#30695=CARTESIAN_POINT('Ctrl Pts',(-1.76028671825096,1.,-1.12389096855086));
#30696=CARTESIAN_POINT('Ctrl Pts',(-1.75699720772105,1.,-1.11858293216763));
#30697=CARTESIAN_POINT('Ctrl Pts',(-1.7536777209463,1.,-1.11330807582551));
#30698=CARTESIAN_POINT('Ctrl Pts',(-1.7503286607592,1.,-1.10806728183007));
#30699=CARTESIAN_POINT('Ctrl Pts',(-1.74695004214923,1.,-1.10286118991143));
#30700=CARTESIAN_POINT('Ctrl Pts',(-1.74354119236208,1.,-1.09768999241225));
#30701=CARTESIAN_POINT('Ctrl Pts',(-1.74010053962247,1.,-1.09255329056493));
#30702=CARTESIAN_POINT('Ctrl Pts',(-1.73662628326091,1.,-1.08745056285427));
#30703=CARTESIAN_POINT('Ctrl Pts',(-1.73311705663407,1.,-1.08238162784749));
#30704=CARTESIAN_POINT('Ctrl Pts',(-1.72957248977424,1.,-1.0773470373727));
#30705=CARTESIAN_POINT('Ctrl Pts',(-1.72599406198488,1.,-1.07234866990252));
#30706=CARTESIAN_POINT('Ctrl Pts',(-1.72238500928453,1.,-1.06738966975462));
#30707=CARTESIAN_POINT('Ctrl Pts',(-1.71874858456904,1.,-1.06247324680647));
#30708=CARTESIAN_POINT('Ctrl Pts',(-1.7150865442702,1.,-1.05760163192479));
#30709=CARTESIAN_POINT('Ctrl Pts',(-1.71139783543989,1.,-1.05277517202855));
#30710=CARTESIAN_POINT('Ctrl Pts',(-1.70767646263649,1.,-1.04799085404995));
#30711=CARTESIAN_POINT('Ctrl Pts',(-1.70391338707982,1.,-1.04324363334554));
#30712=CARTESIAN_POINT('Ctrl Pts',(-1.70010052930962,1.,-1.03852922490789));
#30713=CARTESIAN_POINT('Ctrl Pts',(-1.69623414782771,1.,-1.03384646003588));
#30714=CARTESIAN_POINT('Ctrl Pts',(-1.69231840863458,1.,-1.02919977579147));
#30715=CARTESIAN_POINT('Ctrl Pts',(-1.68836910178447,1.,-1.02460180535255));
#30716=CARTESIAN_POINT('Ctrl Pts',(-1.68440578021706,1.,-1.02006795074201));
#30717=CARTESIAN_POINT('Ctrl Pts',(-1.68044289894798,1.,-1.01561026162773));
#30718=CARTESIAN_POINT('Ctrl Pts',(-1.67648246776464,1.,-1.01123236493511));
#30719=CARTESIAN_POINT('Ctrl Pts',(-1.67250335383293,1.,-1.00692206696414));
#30720=CARTESIAN_POINT('Ctrl Pts',(-1.66846059277303,1.,-1.00265091003727));
#30721=CARTESIAN_POINT('Ctrl Pts',(-1.66430758030376,1.,-0.998389654952758));
#30722=CARTESIAN_POINT('Ctrl Pts',(-1.66001553809947,1.,-0.994121836661306));
#30723=CARTESIAN_POINT('Ctrl Pts',(-1.65559044289699,1.,-0.989855627854165));
#30724=CARTESIAN_POINT('Ctrl Pts',(-1.65110016612638,1.,-0.985642622920821));
#30725=CARTESIAN_POINT('Ctrl Pts',(-1.64665139190656,1.,-0.981562530939489));
#30726=CARTESIAN_POINT('Ctrl Pts',(-1.64233990826687,1.,-0.977689794119416));
#30727=CARTESIAN_POINT('Ctrl Pts',(-1.63820952658144,1.,-0.974066058287418));
#30728=CARTESIAN_POINT('Ctrl Pts',(-1.63420665729798,1.,-0.970669715997509));
#30729=CARTESIAN_POINT('Ctrl Pts',(-1.63013849959461,1.,-0.967387853230345));
#30730=CARTESIAN_POINT('Ctrl Pts',(-1.62571930670187,1.,-0.964046107040536));
#30731=CARTESIAN_POINT('Ctrl Pts',(-1.62061638140221,1.,-0.960438326101729));
#30732=CARTESIAN_POINT('Ctrl Pts',(-1.61449324337085,1.,-0.956354422920671));
#30733=CARTESIAN_POINT('Ctrl Pts',(-1.60706069896936,1.,-0.951613284356035));
#30734=CARTESIAN_POINT('Ctrl Pts',(-1.59810042043673,1.,-0.946078063315257));
#30735=CARTESIAN_POINT('Ctrl Pts',(-1.58744937487176,1.,-0.939646377893399));
#30736=CARTESIAN_POINT('Ctrl Pts',(-1.57499388382243,1.,-0.932246680108685));
#30737=CARTESIAN_POINT('Ctrl Pts',(-1.56065988578893,1.,-0.923832188944341));
#30738=CARTESIAN_POINT('Ctrl Pts',(-1.54440491149498,1.,-0.914375919026456));
#30739=CARTESIAN_POINT('Ctrl Pts',(-1.52984849887993,1.,-0.905967409625651));
#30740=CARTESIAN_POINT('Ctrl Pts',(-1.51805569590094,1.,-0.899185047483511));
#30741=CARTESIAN_POINT('Ctrl Pts',(-1.50980486806688,1.,-0.894452006964543));
#30742=CARTESIAN_POINT('Ctrl Pts',(-1.5055822144029,1.,-0.892032620296855));
#30743=CARTESIAN_POINT('',(-1.81978687191668,0.,-1.23627494547115));
#30744=CARTESIAN_POINT('Origin',(-1.73811241238545,0.,-1.34869019493419));
#30745=CARTESIAN_POINT('',(-1.73811241238545,1.,-1.34869019493419));
#30746=CARTESIAN_POINT('',(-1.81978687191668,1.,-1.23627494547115));
#30747=CARTESIAN_POINT('',(-1.73811241238545,0.,-1.34869019493419));
#30748=CARTESIAN_POINT('Ctrl Pts',(-1.31362392696032,-1.,-1.15624053661742));
#30749=CARTESIAN_POINT('Ctrl Pts',(-1.31362392696032,1.,-1.15624053661742));
#30750=CARTESIAN_POINT('Ctrl Pts',(-1.31722977216397,-1.,-1.15950888730809));
#30751=CARTESIAN_POINT('Ctrl Pts',(-1.31722977216397,1.,-1.15950888730809));
#30752=CARTESIAN_POINT('Ctrl Pts',(-1.32428080721772,-1.,-1.16589330093588));
#30753=CARTESIAN_POINT('Ctrl Pts',(-1.32428080721772,1.,-1.16589330093588));
#30754=CARTESIAN_POINT('Ctrl Pts',(-1.33437539347008,-1.,-1.17501305789857));
#30755=CARTESIAN_POINT('Ctrl Pts',(-1.33437539347008,1.,-1.17501305789857));
#30756=CARTESIAN_POINT('Ctrl Pts',(-1.34687054001093,-1.,-1.18625865667441));
#30757=CARTESIAN_POINT('Ctrl Pts',(-1.34687054001093,1.,-1.18625865667441));
#30758=CARTESIAN_POINT('Ctrl Pts',(-1.36088705043885,-1.,-1.1987959077932));
#30759=CARTESIAN_POINT('Ctrl Pts',(-1.36088705043885,1.,-1.1987959077932));
#30760=CARTESIAN_POINT('Ctrl Pts',(-1.37331915607905,-1.,-1.20982812925645));
#30761=CARTESIAN_POINT('Ctrl Pts',(-1.37331915607905,1.,-1.20982812925645));
#30762=CARTESIAN_POINT('Ctrl Pts',(-1.38420564527715,-1.,-1.21938737280852));
#30763=CARTESIAN_POINT('Ctrl Pts',(-1.38420564527715,1.,-1.21938737280852));
#30764=CARTESIAN_POINT('Ctrl Pts',(-1.39361389568796,-1.,-1.22752961899387));
#30765=CARTESIAN_POINT('Ctrl Pts',(-1.39361389568796,1.,-1.22752961899387));
#30766=CARTESIAN_POINT('Ctrl Pts',(-1.40164708206106,-1.,-1.23434087290423));
#30767=CARTESIAN_POINT('Ctrl Pts',(-1.40164708206106,1.,-1.23434087290423));
#30768=CARTESIAN_POINT('Ctrl Pts',(-1.40845295531283,-1.,-1.23994455029534));
#30769=CARTESIAN_POINT('Ctrl Pts',(-1.40845295531283,1.,-1.23994455029534));
#30770=CARTESIAN_POINT('Ctrl Pts',(-1.41422913175179,-1.,-1.24450600513056));
#30771=CARTESIAN_POINT('Ctrl Pts',(-1.41422913175179,1.,-1.24450600513056));
#30772=CARTESIAN_POINT('Ctrl Pts',(-1.41923722596025,-1.,-1.24824430986571));
#30773=CARTESIAN_POINT('Ctrl Pts',(-1.41923722596025,1.,-1.24824430986571));
#30774=CARTESIAN_POINT('Ctrl Pts',(-1.42378102115575,-1.,-1.2514145557001));
#30775=CARTESIAN_POINT('Ctrl Pts',(-1.42378102115575,1.,-1.2514145557001));
#30776=CARTESIAN_POINT('Ctrl Pts',(-1.42815938799387,-1.,-1.25426945222639));
#30777=CARTESIAN_POINT('Ctrl Pts',(-1.42815938799387,1.,-1.25426945222639));
#30778=CARTESIAN_POINT('Ctrl Pts',(-1.43262645609691,-1.,-1.25702687965755));
#30779=CARTESIAN_POINT('Ctrl Pts',(-1.43262645609691,1.,-1.25702687965755));
#30780=CARTESIAN_POINT('Ctrl Pts',(-1.43734919180848,-1.,-1.25983531012005));
#30781=CARTESIAN_POINT('Ctrl Pts',(-1.43734919180848,1.,-1.25983531012005));
#30782=CARTESIAN_POINT('Ctrl Pts',(-1.44236470511303,-1.,-1.26273903323859));
#30783=CARTESIAN_POINT('Ctrl Pts',(-1.44236470511303,1.,-1.26273903323859));
#30784=CARTESIAN_POINT('Ctrl Pts',(-1.44761985001662,-1.,-1.26570925118868));
#30785=CARTESIAN_POINT('Ctrl Pts',(-1.44761985001662,1.,-1.26570925118868));
#30786=CARTESIAN_POINT('Ctrl Pts',(-1.45301422764247,-1.,-1.2686778680489));
#30787=CARTESIAN_POINT('Ctrl Pts',(-1.45301422764247,1.,-1.2686778680489));
#30788=CARTESIAN_POINT('Ctrl Pts',(-1.45843906294697,-1.,-1.27156805265289));
#30789=CARTESIAN_POINT('Ctrl Pts',(-1.45843906294697,1.,-1.27156805265289));
#30790=CARTESIAN_POINT('Ctrl Pts',(-1.46382431332476,-1.,-1.27433119897822));
#30791=CARTESIAN_POINT('Ctrl Pts',(-1.46382431332476,1.,-1.27433119897822));
#30792=CARTESIAN_POINT('Ctrl Pts',(-1.46916035917133,-1.,-1.27696414831089));
#30793=CARTESIAN_POINT('Ctrl Pts',(-1.46916035917133,1.,-1.27696414831089));
#30794=CARTESIAN_POINT('Ctrl Pts',(-1.4744717526707,-1.,-1.2794891824849));
#30795=CARTESIAN_POINT('Ctrl Pts',(-1.4744717526707,1.,-1.2794891824849));
#30796=CARTESIAN_POINT('Ctrl Pts',(-1.47980070347095,-1.,-1.28194158939517));
#30797=CARTESIAN_POINT('Ctrl Pts',(-1.47980070347095,1.,-1.28194158939517));
#30798=CARTESIAN_POINT('Ctrl Pts',(-1.4851881711891,-1.,-1.28435533880201));
#30799=CARTESIAN_POINT('Ctrl Pts',(-1.4851881711891,1.,-1.28435533880201));
#30800=CARTESIAN_POINT('Ctrl Pts',(-1.4906522831278,-1.,-1.2867467611644));
#30801=CARTESIAN_POINT('Ctrl Pts',(-1.4906522831278,1.,-1.2867467611644));
#30802=CARTESIAN_POINT('Ctrl Pts',(-1.49618896881754,-1.,-1.28911506584254));
#30803=CARTESIAN_POINT('Ctrl Pts',(-1.49618896881754,1.,-1.28911506584254));
#30804=CARTESIAN_POINT('Ctrl Pts',(-1.50178230149776,-1.,-1.29145022885181));
#30805=CARTESIAN_POINT('Ctrl Pts',(-1.50178230149776,1.,-1.29145022885181));
#30806=CARTESIAN_POINT('Ctrl Pts',(-1.50741159078365,-1.,-1.29373841372842));
#30807=CARTESIAN_POINT('Ctrl Pts',(-1.50741159078365,1.,-1.29373841372842));
#30808=CARTESIAN_POINT('Ctrl Pts',(-1.51305994241402,-1.,-1.29596850710509));
#30809=CARTESIAN_POINT('Ctrl Pts',(-1.51305994241402,1.,-1.29596850710509));
#30810=CARTESIAN_POINT('Ctrl Pts',(-1.51872184912724,-1.,-1.29813791800747));
#30811=CARTESIAN_POINT('Ctrl Pts',(-1.51872184912724,1.,-1.29813791800747));
#30812=CARTESIAN_POINT('Ctrl Pts',(-1.52439957861062,-1.,-1.30024984366328));
#30813=CARTESIAN_POINT('Ctrl Pts',(-1.52439957861062,1.,-1.30024984366328));
#30814=CARTESIAN_POINT('Ctrl Pts',(-1.53009970283891,-1.,-1.30231064395568));
#30815=CARTESIAN_POINT('Ctrl Pts',(-1.53009970283891,1.,-1.30231064395568));
#30816=CARTESIAN_POINT('Ctrl Pts',(-1.53582981268977,-1.,-1.30432735639489));
#30817=CARTESIAN_POINT('Ctrl Pts',(-1.53582981268977,1.,-1.30432735639489));
#30818=CARTESIAN_POINT('Ctrl Pts',(-1.54159462645432,-1.,-1.30630475189556));
#30819=CARTESIAN_POINT('Ctrl Pts',(-1.54159462645432,1.,-1.30630475189556));
#30820=CARTESIAN_POINT('Ctrl Pts',(-1.54739413957185,-1.,-1.30824393907473));
#30821=CARTESIAN_POINT('Ctrl Pts',(-1.54739413957185,1.,-1.30824393907473));
#30822=CARTESIAN_POINT('Ctrl Pts',(-1.55322568759481,-1.,-1.31014393684222));
#30823=CARTESIAN_POINT('Ctrl Pts',(-1.55322568759481,1.,-1.31014393684222));
#30824=CARTESIAN_POINT('Ctrl Pts',(-1.55908521254821,-1.,-1.31200264341696));
#30825=CARTESIAN_POINT('Ctrl Pts',(-1.55908521254821,1.,-1.31200264341696));
#30826=CARTESIAN_POINT('Ctrl Pts',(-1.56496872402353,-1.,-1.31381795281002));
#30827=CARTESIAN_POINT('Ctrl Pts',(-1.56496872402353,1.,-1.31381795281002));
#30828=CARTESIAN_POINT('Ctrl Pts',(-1.57087397835723,-1.,-1.31558903860016));
#30829=CARTESIAN_POINT('Ctrl Pts',(-1.57087397835723,1.,-1.31558903860016));
#30830=CARTESIAN_POINT('Ctrl Pts',(-1.5768005650559,-1.,-1.31731642317187));
#30831=CARTESIAN_POINT('Ctrl Pts',(-1.5768005650559,1.,-1.31731642317187));
#30832=CARTESIAN_POINT('Ctrl Pts',(-1.58274907898834,-1.,-1.31900135021432));
#30833=CARTESIAN_POINT('Ctrl Pts',(-1.58274907898834,1.,-1.31900135021432));
#30834=CARTESIAN_POINT('Ctrl Pts',(-1.58872057258245,-1.,-1.32064537110892));
#30835=CARTESIAN_POINT('Ctrl Pts',(-1.58872057258245,1.,-1.32064537110892));
#30836=CARTESIAN_POINT('Ctrl Pts',(-1.59471591079403,-1.,-1.32224985747682));
#30837=CARTESIAN_POINT('Ctrl Pts',(-1.59471591079403,1.,-1.32224985747682));
#30838=CARTESIAN_POINT('Ctrl Pts',(-1.60073511858687,-1.,-1.32381550858256));
#30839=CARTESIAN_POINT('Ctrl Pts',(-1.60073511858687,1.,-1.32381550858256));
#30840=CARTESIAN_POINT('Ctrl Pts',(-1.60677758290954,-1.,-1.32534250785782));
#30841=CARTESIAN_POINT('Ctrl Pts',(-1.60677758290954,1.,-1.32534250785782));
#30842=CARTESIAN_POINT('Ctrl Pts',(-1.6128423401575,-1.,-1.32683074483356));
#30843=CARTESIAN_POINT('Ctrl Pts',(-1.6128423401575,1.,-1.32683074483356));
#30844=CARTESIAN_POINT('Ctrl Pts',(-1.61892832270724,-1.,-1.32828000610449));
#30845=CARTESIAN_POINT('Ctrl Pts',(-1.61892832270724,1.,-1.32828000610449));
#30846=CARTESIAN_POINT('Ctrl Pts',(-1.62503464209797,-1.,-1.3296901950568));
#30847=CARTESIAN_POINT('Ctrl Pts',(-1.62503464209797,1.,-1.3296901950568));
#30848=CARTESIAN_POINT('Ctrl Pts',(-1.63116079730923,-1.,-1.33106149345645));
#30849=CARTESIAN_POINT('Ctrl Pts',(-1.63116079730923,1.,-1.33106149345645));
#30850=CARTESIAN_POINT('Ctrl Pts',(-1.63730653475089,-1.,-1.33239425103724));
#30851=CARTESIAN_POINT('Ctrl Pts',(-1.63730653475089,1.,-1.33239425103724));
#30852=CARTESIAN_POINT('Ctrl Pts',(-1.6434717485603,-1.,-1.33368890676572));
#30853=CARTESIAN_POINT('Ctrl Pts',(-1.6434717485603,1.,-1.33368890676572));
#30854=CARTESIAN_POINT('Ctrl Pts',(-1.6496563728683,-1.,-1.33494590467993));
#30855=CARTESIAN_POINT('Ctrl Pts',(-1.6496563728683,1.,-1.33494590467993));
#30856=CARTESIAN_POINT('Ctrl Pts',(-1.65586025952593,-1.,-1.33616559745172));
#30857=CARTESIAN_POINT('Ctrl Pts',(-1.65586025952593,1.,-1.33616559745172));
#30858=CARTESIAN_POINT('Ctrl Pts',(-1.66208312541983,-1.,-1.33734820885262));
#30859=CARTESIAN_POINT('Ctrl Pts',(-1.66208312541983,1.,-1.33734820885262));
#30860=CARTESIAN_POINT('Ctrl Pts',(-1.66832460783989,-1.,-1.33849388654388));
#30861=CARTESIAN_POINT('Ctrl Pts',(-1.66832460783989,1.,-1.33849388654388));
#30862=CARTESIAN_POINT('Ctrl Pts',(-1.67458429426086,-1.,-1.3396027347034));
#30863=CARTESIAN_POINT('Ctrl Pts',(-1.67458429426086,1.,-1.3396027347034));
#30864=CARTESIAN_POINT('Ctrl Pts',(-1.68086176030362,-1.,-1.34067485185203));
#30865=CARTESIAN_POINT('Ctrl Pts',(-1.68086176030362,1.,-1.34067485185203));
#30866=CARTESIAN_POINT('Ctrl Pts',(-1.68715660868764,-1.,-1.341710374848));
#30867=CARTESIAN_POINT('Ctrl Pts',(-1.68715660868764,1.,-1.341710374848));
#30868=CARTESIAN_POINT('Ctrl Pts',(-1.6934684849687,-1.,-1.34270948206319));
#30869=CARTESIAN_POINT('Ctrl Pts',(-1.6934684849687,1.,-1.34270948206319));
#30870=CARTESIAN_POINT('Ctrl Pts',(-1.69979707754427,-1.,-1.34367237124483));
#30871=CARTESIAN_POINT('Ctrl Pts',(-1.69979707754427,1.,-1.34367237124483));
#30872=CARTESIAN_POINT('Ctrl Pts',(-1.70614212266738,-1.,-1.34459924533831));
#30873=CARTESIAN_POINT('Ctrl Pts',(-1.70614212266738,1.,-1.34459924533831));
#30874=CARTESIAN_POINT('Ctrl Pts',(-1.71250340686822,-1.,-1.34549029589416));
#30875=CARTESIAN_POINT('Ctrl Pts',(-1.71250340686822,1.,-1.34549029589416));
#30876=CARTESIAN_POINT('Ctrl Pts',(-1.7188807715049,-1.,-1.34634568653227));
#30877=CARTESIAN_POINT('Ctrl Pts',(-1.7188807715049,1.,-1.34634568653227));
#30878=CARTESIAN_POINT('Ctrl Pts',(-1.72527410680674,-1.,-1.34716554819527));
#30879=CARTESIAN_POINT('Ctrl Pts',(-1.72527410680674,1.,-1.34716554819527));
#30880=CARTESIAN_POINT('Ctrl Pts',(-1.7304014965394,-1.,-1.34779309152035));
#30881=CARTESIAN_POINT('Ctrl Pts',(-1.7304014965394,1.,-1.34779309152035));
#30882=CARTESIAN_POINT('Ctrl Pts',(-1.73425417885907,-1.,-1.34824783112887));
#30883=CARTESIAN_POINT('Ctrl Pts',(-1.73425417885907,1.,-1.34824783112887));
#30884=CARTESIAN_POINT('Ctrl Pts',(-1.73682580585691,-1.,-1.34854391898045));
#30885=CARTESIAN_POINT('Ctrl Pts',(-1.73682580585691,1.,-1.34854391898045));
#30886=CARTESIAN_POINT('Ctrl Pts',(-1.73811241238545,-1.,-1.34869019493419));
#30887=CARTESIAN_POINT('Ctrl Pts',(-1.73811241238545,1.,-1.34869019493419));
#30888=CARTESIAN_POINT('',(-1.31362392696032,1.,-1.15624053661742));
#30889=CARTESIAN_POINT('Ctrl Pts',(-1.31362392696032,1.,-1.15624053661742));
#30890=CARTESIAN_POINT('Ctrl Pts',(-1.31722977216397,1.,-1.15950888730809));
#30891=CARTESIAN_POINT('Ctrl Pts',(-1.32428080721772,1.,-1.16589330093588));
#30892=CARTESIAN_POINT('Ctrl Pts',(-1.33437539347008,1.,-1.17501305789857));
#30893=CARTESIAN_POINT('Ctrl Pts',(-1.34687054001093,1.,-1.18625865667441));
#30894=CARTESIAN_POINT('Ctrl Pts',(-1.36088705043885,1.,-1.1987959077932));
#30895=CARTESIAN_POINT('Ctrl Pts',(-1.37331915607905,1.,-1.20982812925645));
#30896=CARTESIAN_POINT('Ctrl Pts',(-1.38420564527715,1.,-1.21938737280852));
#30897=CARTESIAN_POINT('Ctrl Pts',(-1.39361389568796,1.,-1.22752961899387));
#30898=CARTESIAN_POINT('Ctrl Pts',(-1.40164708206106,1.,-1.23434087290423));
#30899=CARTESIAN_POINT('Ctrl Pts',(-1.40845295531283,1.,-1.23994455029534));
#30900=CARTESIAN_POINT('Ctrl Pts',(-1.41422913175179,1.,-1.24450600513056));
#30901=CARTESIAN_POINT('Ctrl Pts',(-1.41923722596025,1.,-1.24824430986571));
#30902=CARTESIAN_POINT('Ctrl Pts',(-1.42378102115575,1.,-1.2514145557001));
#30903=CARTESIAN_POINT('Ctrl Pts',(-1.42815938799387,1.,-1.25426945222639));
#30904=CARTESIAN_POINT('Ctrl Pts',(-1.43262645609691,1.,-1.25702687965755));
#30905=CARTESIAN_POINT('Ctrl Pts',(-1.43734919180848,1.,-1.25983531012005));
#30906=CARTESIAN_POINT('Ctrl Pts',(-1.44236470511303,1.,-1.26273903323859));
#30907=CARTESIAN_POINT('Ctrl Pts',(-1.44761985001662,1.,-1.26570925118868));
#30908=CARTESIAN_POINT('Ctrl Pts',(-1.45301422764247,1.,-1.2686778680489));
#30909=CARTESIAN_POINT('Ctrl Pts',(-1.45843906294697,1.,-1.27156805265289));
#30910=CARTESIAN_POINT('Ctrl Pts',(-1.46382431332476,1.,-1.27433119897822));
#30911=CARTESIAN_POINT('Ctrl Pts',(-1.46916035917133,1.,-1.27696414831089));
#30912=CARTESIAN_POINT('Ctrl Pts',(-1.4744717526707,1.,-1.2794891824849));
#30913=CARTESIAN_POINT('Ctrl Pts',(-1.47980070347095,1.,-1.28194158939517));
#30914=CARTESIAN_POINT('Ctrl Pts',(-1.4851881711891,1.,-1.28435533880201));
#30915=CARTESIAN_POINT('Ctrl Pts',(-1.4906522831278,1.,-1.2867467611644));
#30916=CARTESIAN_POINT('Ctrl Pts',(-1.49618896881754,1.,-1.28911506584254));
#30917=CARTESIAN_POINT('Ctrl Pts',(-1.50178230149776,1.,-1.29145022885181));
#30918=CARTESIAN_POINT('Ctrl Pts',(-1.50741159078365,1.,-1.29373841372842));
#30919=CARTESIAN_POINT('Ctrl Pts',(-1.51305994241402,1.,-1.29596850710509));
#30920=CARTESIAN_POINT('Ctrl Pts',(-1.51872184912724,1.,-1.29813791800747));
#30921=CARTESIAN_POINT('Ctrl Pts',(-1.52439957861062,1.,-1.30024984366328));
#30922=CARTESIAN_POINT('Ctrl Pts',(-1.53009970283891,1.,-1.30231064395568));
#30923=CARTESIAN_POINT('Ctrl Pts',(-1.53582981268977,1.,-1.30432735639489));
#30924=CARTESIAN_POINT('Ctrl Pts',(-1.54159462645432,1.,-1.30630475189556));
#30925=CARTESIAN_POINT('Ctrl Pts',(-1.54739413957185,1.,-1.30824393907473));
#30926=CARTESIAN_POINT('Ctrl Pts',(-1.55322568759481,1.,-1.31014393684222));
#30927=CARTESIAN_POINT('Ctrl Pts',(-1.55908521254821,1.,-1.31200264341696));
#30928=CARTESIAN_POINT('Ctrl Pts',(-1.56496872402353,1.,-1.31381795281002));
#30929=CARTESIAN_POINT('Ctrl Pts',(-1.57087397835723,1.,-1.31558903860016));
#30930=CARTESIAN_POINT('Ctrl Pts',(-1.5768005650559,1.,-1.31731642317187));
#30931=CARTESIAN_POINT('Ctrl Pts',(-1.58274907898834,1.,-1.31900135021432));
#30932=CARTESIAN_POINT('Ctrl Pts',(-1.58872057258245,1.,-1.32064537110892));
#30933=CARTESIAN_POINT('Ctrl Pts',(-1.59471591079403,1.,-1.32224985747682));
#30934=CARTESIAN_POINT('Ctrl Pts',(-1.60073511858687,1.,-1.32381550858256));
#30935=CARTESIAN_POINT('Ctrl Pts',(-1.60677758290954,1.,-1.32534250785782));
#30936=CARTESIAN_POINT('Ctrl Pts',(-1.6128423401575,1.,-1.32683074483356));
#30937=CARTESIAN_POINT('Ctrl Pts',(-1.61892832270724,1.,-1.32828000610449));
#30938=CARTESIAN_POINT('Ctrl Pts',(-1.62503464209797,1.,-1.3296901950568));
#30939=CARTESIAN_POINT('Ctrl Pts',(-1.63116079730923,1.,-1.33106149345645));
#30940=CARTESIAN_POINT('Ctrl Pts',(-1.63730653475089,1.,-1.33239425103724));
#30941=CARTESIAN_POINT('Ctrl Pts',(-1.6434717485603,1.,-1.33368890676572));
#30942=CARTESIAN_POINT('Ctrl Pts',(-1.6496563728683,1.,-1.33494590467993));
#30943=CARTESIAN_POINT('Ctrl Pts',(-1.65586025952593,1.,-1.33616559745172));
#30944=CARTESIAN_POINT('Ctrl Pts',(-1.66208312541983,1.,-1.33734820885262));
#30945=CARTESIAN_POINT('Ctrl Pts',(-1.66832460783989,1.,-1.33849388654388));
#30946=CARTESIAN_POINT('Ctrl Pts',(-1.67458429426086,1.,-1.3396027347034));
#30947=CARTESIAN_POINT('Ctrl Pts',(-1.68086176030362,1.,-1.34067485185203));
#30948=CARTESIAN_POINT('Ctrl Pts',(-1.68715660868764,1.,-1.341710374848));
#30949=CARTESIAN_POINT('Ctrl Pts',(-1.6934684849687,1.,-1.34270948206319));
#30950=CARTESIAN_POINT('Ctrl Pts',(-1.69979707754427,1.,-1.34367237124483));
#30951=CARTESIAN_POINT('Ctrl Pts',(-1.70614212266738,1.,-1.34459924533831));
#30952=CARTESIAN_POINT('Ctrl Pts',(-1.71250340686822,1.,-1.34549029589416));
#30953=CARTESIAN_POINT('Ctrl Pts',(-1.7188807715049,1.,-1.34634568653227));
#30954=CARTESIAN_POINT('Ctrl Pts',(-1.72527410680674,1.,-1.34716554819527));
#30955=CARTESIAN_POINT('Ctrl Pts',(-1.7304014965394,1.,-1.34779309152035));
#30956=CARTESIAN_POINT('Ctrl Pts',(-1.73425417885907,1.,-1.34824783112887));
#30957=CARTESIAN_POINT('Ctrl Pts',(-1.73682580585691,1.,-1.34854391898045));
#30958=CARTESIAN_POINT('Ctrl Pts',(-1.73811241238545,1.,-1.34869019493419));
#30959=CARTESIAN_POINT('',(-1.31362392696032,0.,-1.15624053661742));
#30960=CARTESIAN_POINT('Origin',(0.,0.,0.));
#30961=CARTESIAN_POINT('',(-1.15624053661742,1.,-1.31362392696033));
#30962=CARTESIAN_POINT('Origin',(0.,1.,0.));
#30963=CARTESIAN_POINT('',(-1.15624053661742,0.,-1.31362392696033));
#30964=CARTESIAN_POINT('Ctrl Pts',(-1.34869019493419,-1.,-1.73811241238545));
#30965=CARTESIAN_POINT('Ctrl Pts',(-1.34869019493419,1.,-1.73811241238545));
#30966=CARTESIAN_POINT('Ctrl Pts',(-1.34854391898145,-1.,-1.73682580585819));
#30967=CARTESIAN_POINT('Ctrl Pts',(-1.34854391898145,1.,-1.73682580585819));
#30968=CARTESIAN_POINT('Ctrl Pts',(-1.34824783113158,-1.,-1.73425417886255));
#30969=CARTESIAN_POINT('Ctrl Pts',(-1.34824783113158,1.,-1.73425417886255));
#30970=CARTESIAN_POINT('Ctrl Pts',(-1.3477930915247,-1.,-1.73040149654497));
#30971=CARTESIAN_POINT('Ctrl Pts',(-1.3477930915247,1.,-1.73040149654497));
#30972=CARTESIAN_POINT('Ctrl Pts',(-1.34716554820013,-1.,-1.72527410681298));
#30973=CARTESIAN_POINT('Ctrl Pts',(-1.34716554820013,1.,-1.72527410681298));
#30974=CARTESIAN_POINT('Ctrl Pts',(-1.34634568653586,-1.,-1.7188807715095));
#30975=CARTESIAN_POINT('Ctrl Pts',(-1.34634568653586,1.,-1.7188807715095));
#30976=CARTESIAN_POINT('Ctrl Pts',(-1.34549029589563,-1.,-1.71250340687011));
#30977=CARTESIAN_POINT('Ctrl Pts',(-1.34549029589563,1.,-1.71250340687011));
#30978=CARTESIAN_POINT('Ctrl Pts',(-1.34459924533783,-1.,-1.70614212266676));
#30979=CARTESIAN_POINT('Ctrl Pts',(-1.34459924533783,1.,-1.70614212266676));
#30980=CARTESIAN_POINT('Ctrl Pts',(-1.34367237124322,-1.,-1.69979707754221));
#30981=CARTESIAN_POINT('Ctrl Pts',(-1.34367237124322,1.,-1.69979707754221));
#30982=CARTESIAN_POINT('Ctrl Pts',(-1.34270948206139,-1.,-1.6934684849664));
#30983=CARTESIAN_POINT('Ctrl Pts',(-1.34270948206139,1.,-1.6934684849664));
#30984=CARTESIAN_POINT('Ctrl Pts',(-1.34171037484673,-1.,-1.68715660868602));
#30985=CARTESIAN_POINT('Ctrl Pts',(-1.34171037484673,1.,-1.68715660868602));
#30986=CARTESIAN_POINT('Ctrl Pts',(-1.3406748518516,-1.,-1.68086176030308));
#30987=CARTESIAN_POINT('Ctrl Pts',(-1.3406748518516,1.,-1.68086176030308));
#30988=CARTESIAN_POINT('Ctrl Pts',(-1.33960273470372,-1.,-1.67458429426126));
#30989=CARTESIAN_POINT('Ctrl Pts',(-1.33960273470372,1.,-1.67458429426126));
#30990=CARTESIAN_POINT('Ctrl Pts',(-1.33849388654458,-1.,-1.66832460784078));
#30991=CARTESIAN_POINT('Ctrl Pts',(-1.33849388654458,1.,-1.66832460784078));
#30992=CARTESIAN_POINT('Ctrl Pts',(-1.33734820885331,-1.,-1.66208312542073));
#30993=CARTESIAN_POINT('Ctrl Pts',(-1.33734820885331,1.,-1.66208312542073));
#30994=CARTESIAN_POINT('Ctrl Pts',(-1.33616559745217,-1.,-1.65586025952651));
#30995=CARTESIAN_POINT('Ctrl Pts',(-1.33616559745217,1.,-1.65586025952651));
#30996=CARTESIAN_POINT('Ctrl Pts',(-1.33494590468003,-1.,-1.64965637286843));
#30997=CARTESIAN_POINT('Ctrl Pts',(-1.33494590468003,1.,-1.64965637286843));
#30998=CARTESIAN_POINT('Ctrl Pts',(-1.33368890676554,-1.,-1.64347174856007));
#30999=CARTESIAN_POINT('Ctrl Pts',(-1.33368890676554,1.,-1.64347174856007));
#31000=CARTESIAN_POINT('Ctrl Pts',(-1.33239425103694,-1.,-1.6373065347505));
#31001=CARTESIAN_POINT('Ctrl Pts',(-1.33239425103694,1.,-1.6373065347505));
#31002=CARTESIAN_POINT('Ctrl Pts',(-1.33106149345618,-1.,-1.63116079730887));
#31003=CARTESIAN_POINT('Ctrl Pts',(-1.33106149345618,1.,-1.63116079730887));
#31004=CARTESIAN_POINT('Ctrl Pts',(-1.32969019505665,-1.,-1.62503464209777));
#31005=CARTESIAN_POINT('Ctrl Pts',(-1.32969019505665,1.,-1.62503464209777));
#31006=CARTESIAN_POINT('Ctrl Pts',(-1.32828000610448,-1.,-1.61892832270723));
#31007=CARTESIAN_POINT('Ctrl Pts',(-1.32828000610448,1.,-1.61892832270723));
#31008=CARTESIAN_POINT('Ctrl Pts',(-1.32683074483365,-1.,-1.61284234015762));
#31009=CARTESIAN_POINT('Ctrl Pts',(-1.32683074483365,1.,-1.61284234015762));
#31010=CARTESIAN_POINT('Ctrl Pts',(-1.32534250785794,-1.,-1.6067775829097));
#31011=CARTESIAN_POINT('Ctrl Pts',(-1.32534250785794,1.,-1.6067775829097));
#31012=CARTESIAN_POINT('Ctrl Pts',(-1.32381550858266,-1.,-1.600735118587));
#31013=CARTESIAN_POINT('Ctrl Pts',(-1.32381550858266,1.,-1.600735118587));
#31014=CARTESIAN_POINT('Ctrl Pts',(-1.32224985747686,-1.,-1.59471591079408));
#31015=CARTESIAN_POINT('Ctrl Pts',(-1.32224985747686,1.,-1.59471591079408));
#31016=CARTESIAN_POINT('Ctrl Pts',(-1.32064537110891,-1.,-1.58872057258244));
#31017=CARTESIAN_POINT('Ctrl Pts',(-1.32064537110891,1.,-1.58872057258244));
#31018=CARTESIAN_POINT('Ctrl Pts',(-1.31900135021428,-1.,-1.58274907898829));
#31019=CARTESIAN_POINT('Ctrl Pts',(-1.31900135021428,1.,-1.58274907898829));
#31020=CARTESIAN_POINT('Ctrl Pts',(-1.31731642317183,-1.,-1.57680056505585));
#31021=CARTESIAN_POINT('Ctrl Pts',(-1.31731642317183,1.,-1.57680056505585));
#31022=CARTESIAN_POINT('Ctrl Pts',(-1.31558903860015,-1.,-1.57087397835721));
#31023=CARTESIAN_POINT('Ctrl Pts',(-1.31558903860015,1.,-1.57087397835721));
#31024=CARTESIAN_POINT('Ctrl Pts',(-1.31381795281002,-1.,-1.56496872402352));
#31025=CARTESIAN_POINT('Ctrl Pts',(-1.31381795281002,1.,-1.56496872402352));
#31026=CARTESIAN_POINT('Ctrl Pts',(-1.31200264341696,-1.,-1.55908521254822));
#31027=CARTESIAN_POINT('Ctrl Pts',(-1.31200264341696,1.,-1.55908521254822));
#31028=CARTESIAN_POINT('Ctrl Pts',(-1.31014393684221,-1.,-1.55322568759481));
#31029=CARTESIAN_POINT('Ctrl Pts',(-1.31014393684221,1.,-1.55322568759481));
#31030=CARTESIAN_POINT('Ctrl Pts',(-1.30824393907471,-1.,-1.54739413957183));
#31031=CARTESIAN_POINT('Ctrl Pts',(-1.30824393907471,1.,-1.54739413957183));
#31032=CARTESIAN_POINT('Ctrl Pts',(-1.30630475189553,-1.,-1.54159462645428));
#31033=CARTESIAN_POINT('Ctrl Pts',(-1.30630475189553,1.,-1.54159462645428));
#31034=CARTESIAN_POINT('Ctrl Pts',(-1.30432735639487,-1.,-1.53582981268976));
#31035=CARTESIAN_POINT('Ctrl Pts',(-1.30432735639487,1.,-1.53582981268976));
#31036=CARTESIAN_POINT('Ctrl Pts',(-1.3023106439557,-1.,-1.53009970283893));
#31037=CARTESIAN_POINT('Ctrl Pts',(-1.3023106439557,1.,-1.53009970283893));
#31038=CARTESIAN_POINT('Ctrl Pts',(-1.30024984366334,-1.,-1.5243995786107));
#31039=CARTESIAN_POINT('Ctrl Pts',(-1.30024984366334,1.,-1.5243995786107));
#31040=CARTESIAN_POINT('Ctrl Pts',(-1.29813791800757,-1.,-1.51872184912735));
#31041=CARTESIAN_POINT('Ctrl Pts',(-1.29813791800757,1.,-1.51872184912735));
#31042=CARTESIAN_POINT('Ctrl Pts',(-1.29596850710518,-1.,-1.51305994241412));
#31043=CARTESIAN_POINT('Ctrl Pts',(-1.29596850710518,1.,-1.51305994241412));
#31044=CARTESIAN_POINT('Ctrl Pts',(-1.29373841372843,-1.,-1.50741159078367));
#31045=CARTESIAN_POINT('Ctrl Pts',(-1.29373841372843,1.,-1.50741159078367));
#31046=CARTESIAN_POINT('Ctrl Pts',(-1.29145022885171,-1.,-1.50178230149764));
#31047=CARTESIAN_POINT('Ctrl Pts',(-1.29145022885171,1.,-1.50178230149764));
#31048=CARTESIAN_POINT('Ctrl Pts',(-1.28911506584232,-1.,-1.49618896881729));
#31049=CARTESIAN_POINT('Ctrl Pts',(-1.28911506584232,1.,-1.49618896881729));
#31050=CARTESIAN_POINT('Ctrl Pts',(-1.28674676116415,-1.,-1.4906522831275));
#31051=CARTESIAN_POINT('Ctrl Pts',(-1.28674676116415,1.,-1.4906522831275));
#31052=CARTESIAN_POINT('Ctrl Pts',(-1.28435533880184,-1.,-1.48518817118891));
#31053=CARTESIAN_POINT('Ctrl Pts',(-1.28435533880184,1.,-1.48518817118891));
#31054=CARTESIAN_POINT('Ctrl Pts',(-1.28194158939522,-1.,-1.47980070347102));
#31055=CARTESIAN_POINT('Ctrl Pts',(-1.28194158939522,1.,-1.47980070347102));
#31056=CARTESIAN_POINT('Ctrl Pts',(-1.27948918248524,-1.,-1.4744717526711));
#31057=CARTESIAN_POINT('Ctrl Pts',(-1.27948918248524,1.,-1.4744717526711));
#31058=CARTESIAN_POINT('Ctrl Pts',(-1.27696414831144,-1.,-1.46916035917197));
#31059=CARTESIAN_POINT('Ctrl Pts',(-1.27696414831144,1.,-1.46916035917197));
#31060=CARTESIAN_POINT('Ctrl Pts',(-1.27433119897877,-1.,-1.4638243133254));
#31061=CARTESIAN_POINT('Ctrl Pts',(-1.27433119897877,1.,-1.4638243133254));
#31062=CARTESIAN_POINT('Ctrl Pts',(-1.27156805265312,-1.,-1.45843906294725));
#31063=CARTESIAN_POINT('Ctrl Pts',(-1.27156805265312,1.,-1.45843906294725));
#31064=CARTESIAN_POINT('Ctrl Pts',(-1.26867786804854,-1.,-1.45301422764205));
#31065=CARTESIAN_POINT('Ctrl Pts',(-1.26867786804854,1.,-1.45301422764205));
#31066=CARTESIAN_POINT('Ctrl Pts',(-1.26570925118767,-1.,-1.44761985001544));
#31067=CARTESIAN_POINT('Ctrl Pts',(-1.26570925118767,1.,-1.44761985001544));
#31068=CARTESIAN_POINT('Ctrl Pts',(-1.26273903323723,-1.,-1.44236470511145));
#31069=CARTESIAN_POINT('Ctrl Pts',(-1.26273903323723,1.,-1.44236470511145));
#31070=CARTESIAN_POINT('Ctrl Pts',(-1.25983531011894,-1.,-1.43734919180719));
#31071=CARTESIAN_POINT('Ctrl Pts',(-1.25983531011894,1.,-1.43734919180719));
#31072=CARTESIAN_POINT('Ctrl Pts',(-1.25702687965744,-1.,-1.43262645609679));
#31073=CARTESIAN_POINT('Ctrl Pts',(-1.25702687965744,1.,-1.43262645609679));
#31074=CARTESIAN_POINT('Ctrl Pts',(-1.25426945222783,-1.,-1.42815938799555));
#31075=CARTESIAN_POINT('Ctrl Pts',(-1.25426945222783,1.,-1.42815938799555));
#31076=CARTESIAN_POINT('Ctrl Pts',(-1.25141455570299,-1.,-1.42378102115911));
#31077=CARTESIAN_POINT('Ctrl Pts',(-1.25141455570299,1.,-1.42378102115911));
#31078=CARTESIAN_POINT('Ctrl Pts',(-1.24824430986911,-1.,-1.41923722596421));
#31079=CARTESIAN_POINT('Ctrl Pts',(-1.24824430986911,1.,-1.41923722596421));
#31080=CARTESIAN_POINT('Ctrl Pts',(-1.24450600513278,-1.,-1.41422913175437));
#31081=CARTESIAN_POINT('Ctrl Pts',(-1.24450600513278,1.,-1.41422913175437));
#31082=CARTESIAN_POINT('Ctrl Pts',(-1.23994455029421,-1.,-1.40845295531151));
#31083=CARTESIAN_POINT('Ctrl Pts',(-1.23994455029421,1.,-1.40845295531151));
#31084=CARTESIAN_POINT('Ctrl Pts',(-1.23434087289768,-1.,-1.40164708205345));
#31085=CARTESIAN_POINT('Ctrl Pts',(-1.23434087289768,1.,-1.40164708205345));
#31086=CARTESIAN_POINT('Ctrl Pts',(-1.22752961898063,-1.,-1.39361389567257));
#31087=CARTESIAN_POINT('Ctrl Pts',(-1.22752961898063,1.,-1.39361389567257));
#31088=CARTESIAN_POINT('Ctrl Pts',(-1.21938737278853,-1.,-1.38420564525391));
#31089=CARTESIAN_POINT('Ctrl Pts',(-1.21938737278853,1.,-1.38420564525391));
#31090=CARTESIAN_POINT('Ctrl Pts',(-1.20982812923113,-1.,-1.37331915604962));
#31091=CARTESIAN_POINT('Ctrl Pts',(-1.20982812923113,1.,-1.37331915604962));
#31092=CARTESIAN_POINT('Ctrl Pts',(-1.1987959077656,-1.,-1.36088705040677));
#31093=CARTESIAN_POINT('Ctrl Pts',(-1.1987959077656,1.,-1.36088705040677));
#31094=CARTESIAN_POINT('Ctrl Pts',(-1.18625865664915,-1.,-1.34687053998157));
#31095=CARTESIAN_POINT('Ctrl Pts',(-1.18625865664915,1.,-1.34687053998157));
#31096=CARTESIAN_POINT('Ctrl Pts',(-1.17501305787994,-1.,-1.33437539344842));
#31097=CARTESIAN_POINT('Ctrl Pts',(-1.17501305787994,1.,-1.33437539344842));
#31098=CARTESIAN_POINT('Ctrl Pts',(-1.16589330092532,-1.,-1.32428080720544));
#31099=CARTESIAN_POINT('Ctrl Pts',(-1.16589330092532,1.,-1.32428080720544));
#31100=CARTESIAN_POINT('Ctrl Pts',(-1.15950888730433,-1.,-1.3172297721596));
#31101=CARTESIAN_POINT('Ctrl Pts',(-1.15950888730433,1.,-1.3172297721596));
#31102=CARTESIAN_POINT('Ctrl Pts',(-1.15624053661742,-1.,-1.31362392696033));
#31103=CARTESIAN_POINT('Ctrl Pts',(-1.15624053661742,1.,-1.31362392696033));
#31104=CARTESIAN_POINT('',(-1.34869019493419,1.,-1.73811241238545));
#31105=CARTESIAN_POINT('Ctrl Pts',(-1.34869019493419,1.,-1.73811241238545));
#31106=CARTESIAN_POINT('Ctrl Pts',(-1.34854391898145,1.,-1.73682580585819));
#31107=CARTESIAN_POINT('Ctrl Pts',(-1.34824783113158,1.,-1.73425417886255));
#31108=CARTESIAN_POINT('Ctrl Pts',(-1.3477930915247,1.,-1.73040149654497));
#31109=CARTESIAN_POINT('Ctrl Pts',(-1.34716554820013,1.,-1.72527410681298));
#31110=CARTESIAN_POINT('Ctrl Pts',(-1.34634568653586,1.,-1.7188807715095));
#31111=CARTESIAN_POINT('Ctrl Pts',(-1.34549029589563,1.,-1.71250340687011));
#31112=CARTESIAN_POINT('Ctrl Pts',(-1.34459924533783,1.,-1.70614212266676));
#31113=CARTESIAN_POINT('Ctrl Pts',(-1.34367237124322,1.,-1.69979707754221));
#31114=CARTESIAN_POINT('Ctrl Pts',(-1.34270948206139,1.,-1.6934684849664));
#31115=CARTESIAN_POINT('Ctrl Pts',(-1.34171037484673,1.,-1.68715660868602));
#31116=CARTESIAN_POINT('Ctrl Pts',(-1.3406748518516,1.,-1.68086176030308));
#31117=CARTESIAN_POINT('Ctrl Pts',(-1.33960273470372,1.,-1.67458429426126));
#31118=CARTESIAN_POINT('Ctrl Pts',(-1.33849388654458,1.,-1.66832460784078));
#31119=CARTESIAN_POINT('Ctrl Pts',(-1.33734820885331,1.,-1.66208312542073));
#31120=CARTESIAN_POINT('Ctrl Pts',(-1.33616559745217,1.,-1.65586025952651));
#31121=CARTESIAN_POINT('Ctrl Pts',(-1.33494590468003,1.,-1.64965637286843));
#31122=CARTESIAN_POINT('Ctrl Pts',(-1.33368890676554,1.,-1.64347174856007));
#31123=CARTESIAN_POINT('Ctrl Pts',(-1.33239425103694,1.,-1.6373065347505));
#31124=CARTESIAN_POINT('Ctrl Pts',(-1.33106149345618,1.,-1.63116079730887));
#31125=CARTESIAN_POINT('Ctrl Pts',(-1.32969019505665,1.,-1.62503464209777));
#31126=CARTESIAN_POINT('Ctrl Pts',(-1.32828000610448,1.,-1.61892832270723));
#31127=CARTESIAN_POINT('Ctrl Pts',(-1.32683074483365,1.,-1.61284234015762));
#31128=CARTESIAN_POINT('Ctrl Pts',(-1.32534250785794,1.,-1.6067775829097));
#31129=CARTESIAN_POINT('Ctrl Pts',(-1.32381550858266,1.,-1.600735118587));
#31130=CARTESIAN_POINT('Ctrl Pts',(-1.32224985747686,1.,-1.59471591079408));
#31131=CARTESIAN_POINT('Ctrl Pts',(-1.32064537110891,1.,-1.58872057258244));
#31132=CARTESIAN_POINT('Ctrl Pts',(-1.31900135021428,1.,-1.58274907898829));
#31133=CARTESIAN_POINT('Ctrl Pts',(-1.31731642317183,1.,-1.57680056505585));
#31134=CARTESIAN_POINT('Ctrl Pts',(-1.31558903860015,1.,-1.57087397835721));
#31135=CARTESIAN_POINT('Ctrl Pts',(-1.31381795281002,1.,-1.56496872402352));
#31136=CARTESIAN_POINT('Ctrl Pts',(-1.31200264341696,1.,-1.55908521254822));
#31137=CARTESIAN_POINT('Ctrl Pts',(-1.31014393684221,1.,-1.55322568759481));
#31138=CARTESIAN_POINT('Ctrl Pts',(-1.30824393907471,1.,-1.54739413957183));
#31139=CARTESIAN_POINT('Ctrl Pts',(-1.30630475189553,1.,-1.54159462645428));
#31140=CARTESIAN_POINT('Ctrl Pts',(-1.30432735639487,1.,-1.53582981268976));
#31141=CARTESIAN_POINT('Ctrl Pts',(-1.3023106439557,1.,-1.53009970283893));
#31142=CARTESIAN_POINT('Ctrl Pts',(-1.30024984366334,1.,-1.5243995786107));
#31143=CARTESIAN_POINT('Ctrl Pts',(-1.29813791800757,1.,-1.51872184912735));
#31144=CARTESIAN_POINT('Ctrl Pts',(-1.29596850710518,1.,-1.51305994241412));
#31145=CARTESIAN_POINT('Ctrl Pts',(-1.29373841372843,1.,-1.50741159078367));
#31146=CARTESIAN_POINT('Ctrl Pts',(-1.29145022885171,1.,-1.50178230149764));
#31147=CARTESIAN_POINT('Ctrl Pts',(-1.28911506584232,1.,-1.49618896881729));
#31148=CARTESIAN_POINT('Ctrl Pts',(-1.28674676116415,1.,-1.4906522831275));
#31149=CARTESIAN_POINT('Ctrl Pts',(-1.28435533880184,1.,-1.48518817118891));
#31150=CARTESIAN_POINT('Ctrl Pts',(-1.28194158939522,1.,-1.47980070347102));
#31151=CARTESIAN_POINT('Ctrl Pts',(-1.27948918248524,1.,-1.4744717526711));
#31152=CARTESIAN_POINT('Ctrl Pts',(-1.27696414831144,1.,-1.46916035917197));
#31153=CARTESIAN_POINT('Ctrl Pts',(-1.27433119897877,1.,-1.4638243133254));
#31154=CARTESIAN_POINT('Ctrl Pts',(-1.27156805265312,1.,-1.45843906294725));
#31155=CARTESIAN_POINT('Ctrl Pts',(-1.26867786804854,1.,-1.45301422764205));
#31156=CARTESIAN_POINT('Ctrl Pts',(-1.26570925118767,1.,-1.44761985001544));
#31157=CARTESIAN_POINT('Ctrl Pts',(-1.26273903323723,1.,-1.44236470511145));
#31158=CARTESIAN_POINT('Ctrl Pts',(-1.25983531011894,1.,-1.43734919180719));
#31159=CARTESIAN_POINT('Ctrl Pts',(-1.25702687965744,1.,-1.43262645609679));
#31160=CARTESIAN_POINT('Ctrl Pts',(-1.25426945222783,1.,-1.42815938799555));
#31161=CARTESIAN_POINT('Ctrl Pts',(-1.25141455570299,1.,-1.42378102115911));
#31162=CARTESIAN_POINT('Ctrl Pts',(-1.24824430986911,1.,-1.41923722596421));
#31163=CARTESIAN_POINT('Ctrl Pts',(-1.24450600513278,1.,-1.41422913175437));
#31164=CARTESIAN_POINT('Ctrl Pts',(-1.23994455029421,1.,-1.40845295531151));
#31165=CARTESIAN_POINT('Ctrl Pts',(-1.23434087289768,1.,-1.40164708205345));
#31166=CARTESIAN_POINT('Ctrl Pts',(-1.22752961898063,1.,-1.39361389567257));
#31167=CARTESIAN_POINT('Ctrl Pts',(-1.21938737278853,1.,-1.38420564525391));
#31168=CARTESIAN_POINT('Ctrl Pts',(-1.20982812923113,1.,-1.37331915604962));
#31169=CARTESIAN_POINT('Ctrl Pts',(-1.1987959077656,1.,-1.36088705040677));
#31170=CARTESIAN_POINT('Ctrl Pts',(-1.18625865664915,1.,-1.34687053998157));
#31171=CARTESIAN_POINT('Ctrl Pts',(-1.17501305787994,1.,-1.33437539344842));
#31172=CARTESIAN_POINT('Ctrl Pts',(-1.16589330092532,1.,-1.32428080720544));
#31173=CARTESIAN_POINT('Ctrl Pts',(-1.15950888730433,1.,-1.3172297721596));
#31174=CARTESIAN_POINT('Ctrl Pts',(-1.15624053661742,1.,-1.31362392696033));
#31175=CARTESIAN_POINT('',(-1.34869019493419,0.,-1.73811241238545));
#31176=CARTESIAN_POINT('Origin',(-1.23627494547115,0.,-1.81978687191668));
#31177=CARTESIAN_POINT('',(-1.23627494547115,1.,-1.81978687191668));
#31178=CARTESIAN_POINT('',(-1.34869019493419,1.,-1.73811241238545));
#31179=CARTESIAN_POINT('',(-1.23627494547115,0.,-1.81978687191668));
#31180=CARTESIAN_POINT('Ctrl Pts',(-0.892032620296855,-1.,-1.5055822144029));
#31181=CARTESIAN_POINT('Ctrl Pts',(-0.892032620296855,1.,-1.5055822144029));
#31182=CARTESIAN_POINT('Ctrl Pts',(-0.894452006967538,-1.,-1.50980486807181));
#31183=CARTESIAN_POINT('Ctrl Pts',(-0.894452006967538,1.,-1.50980486807181));
#31184=CARTESIAN_POINT('Ctrl Pts',(-0.89918504749193,-1.,-1.51805569591479));
#31185=CARTESIAN_POINT('Ctrl Pts',(-0.89918504749193,1.,-1.51805569591479));
#31186=CARTESIAN_POINT('Ctrl Pts',(-0.905967409640499,-1.,-1.52984849890434));
#31187=CARTESIAN_POINT('Ctrl Pts',(-0.905967409640499,1.,-1.52984849890434));
#31188=CARTESIAN_POINT('Ctrl Pts',(-0.91437591904658,-1.,-1.54440491152808));
#31189=CARTESIAN_POINT('Ctrl Pts',(-0.91437591904658,1.,-1.54440491152808));
#31190=CARTESIAN_POINT('Ctrl Pts',(-0.923832188966322,-1.,-1.56065988582509));
#31191=CARTESIAN_POINT('Ctrl Pts',(-0.923832188966322,1.,-1.56065988582509));
#31192=CARTESIAN_POINT('Ctrl Pts',(-0.932246680128849,-1.,-1.57499388385561));
#31193=CARTESIAN_POINT('Ctrl Pts',(-0.932246680128849,1.,-1.57499388385561));
#31194=CARTESIAN_POINT('Ctrl Pts',(-0.939646377909319,-1.,-1.58744937489796));
#31195=CARTESIAN_POINT('Ctrl Pts',(-0.939646377909319,1.,-1.58744937489796));
#31196=CARTESIAN_POINT('Ctrl Pts',(-0.946078063325796,-1.,-1.59810042045408));
#31197=CARTESIAN_POINT('Ctrl Pts',(-0.946078063325796,1.,-1.59810042045408));
#31198=CARTESIAN_POINT('Ctrl Pts',(-0.951613284361248,-1.,-1.60706069897794));
#31199=CARTESIAN_POINT('Ctrl Pts',(-0.951613284361248,1.,-1.60706069897794));
#31200=CARTESIAN_POINT('Ctrl Pts',(-0.956354422921573,-1.,-1.61449324337233));
#31201=CARTESIAN_POINT('Ctrl Pts',(-0.956354422921573,1.,-1.61449324337233));
#31202=CARTESIAN_POINT('Ctrl Pts',(-0.960438326099958,-1.,-1.62061638139929));
#31203=CARTESIAN_POINT('Ctrl Pts',(-0.960438326099958,1.,-1.62061638139929));
#31204=CARTESIAN_POINT('Ctrl Pts',(-0.964046107037821,-1.,-1.6257193066974));
#31205=CARTESIAN_POINT('Ctrl Pts',(-0.964046107037821,1.,-1.6257193066974));
#31206=CARTESIAN_POINT('Ctrl Pts',(-0.967387853228041,-1.,-1.63013849959083));
#31207=CARTESIAN_POINT('Ctrl Pts',(-0.967387853228041,1.,-1.63013849959083));
#31208=CARTESIAN_POINT('Ctrl Pts',(-0.970669715996356,-1.,-1.63420665729609));
#31209=CARTESIAN_POINT('Ctrl Pts',(-0.970669715996356,1.,-1.63420665729609));
#31210=CARTESIAN_POINT('Ctrl Pts',(-0.974066058287501,-1.,-1.63820952658157));
#31211=CARTESIAN_POINT('Ctrl Pts',(-0.974066058287501,1.,-1.63820952658157));
#31212=CARTESIAN_POINT('Ctrl Pts',(-0.977689794120297,-1.,-1.64233990826831));
#31213=CARTESIAN_POINT('Ctrl Pts',(-0.977689794120297,1.,-1.64233990826831));
#31214=CARTESIAN_POINT('Ctrl Pts',(-0.981562530940574,-1.,-1.64665139190834));
#31215=CARTESIAN_POINT('Ctrl Pts',(-0.981562530940574,1.,-1.64665139190834));
#31216=CARTESIAN_POINT('Ctrl Pts',(-0.985642622921626,-1.,-1.6511001661277));
#31217=CARTESIAN_POINT('Ctrl Pts',(-0.985642622921626,1.,-1.6511001661277));
#31218=CARTESIAN_POINT('Ctrl Pts',(-0.98985562785445,-1.,-1.65559044289746));
#31219=CARTESIAN_POINT('Ctrl Pts',(-0.98985562785445,1.,-1.65559044289746));
#31220=CARTESIAN_POINT('Ctrl Pts',(-0.994121836661116,-1.,-1.66001553809916));
#31221=CARTESIAN_POINT('Ctrl Pts',(-0.994121836661116,1.,-1.66001553809916));
#31222=CARTESIAN_POINT('Ctrl Pts',(-0.998389654952317,-1.,-1.66430758030304));
#31223=CARTESIAN_POINT('Ctrl Pts',(-0.998389654952317,1.,-1.66430758030304));
#31224=CARTESIAN_POINT('Ctrl Pts',(-1.00265091003682,-1.,-1.66846059277231));
#31225=CARTESIAN_POINT('Ctrl Pts',(-1.00265091003682,1.,-1.66846059277231));
#31226=CARTESIAN_POINT('Ctrl Pts',(-1.00692206696387,-1.,-1.67250335383248));
#31227=CARTESIAN_POINT('Ctrl Pts',(-1.00692206696387,1.,-1.67250335383248));
#31228=CARTESIAN_POINT('Ctrl Pts',(-1.01123236493507,-1.,-1.67648246776457));
#31229=CARTESIAN_POINT('Ctrl Pts',(-1.01123236493507,1.,-1.67648246776457));
#31230=CARTESIAN_POINT('Ctrl Pts',(-1.01561026162787,-1.,-1.6804428989482));
#31231=CARTESIAN_POINT('Ctrl Pts',(-1.01561026162787,1.,-1.6804428989482));
#31232=CARTESIAN_POINT('Ctrl Pts',(-1.02006795074222,-1.,-1.68440578021739));
#31233=CARTESIAN_POINT('Ctrl Pts',(-1.02006795074222,1.,-1.68440578021739));
#31234=CARTESIAN_POINT('Ctrl Pts',(-1.02460180535272,-1.,-1.68836910178475));
#31235=CARTESIAN_POINT('Ctrl Pts',(-1.02460180535272,1.,-1.68836910178475));
#31236=CARTESIAN_POINT('Ctrl Pts',(-1.02919977579155,-1.,-1.69231840863471));
#31237=CARTESIAN_POINT('Ctrl Pts',(-1.02919977579155,1.,-1.69231840863471));
#31238=CARTESIAN_POINT('Ctrl Pts',(-1.03384646003587,-1.,-1.69623414782769));
#31239=CARTESIAN_POINT('Ctrl Pts',(-1.03384646003587,1.,-1.69623414782769));
#31240=CARTESIAN_POINT('Ctrl Pts',(-1.03852922490782,-1.,-1.70010052930951));
#31241=CARTESIAN_POINT('Ctrl Pts',(-1.03852922490782,1.,-1.70010052930951));
#31242=CARTESIAN_POINT('Ctrl Pts',(-1.04324363334546,-1.,-1.70391338707969));
#31243=CARTESIAN_POINT('Ctrl Pts',(-1.04324363334546,1.,-1.70391338707969));
#31244=CARTESIAN_POINT('Ctrl Pts',(-1.0479908540499,-1.,-1.70767646263641));
#31245=CARTESIAN_POINT('Ctrl Pts',(-1.0479908540499,1.,-1.70767646263641));
#31246=CARTESIAN_POINT('Ctrl Pts',(-1.05277517202854,-1.,-1.71139783543986));
#31247=CARTESIAN_POINT('Ctrl Pts',(-1.05277517202854,1.,-1.71139783543986));
#31248=CARTESIAN_POINT('Ctrl Pts',(-1.05760163192481,-1.,-1.71508654427022));
#31249=CARTESIAN_POINT('Ctrl Pts',(-1.05760163192481,1.,-1.71508654427022));
#31250=CARTESIAN_POINT('Ctrl Pts',(-1.0624732468065,-1.,-1.71874858456908));
#31251=CARTESIAN_POINT('Ctrl Pts',(-1.0624732468065,1.,-1.71874858456908));
#31252=CARTESIAN_POINT('Ctrl Pts',(-1.06738966975463,-1.,-1.72238500928456));
#31253=CARTESIAN_POINT('Ctrl Pts',(-1.06738966975463,1.,-1.72238500928456));
#31254=CARTESIAN_POINT('Ctrl Pts',(-1.07234866990252,-1.,-1.72599406198489));
#31255=CARTESIAN_POINT('Ctrl Pts',(-1.07234866990252,1.,-1.72599406198489));
#31256=CARTESIAN_POINT('Ctrl Pts',(-1.0773470373727,-1.,-1.72957248977424));
#31257=CARTESIAN_POINT('Ctrl Pts',(-1.0773470373727,1.,-1.72957248977424));
#31258=CARTESIAN_POINT('Ctrl Pts',(-1.08238162784749,-1.,-1.73311705663407));
#31259=CARTESIAN_POINT('Ctrl Pts',(-1.08238162784749,1.,-1.73311705663407));
#31260=CARTESIAN_POINT('Ctrl Pts',(-1.08745056285429,-1.,-1.73662628326093));
#31261=CARTESIAN_POINT('Ctrl Pts',(-1.08745056285429,1.,-1.73662628326093));
#31262=CARTESIAN_POINT('Ctrl Pts',(-1.09255329056496,-1.,-1.74010053962252));
#31263=CARTESIAN_POINT('Ctrl Pts',(-1.09255329056496,1.,-1.74010053962252));
#31264=CARTESIAN_POINT('Ctrl Pts',(-1.09768999241229,-1.,-1.74354119236212));
#31265=CARTESIAN_POINT('Ctrl Pts',(-1.09768999241229,1.,-1.74354119236212));
#31266=CARTESIAN_POINT('Ctrl Pts',(-1.10286118991144,-1.,-1.74695004214924));
#31267=CARTESIAN_POINT('Ctrl Pts',(-1.10286118991144,1.,-1.74695004214924));
#31268=CARTESIAN_POINT('Ctrl Pts',(-1.10806728183003,-1.,-1.75032866075914));
#31269=CARTESIAN_POINT('Ctrl Pts',(-1.10806728183003,1.,-1.75032866075914));
#31270=CARTESIAN_POINT('Ctrl Pts',(-1.11330807582542,-1.,-1.75367772094617));
#31271=CARTESIAN_POINT('Ctrl Pts',(-1.11330807582542,1.,-1.75367772094617));
#31272=CARTESIAN_POINT('Ctrl Pts',(-1.11858293216752,-1.,-1.75699720772089));
#31273=CARTESIAN_POINT('Ctrl Pts',(-1.11858293216752,1.,-1.75699720772089));
#31274=CARTESIAN_POINT('Ctrl Pts',(-1.12389096855078,-1.,-1.76028671825084));
#31275=CARTESIAN_POINT('Ctrl Pts',(-1.12389096855078,1.,-1.76028671825084));
#31276=CARTESIAN_POINT('Ctrl Pts',(-1.12923123555076,-1.,-1.76354571966171));
#31277=CARTESIAN_POINT('Ctrl Pts',(-1.12923123555076,1.,-1.76354571966171));
#31278=CARTESIAN_POINT('Ctrl Pts',(-1.13460291804635,-1.,-1.76677384551883));
#31279=CARTESIAN_POINT('Ctrl Pts',(-1.13460291804635,1.,-1.76677384551883));
#31280=CARTESIAN_POINT('Ctrl Pts',(-1.14000548337,-1.,-1.76997111386806));
#31281=CARTESIAN_POINT('Ctrl Pts',(-1.14000548337,1.,-1.76997111386806));
#31282=CARTESIAN_POINT('Ctrl Pts',(-1.14543858226948,-1.,-1.77313777896234));
#31283=CARTESIAN_POINT('Ctrl Pts',(-1.14543858226948,1.,-1.77313777896234));
#31284=CARTESIAN_POINT('Ctrl Pts',(-1.15090197841531,-1.,-1.77627422557034));
#31285=CARTESIAN_POINT('Ctrl Pts',(-1.15090197841531,1.,-1.77627422557034));
#31286=CARTESIAN_POINT('Ctrl Pts',(-1.15639547194689,-1.,-1.77938085564261));
#31287=CARTESIAN_POINT('Ctrl Pts',(-1.15639547194689,1.,-1.77938085564261));
#31288=CARTESIAN_POINT('Ctrl Pts',(-1.16191881298458,-1.,-1.78245795880949));
#31289=CARTESIAN_POINT('Ctrl Pts',(-1.16191881298458,1.,-1.78245795880949));
#31290=CARTESIAN_POINT('Ctrl Pts',(-1.16747166312239,-1.,-1.78550566040349));
#31291=CARTESIAN_POINT('Ctrl Pts',(-1.16747166312239,1.,-1.78550566040349));
#31292=CARTESIAN_POINT('Ctrl Pts',(-1.17305363177265,-1.,-1.78852398877523));
#31293=CARTESIAN_POINT('Ctrl Pts',(-1.17305363177265,1.,-1.78852398877523));
#31294=CARTESIAN_POINT('Ctrl Pts',(-1.17866429440781,-1.,-1.79151291552646));
#31295=CARTESIAN_POINT('Ctrl Pts',(-1.17866429440781,1.,-1.79151291552646));
#31296=CARTESIAN_POINT('Ctrl Pts',(-1.18430321697471,-1.,-1.79447240321572));
#31297=CARTESIAN_POINT('Ctrl Pts',(-1.18430321697471,1.,-1.79447240321572));
#31298=CARTESIAN_POINT('Ctrl Pts',(-1.1899699793456,-1.,-1.79740245923649));
#31299=CARTESIAN_POINT('Ctrl Pts',(-1.1899699793456,1.,-1.79740245923649));
#31300=CARTESIAN_POINT('Ctrl Pts',(-1.19566418930405,-1.,-1.80030314370121));
#31301=CARTESIAN_POINT('Ctrl Pts',(-1.19566418930405,1.,-1.80030314370121));
#31302=CARTESIAN_POINT('Ctrl Pts',(-1.2013854893912,-1.,-1.8031745483882));
#31303=CARTESIAN_POINT('Ctrl Pts',(-1.2013854893912,1.,-1.8031745483882));
#31304=CARTESIAN_POINT('Ctrl Pts',(-1.20713356605519,-1.,-1.80601678480772));
#31305=CARTESIAN_POINT('Ctrl Pts',(-1.20713356605519,1.,-1.80601678480772));
#31306=CARTESIAN_POINT('Ctrl Pts',(-1.2129081570818,-1.,-1.80882996916931));
#31307=CARTESIAN_POINT('Ctrl Pts',(-1.2129081570818,1.,-1.80882996916931));
#31308=CARTESIAN_POINT('Ctrl Pts',(-1.2187090610323,-1.,-1.81161420806172));
#31309=CARTESIAN_POINT('Ctrl Pts',(-1.2187090610323,1.,-1.81161420806172));
#31310=CARTESIAN_POINT('Ctrl Pts',(-1.22453613304507,-1.,-1.81436959209778));
#31311=CARTESIAN_POINT('Ctrl Pts',(-1.22453613304507,1.,-1.81436959209778));
#31312=CARTESIAN_POINT('Ctrl Pts',(-1.22921864890975,-1.,-1.81655087183054));
#31313=CARTESIAN_POINT('Ctrl Pts',(-1.22921864890975,1.,-1.81655087183054));
#31314=CARTESIAN_POINT('Ctrl Pts',(-1.23274224526804,-1.,-1.81817389920914));
#31315=CARTESIAN_POINT('Ctrl Pts',(-1.23274224526804,1.,-1.81817389920914));
#31316=CARTESIAN_POINT('Ctrl Pts',(-1.23509651170384,-1.,-1.81925017193531));
#31317=CARTESIAN_POINT('Ctrl Pts',(-1.23509651170384,1.,-1.81925017193531));
#31318=CARTESIAN_POINT('Ctrl Pts',(-1.23627494547115,-1.,-1.81978687191668));
#31319=CARTESIAN_POINT('Ctrl Pts',(-1.23627494547115,1.,-1.81978687191668));
#31320=CARTESIAN_POINT('',(-0.892032620296855,1.,-1.5055822144029));
#31321=CARTESIAN_POINT('Ctrl Pts',(-0.892032620296855,1.,-1.5055822144029));
#31322=CARTESIAN_POINT('Ctrl Pts',(-0.894452006967538,1.,-1.50980486807181));
#31323=CARTESIAN_POINT('Ctrl Pts',(-0.89918504749193,1.,-1.51805569591479));
#31324=CARTESIAN_POINT('Ctrl Pts',(-0.905967409640499,1.,-1.52984849890434));
#31325=CARTESIAN_POINT('Ctrl Pts',(-0.91437591904658,1.,-1.54440491152808));
#31326=CARTESIAN_POINT('Ctrl Pts',(-0.923832188966322,1.,-1.56065988582509));
#31327=CARTESIAN_POINT('Ctrl Pts',(-0.932246680128849,1.,-1.57499388385561));
#31328=CARTESIAN_POINT('Ctrl Pts',(-0.939646377909319,1.,-1.58744937489796));
#31329=CARTESIAN_POINT('Ctrl Pts',(-0.946078063325796,1.,-1.59810042045408));
#31330=CARTESIAN_POINT('Ctrl Pts',(-0.951613284361248,1.,-1.60706069897794));
#31331=CARTESIAN_POINT('Ctrl Pts',(-0.956354422921573,1.,-1.61449324337233));
#31332=CARTESIAN_POINT('Ctrl Pts',(-0.960438326099958,1.,-1.62061638139929));
#31333=CARTESIAN_POINT('Ctrl Pts',(-0.964046107037821,1.,-1.6257193066974));
#31334=CARTESIAN_POINT('Ctrl Pts',(-0.967387853228041,1.,-1.63013849959083));
#31335=CARTESIAN_POINT('Ctrl Pts',(-0.970669715996356,1.,-1.63420665729609));
#31336=CARTESIAN_POINT('Ctrl Pts',(-0.974066058287501,1.,-1.63820952658157));
#31337=CARTESIAN_POINT('Ctrl Pts',(-0.977689794120297,1.,-1.64233990826831));
#31338=CARTESIAN_POINT('Ctrl Pts',(-0.981562530940574,1.,-1.64665139190834));
#31339=CARTESIAN_POINT('Ctrl Pts',(-0.985642622921626,1.,-1.6511001661277));
#31340=CARTESIAN_POINT('Ctrl Pts',(-0.98985562785445,1.,-1.65559044289746));
#31341=CARTESIAN_POINT('Ctrl Pts',(-0.994121836661116,1.,-1.66001553809916));
#31342=CARTESIAN_POINT('Ctrl Pts',(-0.998389654952317,1.,-1.66430758030304));
#31343=CARTESIAN_POINT('Ctrl Pts',(-1.00265091003682,1.,-1.66846059277231));
#31344=CARTESIAN_POINT('Ctrl Pts',(-1.00692206696387,1.,-1.67250335383248));
#31345=CARTESIAN_POINT('Ctrl Pts',(-1.01123236493507,1.,-1.67648246776457));
#31346=CARTESIAN_POINT('Ctrl Pts',(-1.01561026162787,1.,-1.6804428989482));
#31347=CARTESIAN_POINT('Ctrl Pts',(-1.02006795074222,1.,-1.68440578021739));
#31348=CARTESIAN_POINT('Ctrl Pts',(-1.02460180535272,1.,-1.68836910178475));
#31349=CARTESIAN_POINT('Ctrl Pts',(-1.02919977579155,1.,-1.69231840863471));
#31350=CARTESIAN_POINT('Ctrl Pts',(-1.03384646003587,1.,-1.69623414782769));
#31351=CARTESIAN_POINT('Ctrl Pts',(-1.03852922490782,1.,-1.70010052930951));
#31352=CARTESIAN_POINT('Ctrl Pts',(-1.04324363334546,1.,-1.70391338707969));
#31353=CARTESIAN_POINT('Ctrl Pts',(-1.0479908540499,1.,-1.70767646263641));
#31354=CARTESIAN_POINT('Ctrl Pts',(-1.05277517202854,1.,-1.71139783543986));
#31355=CARTESIAN_POINT('Ctrl Pts',(-1.05760163192481,1.,-1.71508654427022));
#31356=CARTESIAN_POINT('Ctrl Pts',(-1.0624732468065,1.,-1.71874858456908));
#31357=CARTESIAN_POINT('Ctrl Pts',(-1.06738966975463,1.,-1.72238500928456));
#31358=CARTESIAN_POINT('Ctrl Pts',(-1.07234866990252,1.,-1.72599406198489));
#31359=CARTESIAN_POINT('Ctrl Pts',(-1.0773470373727,1.,-1.72957248977424));
#31360=CARTESIAN_POINT('Ctrl Pts',(-1.08238162784749,1.,-1.73311705663407));
#31361=CARTESIAN_POINT('Ctrl Pts',(-1.08745056285429,1.,-1.73662628326093));
#31362=CARTESIAN_POINT('Ctrl Pts',(-1.09255329056496,1.,-1.74010053962252));
#31363=CARTESIAN_POINT('Ctrl Pts',(-1.09768999241229,1.,-1.74354119236212));
#31364=CARTESIAN_POINT('Ctrl Pts',(-1.10286118991144,1.,-1.74695004214924));
#31365=CARTESIAN_POINT('Ctrl Pts',(-1.10806728183003,1.,-1.75032866075914));
#31366=CARTESIAN_POINT('Ctrl Pts',(-1.11330807582542,1.,-1.75367772094617));
#31367=CARTESIAN_POINT('Ctrl Pts',(-1.11858293216752,1.,-1.75699720772089));
#31368=CARTESIAN_POINT('Ctrl Pts',(-1.12389096855078,1.,-1.76028671825084));
#31369=CARTESIAN_POINT('Ctrl Pts',(-1.12923123555076,1.,-1.76354571966171));
#31370=CARTESIAN_POINT('Ctrl Pts',(-1.13460291804635,1.,-1.76677384551883));
#31371=CARTESIAN_POINT('Ctrl Pts',(-1.14000548337,1.,-1.76997111386806));
#31372=CARTESIAN_POINT('Ctrl Pts',(-1.14543858226948,1.,-1.77313777896234));
#31373=CARTESIAN_POINT('Ctrl Pts',(-1.15090197841531,1.,-1.77627422557034));
#31374=CARTESIAN_POINT('Ctrl Pts',(-1.15639547194689,1.,-1.77938085564261));
#31375=CARTESIAN_POINT('Ctrl Pts',(-1.16191881298458,1.,-1.78245795880949));
#31376=CARTESIAN_POINT('Ctrl Pts',(-1.16747166312239,1.,-1.78550566040349));
#31377=CARTESIAN_POINT('Ctrl Pts',(-1.17305363177265,1.,-1.78852398877523));
#31378=CARTESIAN_POINT('Ctrl Pts',(-1.17866429440781,1.,-1.79151291552646));
#31379=CARTESIAN_POINT('Ctrl Pts',(-1.18430321697471,1.,-1.79447240321572));
#31380=CARTESIAN_POINT('Ctrl Pts',(-1.1899699793456,1.,-1.79740245923649));
#31381=CARTESIAN_POINT('Ctrl Pts',(-1.19566418930405,1.,-1.80030314370121));
#31382=CARTESIAN_POINT('Ctrl Pts',(-1.2013854893912,1.,-1.8031745483882));
#31383=CARTESIAN_POINT('Ctrl Pts',(-1.20713356605519,1.,-1.80601678480772));
#31384=CARTESIAN_POINT('Ctrl Pts',(-1.2129081570818,1.,-1.80882996916931));
#31385=CARTESIAN_POINT('Ctrl Pts',(-1.2187090610323,1.,-1.81161420806172));
#31386=CARTESIAN_POINT('Ctrl Pts',(-1.22453613304507,1.,-1.81436959209778));
#31387=CARTESIAN_POINT('Ctrl Pts',(-1.22921864890975,1.,-1.81655087183054));
#31388=CARTESIAN_POINT('Ctrl Pts',(-1.23274224526804,1.,-1.81817389920914));
#31389=CARTESIAN_POINT('Ctrl Pts',(-1.23509651170384,1.,-1.81925017193531));
#31390=CARTESIAN_POINT('Ctrl Pts',(-1.23627494547115,1.,-1.81978687191668));
#31391=CARTESIAN_POINT('',(-0.892032620296856,0.,-1.5055822144029));
#31392=CARTESIAN_POINT('Origin',(0.,0.,0.));
#31393=CARTESIAN_POINT('',(-0.693717979106305,1.,-1.60662857109684));
#31394=CARTESIAN_POINT('Origin',(0.,1.,0.));
#31395=CARTESIAN_POINT('',(-0.693717979106306,0.,-1.60662857109684));
#31396=CARTESIAN_POINT('Ctrl Pts',(-0.745574324794401,-1.,-2.0698113262342));
#31397=CARTESIAN_POINT('Ctrl Pts',(-0.745574324794401,1.,-2.0698113262342));
#31398=CARTESIAN_POINT('Ctrl Pts',(-0.745832791378367,-1.,-2.06854248895728));
#31399=CARTESIAN_POINT('Ctrl Pts',(-0.745832791378367,1.,-2.06854248895728));
#31400=CARTESIAN_POINT('Ctrl Pts',(-0.7463458715442,-1.,-2.06600523016815));
#31401=CARTESIAN_POINT('Ctrl Pts',(-0.7463458715442,1.,-2.06600523016815));
#31402=CARTESIAN_POINT('Ctrl Pts',(-0.747103932787919,-1.,-2.06220058927826));
#31403=CARTESIAN_POINT('Ctrl Pts',(-0.747103932787919,1.,-2.06220058927826));
#31404=CARTESIAN_POINT('Ctrl Pts',(-0.748091554183802,-1.,-2.05713023031006));
#31405=CARTESIAN_POINT('Ctrl Pts',(-0.748091554183802,1.,-2.05713023031006));
#31406=CARTESIAN_POINT('Ctrl Pts',(-0.749287468665046,-1.,-2.05079645592154));
#31407=CARTESIAN_POINT('Ctrl Pts',(-0.749287468665046,1.,-2.05079645592154));
#31408=CARTESIAN_POINT('Ctrl Pts',(-0.750444657875576,-1.,-2.04446689147979));
#31409=CARTESIAN_POINT('Ctrl Pts',(-0.750444657875576,1.,-2.04446689147979));
#31410=CARTESIAN_POINT('Ctrl Pts',(-0.751562963361115,-1.,-2.03814160092099));
#31411=CARTESIAN_POINT('Ctrl Pts',(-0.751562963361115,1.,-2.03814160092099));
#31412=CARTESIAN_POINT('Ctrl Pts',(-0.752642180487211,-1.,-2.03182068456221));
#31413=CARTESIAN_POINT('Ctrl Pts',(-0.752642180487211,1.,-2.03182068456221));
#31414=CARTESIAN_POINT('Ctrl Pts',(-0.753682061112768,-1.,-2.02550428623313));
#31415=CARTESIAN_POINT('Ctrl Pts',(-0.753682061112768,1.,-2.02550428623313));
#31416=CARTESIAN_POINT('Ctrl Pts',(-0.754682330722816,-1.,-2.01919259405809));
#31417=CARTESIAN_POINT('Ctrl Pts',(-0.754682330722816,1.,-2.01919259405809));
#31418=CARTESIAN_POINT('Ctrl Pts',(-0.755642704957865,-1.,-2.01288584328084));
#31419=CARTESIAN_POINT('Ctrl Pts',(-0.755642704957865,1.,-2.01288584328084));
#31420=CARTESIAN_POINT('Ctrl Pts',(-0.75656290464667,-1.,-2.0065843158773));
#31421=CARTESIAN_POINT('Ctrl Pts',(-0.75656290464667,1.,-2.0065843158773));
#31422=CARTESIAN_POINT('Ctrl Pts',(-0.757442676862724,-1.,-2.00028834739178));
#31423=CARTESIAN_POINT('Ctrl Pts',(-0.757442676862724,1.,-2.00028834739178));
#31424=CARTESIAN_POINT('Ctrl Pts',(-0.758281796766761,-1.,-1.99399831098817));
#31425=CARTESIAN_POINT('Ctrl Pts',(-0.758281796766761,1.,-1.99399831098817));
#31426=CARTESIAN_POINT('Ctrl Pts',(-0.759080037802488,-1.,-1.98771456680874));
#31427=CARTESIAN_POINT('Ctrl Pts',(-0.759080037802488,1.,-1.98771456680874));
#31428=CARTESIAN_POINT('Ctrl Pts',(-0.75983714745219,-1.,-1.98143741418172));
#31429=CARTESIAN_POINT('Ctrl Pts',(-0.75983714745219,1.,-1.98143741418172));
#31430=CARTESIAN_POINT('Ctrl Pts',(-0.760552825409757,-1.,-1.97516705321494));
#31431=CARTESIAN_POINT('Ctrl Pts',(-0.760552825409757,1.,-1.97516705321494));
#31432=CARTESIAN_POINT('Ctrl Pts',(-0.76122669048382,-1.,-1.96890351582499));
#31433=CARTESIAN_POINT('Ctrl Pts',(-0.76122669048382,1.,-1.96890351582499));
#31434=CARTESIAN_POINT('Ctrl Pts',(-0.761858300014423,-1.,-1.96264672744186));
#31435=CARTESIAN_POINT('Ctrl Pts',(-0.761858300014423,1.,-1.96264672744186));
#31436=CARTESIAN_POINT('Ctrl Pts',(-0.762447203806179,-1.,-1.95639665309869));
#31437=CARTESIAN_POINT('Ctrl Pts',(-0.762447203806179,1.,-1.95639665309869));
#31438=CARTESIAN_POINT('Ctrl Pts',(-0.762992990878769,-1.,-1.95015342590024));
#31439=CARTESIAN_POINT('Ctrl Pts',(-0.762992990878769,1.,-1.95015342590024));
#31440=CARTESIAN_POINT('Ctrl Pts',(-0.763495333538629,-1.,-1.9439174661764));
#31441=CARTESIAN_POINT('Ctrl Pts',(-0.763495333538629,1.,-1.9439174661764));
#31442=CARTESIAN_POINT('Ctrl Pts',(-0.763954049121458,-1.,-1.93768964875886));
#31443=CARTESIAN_POINT('Ctrl Pts',(-0.763954049121458,1.,-1.93768964875886));
#31444=CARTESIAN_POINT('Ctrl Pts',(-0.764369010673941,-1.,-1.93147105496382));
#31445=CARTESIAN_POINT('Ctrl Pts',(-0.764369010673941,1.,-1.93147105496382));
#31446=CARTESIAN_POINT('Ctrl Pts',(-0.764740025488211,-1.,-1.92526263537048));
#31447=CARTESIAN_POINT('Ctrl Pts',(-0.764740025488211,1.,-1.92526263537048));
#31448=CARTESIAN_POINT('Ctrl Pts',(-0.765066729667088,-1.,-1.91906491634196));
#31449=CARTESIAN_POINT('Ctrl Pts',(-0.765066729667088,1.,-1.91906491634196));
#31450=CARTESIAN_POINT('Ctrl Pts',(-0.765348465884722,-1.,-1.91287765805169));
#31451=CARTESIAN_POINT('Ctrl Pts',(-0.765348465884722,1.,-1.91287765805169));
#31452=CARTESIAN_POINT('Ctrl Pts',(-0.765584196937919,-1.,-1.90669961402356));
#31453=CARTESIAN_POINT('Ctrl Pts',(-0.765584196937919,1.,-1.90669961402356));
#31454=CARTESIAN_POINT('Ctrl Pts',(-0.765772772593386,-1.,-1.90052930393596));
#31455=CARTESIAN_POINT('Ctrl Pts',(-0.765772772593386,1.,-1.90052930393596));
#31456=CARTESIAN_POINT('Ctrl Pts',(-0.765913193856978,-1.,-1.89436577771388));
#31457=CARTESIAN_POINT('Ctrl Pts',(-0.765913193856978,1.,-1.89436577771388));
#31458=CARTESIAN_POINT('Ctrl Pts',(-0.766004837062091,-1.,-1.88820926433409));
#31459=CARTESIAN_POINT('Ctrl Pts',(-0.766004837062091,1.,-1.88820926433409));
#31460=CARTESIAN_POINT('Ctrl Pts',(-0.766047794851865,-1.,-1.88206215302561));
#31461=CARTESIAN_POINT('Ctrl Pts',(-0.766047794851865,1.,-1.88206215302561));
#31462=CARTESIAN_POINT('Ctrl Pts',(-0.766042837036744,-1.,-1.87592888967883));
#31463=CARTESIAN_POINT('Ctrl Pts',(-0.766042837036744,1.,-1.87592888967883));
#31464=CARTESIAN_POINT('Ctrl Pts',(-0.765990708546091,-1.,-1.86981398314341));
#31465=CARTESIAN_POINT('Ctrl Pts',(-0.765990708546091,1.,-1.86981398314341));
#31466=CARTESIAN_POINT('Ctrl Pts',(-0.765891519092547,-1.,-1.86372027063312));
#31467=CARTESIAN_POINT('Ctrl Pts',(-0.765891519092547,1.,-1.86372027063312));
#31468=CARTESIAN_POINT('Ctrl Pts',(-0.765744212909318,-1.,-1.85764741390394));
#31469=CARTESIAN_POINT('Ctrl Pts',(-0.765744212909318,1.,-1.85764741390394));
#31470=CARTESIAN_POINT('Ctrl Pts',(-0.765545710619062,-1.,-1.85158945130063));
#31471=CARTESIAN_POINT('Ctrl Pts',(-0.765545710619062,1.,-1.85158945130063));
#31472=CARTESIAN_POINT('Ctrl Pts',(-0.765291664862029,-1.,-1.84553698875924));
#31473=CARTESIAN_POINT('Ctrl Pts',(-0.765291664862029,1.,-1.84553698875924));
#31474=CARTESIAN_POINT('Ctrl Pts',(-0.764978057881737,-1.,-1.83948181064835));
#31475=CARTESIAN_POINT('Ctrl Pts',(-0.764978057881737,1.,-1.83948181064835));
#31476=CARTESIAN_POINT('Ctrl Pts',(-0.764602549687853,-1.,-1.83342077227142));
#31477=CARTESIAN_POINT('Ctrl Pts',(-0.764602549687853,1.,-1.83342077227142));
#31478=CARTESIAN_POINT('Ctrl Pts',(-0.764165902605995,-1.,-1.82735991200065));
#31479=CARTESIAN_POINT('Ctrl Pts',(-0.764165902605995,1.,-1.82735991200065));
#31480=CARTESIAN_POINT('Ctrl Pts',(-0.763673465462726,-1.,-1.82131873145266));
#31481=CARTESIAN_POINT('Ctrl Pts',(-0.763673465462726,1.,-1.82131873145266));
#31482=CARTESIAN_POINT('Ctrl Pts',(-0.763132003836634,-1.,-1.8153211840553));
#31483=CARTESIAN_POINT('Ctrl Pts',(-0.763132003836634,1.,-1.8153211840553));
#31484=CARTESIAN_POINT('Ctrl Pts',(-0.762546129463938,-1.,-1.80938551463965));
#31485=CARTESIAN_POINT('Ctrl Pts',(-0.762546129463938,1.,-1.80938551463965));
#31486=CARTESIAN_POINT('Ctrl Pts',(-0.761915336443547,-1.,-1.80351583877342));
#31487=CARTESIAN_POINT('Ctrl Pts',(-0.761915336443547,1.,-1.80351583877342));
#31488=CARTESIAN_POINT('Ctrl Pts',(-0.761229695230558,-1.,-1.79768986997783));
#31489=CARTESIAN_POINT('Ctrl Pts',(-0.761229695230558,1.,-1.79768986997783));
#31490=CARTESIAN_POINT('Ctrl Pts',(-0.760469555880749,-1.,-1.7918581561088));
#31491=CARTESIAN_POINT('Ctrl Pts',(-0.760469555880749,1.,-1.7918581561088));
#31492=CARTESIAN_POINT('Ctrl Pts',(-0.759614401110189,-1.,-1.78596964884604));
#31493=CARTESIAN_POINT('Ctrl Pts',(-0.759614401110189,1.,-1.78596964884604));
#31494=CARTESIAN_POINT('Ctrl Pts',(-0.758650626677518,-1.,-1.77999411220945));
#31495=CARTESIAN_POINT('Ctrl Pts',(-0.758650626677518,1.,-1.77999411220945));
#31496=CARTESIAN_POINT('Ctrl Pts',(-0.757578264077029,-1.,-1.77394167108292));
#31497=CARTESIAN_POINT('Ctrl Pts',(-0.757578264077029,1.,-1.77394167108292));
#31498=CARTESIAN_POINT('Ctrl Pts',(-0.75642189602781,-1.,-1.76789396002998));
#31499=CARTESIAN_POINT('Ctrl Pts',(-0.75642189602781,1.,-1.76789396002998));
#31500=CARTESIAN_POINT('Ctrl Pts',(-0.755220979974461,-1.,-1.76197817240128));
#31501=CARTESIAN_POINT('Ctrl Pts',(-0.755220979974461,1.,-1.76197817240128));
#31502=CARTESIAN_POINT('Ctrl Pts',(-0.754009254027829,-1.,-1.75631083600019));
#31503=CARTESIAN_POINT('Ctrl Pts',(-0.754009254027829,1.,-1.75631083600019));
#31504=CARTESIAN_POINT('Ctrl Pts',(-0.752797683531314,-1.,-1.75095139468794));
#31505=CARTESIAN_POINT('Ctrl Pts',(-0.752797683531314,1.,-1.75095139468794));
#31506=CARTESIAN_POINT('Ctrl Pts',(-0.751555614164482,-1.,-1.74585086852502));
#31507=CARTESIAN_POINT('Ctrl Pts',(-0.751555614164482,1.,-1.74585086852502));
#31508=CARTESIAN_POINT('Ctrl Pts',(-0.750193435981249,-1.,-1.74080458267114));
#31509=CARTESIAN_POINT('Ctrl Pts',(-0.750193435981249,1.,-1.74080458267114));
#31510=CARTESIAN_POINT('Ctrl Pts',(-0.74858246295687,-1.,-1.7355035168033));
#31511=CARTESIAN_POINT('Ctrl Pts',(-0.74858246295687,1.,-1.7355035168033));
#31512=CARTESIAN_POINT('Ctrl Pts',(-0.746574710097752,-1.,-1.72958533647714));
#31513=CARTESIAN_POINT('Ctrl Pts',(-0.746574710097752,1.,-1.72958533647714));
#31514=CARTESIAN_POINT('Ctrl Pts',(-0.744021445433093,-1.,-1.72268229916769));
#31515=CARTESIAN_POINT('Ctrl Pts',(-0.744021445433093,1.,-1.72268229916769));
#31516=CARTESIAN_POINT('Ctrl Pts',(-0.74079516202821,-1.,-1.71447789751001));
#31517=CARTESIAN_POINT('Ctrl Pts',(-0.74079516202821,1.,-1.71447789751001));
#31518=CARTESIAN_POINT('Ctrl Pts',(-0.736799665716932,-1.,-1.70473309004249));
#31519=CARTESIAN_POINT('Ctrl Pts',(-0.736799665716932,1.,-1.70473309004249));
#31520=CARTESIAN_POINT('Ctrl Pts',(-0.731963238685357,-1.,-1.69326921972915));
#31521=CARTESIAN_POINT('Ctrl Pts',(-0.731963238685357,1.,-1.69326921972915));
#31522=CARTESIAN_POINT('Ctrl Pts',(-0.726235967982445,-1.,-1.67996158451922));
#31523=CARTESIAN_POINT('Ctrl Pts',(-0.726235967982445,1.,-1.67996158451922));
#31524=CARTESIAN_POINT('Ctrl Pts',(-0.71958543378795,-1.,-1.66472880551777));
#31525=CARTESIAN_POINT('Ctrl Pts',(-0.71958543378795,1.,-1.66472880551777));
#31526=CARTESIAN_POINT('Ctrl Pts',(-0.711993139340447,-1.,-1.64752408828442));
#31527=CARTESIAN_POINT('Ctrl Pts',(-0.711993139340447,1.,-1.64752408828442));
#31528=CARTESIAN_POINT('Ctrl Pts',(-0.705159151977294,-1.,-1.6321654166204));
#31529=CARTESIAN_POINT('Ctrl Pts',(-0.705159151977294,1.,-1.6321654166204));
#31530=CARTESIAN_POINT('Ctrl Pts',(-0.699605146398837,-1.,-1.61974673471117));
#31531=CARTESIAN_POINT('Ctrl Pts',(-0.699605146398837,1.,-1.61974673471117));
#31532=CARTESIAN_POINT('Ctrl Pts',(-0.69571209787897,-1.,-1.61106790957619));
#31533=CARTESIAN_POINT('Ctrl Pts',(-0.69571209787897,1.,-1.61106790957619));
#31534=CARTESIAN_POINT('Ctrl Pts',(-0.693717979106305,-1.,-1.60662857109684));
#31535=CARTESIAN_POINT('Ctrl Pts',(-0.693717979106305,1.,-1.60662857109684));
#31536=CARTESIAN_POINT('',(-0.745574324794401,1.,-2.0698113262342));
#31537=CARTESIAN_POINT('Ctrl Pts',(-0.745574324794401,1.,-2.0698113262342));
#31538=CARTESIAN_POINT('Ctrl Pts',(-0.745832791378367,1.,-2.06854248895728));
#31539=CARTESIAN_POINT('Ctrl Pts',(-0.7463458715442,1.,-2.06600523016815));
#31540=CARTESIAN_POINT('Ctrl Pts',(-0.747103932787919,1.,-2.06220058927826));
#31541=CARTESIAN_POINT('Ctrl Pts',(-0.748091554183802,1.,-2.05713023031006));
#31542=CARTESIAN_POINT('Ctrl Pts',(-0.749287468665046,1.,-2.05079645592154));
#31543=CARTESIAN_POINT('Ctrl Pts',(-0.750444657875576,1.,-2.04446689147979));
#31544=CARTESIAN_POINT('Ctrl Pts',(-0.751562963361115,1.,-2.03814160092099));
#31545=CARTESIAN_POINT('Ctrl Pts',(-0.752642180487211,1.,-2.03182068456221));
#31546=CARTESIAN_POINT('Ctrl Pts',(-0.753682061112768,1.,-2.02550428623313));
#31547=CARTESIAN_POINT('Ctrl Pts',(-0.754682330722816,1.,-2.01919259405809));
#31548=CARTESIAN_POINT('Ctrl Pts',(-0.755642704957865,1.,-2.01288584328084));
#31549=CARTESIAN_POINT('Ctrl Pts',(-0.75656290464667,1.,-2.0065843158773));
#31550=CARTESIAN_POINT('Ctrl Pts',(-0.757442676862724,1.,-2.00028834739178));
#31551=CARTESIAN_POINT('Ctrl Pts',(-0.758281796766761,1.,-1.99399831098817));
#31552=CARTESIAN_POINT('Ctrl Pts',(-0.759080037802488,1.,-1.98771456680874));
#31553=CARTESIAN_POINT('Ctrl Pts',(-0.75983714745219,1.,-1.98143741418172));
#31554=CARTESIAN_POINT('Ctrl Pts',(-0.760552825409757,1.,-1.97516705321494));
#31555=CARTESIAN_POINT('Ctrl Pts',(-0.76122669048382,1.,-1.96890351582499));
#31556=CARTESIAN_POINT('Ctrl Pts',(-0.761858300014423,1.,-1.96264672744186));
#31557=CARTESIAN_POINT('Ctrl Pts',(-0.762447203806179,1.,-1.95639665309869));
#31558=CARTESIAN_POINT('Ctrl Pts',(-0.762992990878769,1.,-1.95015342590024));
#31559=CARTESIAN_POINT('Ctrl Pts',(-0.763495333538629,1.,-1.9439174661764));
#31560=CARTESIAN_POINT('Ctrl Pts',(-0.763954049121458,1.,-1.93768964875886));
#31561=CARTESIAN_POINT('Ctrl Pts',(-0.764369010673941,1.,-1.93147105496382));
#31562=CARTESIAN_POINT('Ctrl Pts',(-0.764740025488211,1.,-1.92526263537048));
#31563=CARTESIAN_POINT('Ctrl Pts',(-0.765066729667088,1.,-1.91906491634196));
#31564=CARTESIAN_POINT('Ctrl Pts',(-0.765348465884722,1.,-1.91287765805169));
#31565=CARTESIAN_POINT('Ctrl Pts',(-0.765584196937919,1.,-1.90669961402356));
#31566=CARTESIAN_POINT('Ctrl Pts',(-0.765772772593386,1.,-1.90052930393596));
#31567=CARTESIAN_POINT('Ctrl Pts',(-0.765913193856978,1.,-1.89436577771388));
#31568=CARTESIAN_POINT('Ctrl Pts',(-0.766004837062091,1.,-1.88820926433409));
#31569=CARTESIAN_POINT('Ctrl Pts',(-0.766047794851865,1.,-1.88206215302561));
#31570=CARTESIAN_POINT('Ctrl Pts',(-0.766042837036744,1.,-1.87592888967883));
#31571=CARTESIAN_POINT('Ctrl Pts',(-0.765990708546091,1.,-1.86981398314341));
#31572=CARTESIAN_POINT('Ctrl Pts',(-0.765891519092547,1.,-1.86372027063312));
#31573=CARTESIAN_POINT('Ctrl Pts',(-0.765744212909318,1.,-1.85764741390394));
#31574=CARTESIAN_POINT('Ctrl Pts',(-0.765545710619062,1.,-1.85158945130063));
#31575=CARTESIAN_POINT('Ctrl Pts',(-0.765291664862029,1.,-1.84553698875924));
#31576=CARTESIAN_POINT('Ctrl Pts',(-0.764978057881737,1.,-1.83948181064835));
#31577=CARTESIAN_POINT('Ctrl Pts',(-0.764602549687853,1.,-1.83342077227142));
#31578=CARTESIAN_POINT('Ctrl Pts',(-0.764165902605995,1.,-1.82735991200065));
#31579=CARTESIAN_POINT('Ctrl Pts',(-0.763673465462726,1.,-1.82131873145266));
#31580=CARTESIAN_POINT('Ctrl Pts',(-0.763132003836634,1.,-1.8153211840553));
#31581=CARTESIAN_POINT('Ctrl Pts',(-0.762546129463938,1.,-1.80938551463965));
#31582=CARTESIAN_POINT('Ctrl Pts',(-0.761915336443547,1.,-1.80351583877342));
#31583=CARTESIAN_POINT('Ctrl Pts',(-0.761229695230558,1.,-1.79768986997783));
#31584=CARTESIAN_POINT('Ctrl Pts',(-0.760469555880749,1.,-1.7918581561088));
#31585=CARTESIAN_POINT('Ctrl Pts',(-0.759614401110189,1.,-1.78596964884604));
#31586=CARTESIAN_POINT('Ctrl Pts',(-0.758650626677518,1.,-1.77999411220945));
#31587=CARTESIAN_POINT('Ctrl Pts',(-0.757578264077029,1.,-1.77394167108292));
#31588=CARTESIAN_POINT('Ctrl Pts',(-0.75642189602781,1.,-1.76789396002998));
#31589=CARTESIAN_POINT('Ctrl Pts',(-0.755220979974461,1.,-1.76197817240128));
#31590=CARTESIAN_POINT('Ctrl Pts',(-0.754009254027829,1.,-1.75631083600019));
#31591=CARTESIAN_POINT('Ctrl Pts',(-0.752797683531314,1.,-1.75095139468794));
#31592=CARTESIAN_POINT('Ctrl Pts',(-0.751555614164482,1.,-1.74585086852502));
#31593=CARTESIAN_POINT('Ctrl Pts',(-0.750193435981249,1.,-1.74080458267114));
#31594=CARTESIAN_POINT('Ctrl Pts',(-0.74858246295687,1.,-1.7355035168033));
#31595=CARTESIAN_POINT('Ctrl Pts',(-0.746574710097752,1.,-1.72958533647714));
#31596=CARTESIAN_POINT('Ctrl Pts',(-0.744021445433093,1.,-1.72268229916769));
#31597=CARTESIAN_POINT('Ctrl Pts',(-0.74079516202821,1.,-1.71447789751001));
#31598=CARTESIAN_POINT('Ctrl Pts',(-0.736799665716932,1.,-1.70473309004249));
#31599=CARTESIAN_POINT('Ctrl Pts',(-0.731963238685357,1.,-1.69326921972915));
#31600=CARTESIAN_POINT('Ctrl Pts',(-0.726235967982445,1.,-1.67996158451922));
#31601=CARTESIAN_POINT('Ctrl Pts',(-0.71958543378795,1.,-1.66472880551777));
#31602=CARTESIAN_POINT('Ctrl Pts',(-0.711993139340447,1.,-1.64752408828442));
#31603=CARTESIAN_POINT('Ctrl Pts',(-0.705159151977294,1.,-1.6321654166204));
#31604=CARTESIAN_POINT('Ctrl Pts',(-0.699605146398837,1.,-1.61974673471117));
#31605=CARTESIAN_POINT('Ctrl Pts',(-0.69571209787897,1.,-1.61106790957619));
#31606=CARTESIAN_POINT('Ctrl Pts',(-0.693717979106305,1.,-1.60662857109684));
#31607=CARTESIAN_POINT('',(-0.745574324794401,0.,-2.0698113262342));
#31608=CARTESIAN_POINT('Origin',(-0.61342227326009,0.,-2.11275013067528));
#31609=CARTESIAN_POINT('',(-0.61342227326009,1.,-2.11275013067528));
#31610=CARTESIAN_POINT('',(-0.745574324794401,1.,-2.0698113262342));
#31611=CARTESIAN_POINT('',(-0.61342227326009,0.,-2.11275013067528));
#31612=CARTESIAN_POINT('Ctrl Pts',(-0.383122945602004,-1.,-1.7075470150345));
#31613=CARTESIAN_POINT('Ctrl Pts',(-0.383122945602004,1.,-1.7075470150345));
#31614=CARTESIAN_POINT('Ctrl Pts',(-0.384119047315542,-1.,-1.71231062891958));
#31615=CARTESIAN_POINT('Ctrl Pts',(-0.384119047315542,1.,-1.71231062891958));
#31616=CARTESIAN_POINT('Ctrl Pts',(-0.38607079032701,-1.,-1.72162022246158));
#31617=CARTESIAN_POINT('Ctrl Pts',(-0.38607079032701,1.,-1.72162022246158));
#31618=CARTESIAN_POINT('Ctrl Pts',(-0.388877023509191,-1.,-1.7349317097561));
#31619=CARTESIAN_POINT('Ctrl Pts',(-0.388877023509191,1.,-1.7349317097561));
#31620=CARTESIAN_POINT('Ctrl Pts',(-0.392375812294307,-1.,-1.75137405313962));
#31621=CARTESIAN_POINT('Ctrl Pts',(-0.392375812294307,1.,-1.75137405313962));
#31622=CARTESIAN_POINT('Ctrl Pts',(-0.39634619612042,-1.,-1.7697556004756));
#31623=CARTESIAN_POINT('Ctrl Pts',(-0.39634619612042,1.,-1.7697556004756));
#31624=CARTESIAN_POINT('Ctrl Pts',(-0.39991940378308,-1.,-1.78598826347533));
#31625=CARTESIAN_POINT('Ctrl Pts',(-0.39991940378308,1.,-1.78598826347533));
#31626=CARTESIAN_POINT('Ctrl Pts',(-0.403107976170441,-1.,-1.80012077176221));
#31627=CARTESIAN_POINT('Ctrl Pts',(-0.403107976170441,1.,-1.80012077176221));
#31628=CARTESIAN_POINT('Ctrl Pts',(-0.405933518411838,-1.,-1.81223801813988));
#31629=CARTESIAN_POINT('Ctrl Pts',(-0.405933518411838,1.,-1.81223801813988));
#31630=CARTESIAN_POINT('Ctrl Pts',(-0.408428948108533,-1.,-1.8224702267854));
#31631=CARTESIAN_POINT('Ctrl Pts',(-0.408428948108533,1.,-1.8224702267854));
#31632=CARTESIAN_POINT('Ctrl Pts',(-0.410641256301675,-1.,-1.83100408895216));
#31633=CARTESIAN_POINT('Ctrl Pts',(-0.410641256301675,1.,-1.83100408895216));
#31634=CARTESIAN_POINT('Ctrl Pts',(-0.412633125322162,-1.,-1.83808953475839));
#31635=CARTESIAN_POINT('Ctrl Pts',(-0.412633125322162,1.,-1.83808953475839));
#31636=CARTESIAN_POINT('Ctrl Pts',(-0.41448743825434,-1.,-1.8440575707371));
#31637=CARTESIAN_POINT('Ctrl Pts',(-0.41448743825434,1.,-1.8440575707371));
#31638=CARTESIAN_POINT('Ctrl Pts',(-0.416300022038864,-1.,-1.84929312929882));
#31639=CARTESIAN_POINT('Ctrl Pts',(-0.416300022038864,1.,-1.84929312929882));
#31640=CARTESIAN_POINT('Ctrl Pts',(-0.418164129143534,-1.,-1.85417632856234));
#31641=CARTESIAN_POINT('Ctrl Pts',(-0.418164129143534,1.,-1.85417632856234));
#31642=CARTESIAN_POINT('Ctrl Pts',(-0.420157287975619,-1.,-1.85903281096686));
#31643=CARTESIAN_POINT('Ctrl Pts',(-0.420157287975619,1.,-1.85903281096686));
#31644=CARTESIAN_POINT('Ctrl Pts',(-0.422327307418275,-1.,-1.86408083334028));
#31645=CARTESIAN_POINT('Ctrl Pts',(-0.422327307418275,1.,-1.86408083334028));
#31646=CARTESIAN_POINT('Ctrl Pts',(-0.424678177291359,-1.,-1.86937803944323));
#31647=CARTESIAN_POINT('Ctrl Pts',(-0.424678177291359,1.,-1.86937803944323));
#31648=CARTESIAN_POINT('Ctrl Pts',(-0.427183828519102,-1.,-1.87486989291484));
#31649=CARTESIAN_POINT('Ctrl Pts',(-0.427183828519102,1.,-1.87486989291484));
#31650=CARTESIAN_POINT('Ctrl Pts',(-0.429803062482344,-1.,-1.88044229001832));
#31651=CARTESIAN_POINT('Ctrl Pts',(-0.429803062482344,1.,-1.88044229001832));
#31652=CARTESIAN_POINT('Ctrl Pts',(-0.432493038548748,-1.,-1.88596913666793));
#31653=CARTESIAN_POINT('Ctrl Pts',(-0.432493038548748,1.,-1.88596913666793));
#31654=CARTESIAN_POINT('Ctrl Pts',(-0.435225660963383,-1.,-1.89136993975504));
#31655=CARTESIAN_POINT('Ctrl Pts',(-0.435225660963383,1.,-1.89136993975504));
#31656=CARTESIAN_POINT('Ctrl Pts',(-0.437995003948244,-1.,-1.89663648956466));
#31657=CARTESIAN_POINT('Ctrl Pts',(-0.437995003948244,1.,-1.89663648956466));
#31658=CARTESIAN_POINT('Ctrl Pts',(-0.440807833704038,-1.,-1.90180124389086));
#31659=CARTESIAN_POINT('Ctrl Pts',(-0.440807833704038,1.,-1.90180124389086));
#31660=CARTESIAN_POINT('Ctrl Pts',(-0.443677556849151,-1.,-1.90691756144898));
#31661=CARTESIAN_POINT('Ctrl Pts',(-0.443677556849151,1.,-1.90691756144898));
#31662=CARTESIAN_POINT('Ctrl Pts',(-0.446617343485711,-1.,-1.9120369998112));
#31663=CARTESIAN_POINT('Ctrl Pts',(-0.446617343485711,1.,-1.9120369998112));
#31664=CARTESIAN_POINT('Ctrl Pts',(-0.449632260106662,-1.,-1.91718342555755));
#31665=CARTESIAN_POINT('Ctrl Pts',(-0.449632260106662,1.,-1.91718342555755));
#31666=CARTESIAN_POINT('Ctrl Pts',(-0.452719478359432,-1.,-1.92235380648502));
#31667=CARTESIAN_POINT('Ctrl Pts',(-0.452719478359432,1.,-1.92235380648502));
#31668=CARTESIAN_POINT('Ctrl Pts',(-0.455872005174371,-1.,-1.92753067150476));
#31669=CARTESIAN_POINT('Ctrl Pts',(-0.455872005174371,1.,-1.92753067150476));
#31670=CARTESIAN_POINT('Ctrl Pts',(-0.459081234547926,-1.,-1.93269066517934));
#31671=CARTESIAN_POINT('Ctrl Pts',(-0.459081234547926,1.,-1.93269066517934));
#31672=CARTESIAN_POINT('Ctrl Pts',(-0.462340031009056,-1.,-1.93781486640821));
#31673=CARTESIAN_POINT('Ctrl Pts',(-0.462340031009056,1.,-1.93781486640821));
#31674=CARTESIAN_POINT('Ctrl Pts',(-0.46564546202603,-1.,-1.9428979419619));
#31675=CARTESIAN_POINT('Ctrl Pts',(-0.46564546202603,1.,-1.9428979419619));
#31676=CARTESIAN_POINT('Ctrl Pts',(-0.468997482913135,-1.,-1.94794381136514));
#31677=CARTESIAN_POINT('Ctrl Pts',(-0.468997482913135,1.,-1.94794381136514));
#31678=CARTESIAN_POINT('Ctrl Pts',(-0.472397672264072,-1.,-1.95296148278133));
#31679=CARTESIAN_POINT('Ctrl Pts',(-0.472397672264072,1.,-1.95296148278133));
#31680=CARTESIAN_POINT('Ctrl Pts',(-0.475848034683176,-1.,-1.95796111148177));
#31681=CARTESIAN_POINT('Ctrl Pts',(-0.475848034683176,1.,-1.95796111148177));
#31682=CARTESIAN_POINT('Ctrl Pts',(-0.479349583074855,-1.,-1.96294933055943));
#31683=CARTESIAN_POINT('Ctrl Pts',(-0.479349583074855,1.,-1.96294933055943));
#31684=CARTESIAN_POINT('Ctrl Pts',(-0.482901662120691,-1.,-1.96792703422362));
#31685=CARTESIAN_POINT('Ctrl Pts',(-0.482901662120691,1.,-1.96792703422362));
#31686=CARTESIAN_POINT('Ctrl Pts',(-0.486502692907659,-1.,-1.97289186263272));
#31687=CARTESIAN_POINT('Ctrl Pts',(-0.486502692907659,1.,-1.97289186263272));
#31688=CARTESIAN_POINT('Ctrl Pts',(-0.490150627860952,-1.,-1.97783973019229));
#31689=CARTESIAN_POINT('Ctrl Pts',(-0.490150627860952,1.,-1.97783973019229));
#31690=CARTESIAN_POINT('Ctrl Pts',(-0.493843476541495,-1.,-1.98276658761821));
#31691=CARTESIAN_POINT('Ctrl Pts',(-0.493843476541495,1.,-1.98276658761821));
#31692=CARTESIAN_POINT('Ctrl Pts',(-0.497579909545574,-1.,-1.98767044752932));
#31693=CARTESIAN_POINT('Ctrl Pts',(-0.497579909545574,1.,-1.98767044752932));
#31694=CARTESIAN_POINT('Ctrl Pts',(-0.501359287727146,-1.,-1.99255149126155));
#31695=CARTESIAN_POINT('Ctrl Pts',(-0.501359287727146,1.,-1.99255149126155));
#31696=CARTESIAN_POINT('Ctrl Pts',(-0.505181361323026,-1.,-1.99741107463572));
#31697=CARTESIAN_POINT('Ctrl Pts',(-0.505181361323026,1.,-1.99741107463572));
#31698=CARTESIAN_POINT('Ctrl Pts',(-0.509046069886157,-1.,-2.00225107134734));
#31699=CARTESIAN_POINT('Ctrl Pts',(-0.509046069886157,1.,-2.00225107134734));
#31700=CARTESIAN_POINT('Ctrl Pts',(-0.512953306961792,-1.,-2.00707309946949));
#31701=CARTESIAN_POINT('Ctrl Pts',(-0.512953306961792,1.,-2.00707309946949));
#31702=CARTESIAN_POINT('Ctrl Pts',(-0.516902681728687,-1.,-2.01187773939242));
#31703=CARTESIAN_POINT('Ctrl Pts',(-0.516902681728687,1.,-2.01187773939242));
#31704=CARTESIAN_POINT('Ctrl Pts',(-0.52089359039937,-1.,-2.01666477917286));
#31705=CARTESIAN_POINT('Ctrl Pts',(-0.52089359039937,1.,-2.01666477917286));
#31706=CARTESIAN_POINT('Ctrl Pts',(-0.524925318333476,-1.,-2.02143356304698));
#31707=CARTESIAN_POINT('Ctrl Pts',(-0.524925318333476,1.,-2.02143356304698));
#31708=CARTESIAN_POINT('Ctrl Pts',(-0.528997127241914,-1.,-2.0261832908329));
#31709=CARTESIAN_POINT('Ctrl Pts',(-0.528997127241914,1.,-2.0261832908329));
#31710=CARTESIAN_POINT('Ctrl Pts',(-0.533108355132977,-1.,-2.03091336214426));
#31711=CARTESIAN_POINT('Ctrl Pts',(-0.533108355132977,1.,-2.03091336214426));
#31712=CARTESIAN_POINT('Ctrl Pts',(-0.537258489833262,-1.,-2.03562362954037));
#31713=CARTESIAN_POINT('Ctrl Pts',(-0.537258489833262,1.,-2.03562362954037));
#31714=CARTESIAN_POINT('Ctrl Pts',(-0.541447120615659,-1.,-2.04031422690527));
#31715=CARTESIAN_POINT('Ctrl Pts',(-0.541447120615659,1.,-2.04031422690527));
#31716=CARTESIAN_POINT('Ctrl Pts',(-0.54567390381743,-1.,-2.04498544714588));
#31717=CARTESIAN_POINT('Ctrl Pts',(-0.54567390381743,1.,-2.04498544714588));
#31718=CARTESIAN_POINT('Ctrl Pts',(-0.549938525150295,-1.,-2.04963761077958));
#31719=CARTESIAN_POINT('Ctrl Pts',(-0.549938525150295,1.,-2.04963761077958));
#31720=CARTESIAN_POINT('Ctrl Pts',(-0.554240657463906,-1.,-2.05427091604413));
#31721=CARTESIAN_POINT('Ctrl Pts',(-0.554240657463906,1.,-2.05427091604413));
#31722=CARTESIAN_POINT('Ctrl Pts',(-0.558579940185151,-1.,-2.05888537756462));
#31723=CARTESIAN_POINT('Ctrl Pts',(-0.558579940185151,1.,-2.05888537756462));
#31724=CARTESIAN_POINT('Ctrl Pts',(-0.562955993082261,-1.,-2.06348090160589));
#31725=CARTESIAN_POINT('Ctrl Pts',(-0.562955993082261,1.,-2.06348090160589));
#31726=CARTESIAN_POINT('Ctrl Pts',(-0.567368421181087,-1.,-2.06805732997334));
#31727=CARTESIAN_POINT('Ctrl Pts',(-0.567368421181087,1.,-2.06805732997334));
#31728=CARTESIAN_POINT('Ctrl Pts',(-0.571816823242603,-1.,-2.07261449292824));
#31729=CARTESIAN_POINT('Ctrl Pts',(-0.571816823242603,1.,-2.07261449292824));
#31730=CARTESIAN_POINT('Ctrl Pts',(-0.576300797416844,-1.,-2.07715226767559));
#31731=CARTESIAN_POINT('Ctrl Pts',(-0.576300797416844,1.,-2.07715226767559));
#31732=CARTESIAN_POINT('Ctrl Pts',(-0.580819952108063,-1.,-2.08167059018418));
#31733=CARTESIAN_POINT('Ctrl Pts',(-0.580819952108063,1.,-2.08167059018418));
#31734=CARTESIAN_POINT('Ctrl Pts',(-0.585373918991617,-1.,-2.08616943727951));
#31735=CARTESIAN_POINT('Ctrl Pts',(-0.585373918991617,1.,-2.08616943727951));
#31736=CARTESIAN_POINT('Ctrl Pts',(-0.589962365403406,-1.,-2.09064881812129));
#31737=CARTESIAN_POINT('Ctrl Pts',(-0.589962365403406,1.,-2.09064881812129));
#31738=CARTESIAN_POINT('Ctrl Pts',(-0.594585006052162,-1.,-2.0951087622027));
#31739=CARTESIAN_POINT('Ctrl Pts',(-0.594585006052162,1.,-2.0951087622027));
#31740=CARTESIAN_POINT('Ctrl Pts',(-0.599241616420533,-1.,-2.0995493086477));
#31741=CARTESIAN_POINT('Ctrl Pts',(-0.599241616420533,1.,-2.0995493086477));
#31742=CARTESIAN_POINT('Ctrl Pts',(-0.60393203073603,-1.,-2.10397049886949));
#31743=CARTESIAN_POINT('Ctrl Pts',(-0.60393203073603,1.,-2.10397049886949));
#31744=CARTESIAN_POINT('Ctrl Pts',(-0.607711315454876,-1.,-2.1074919961518));
#31745=CARTESIAN_POINT('Ctrl Pts',(-0.607711315454876,1.,-2.1074919961518));
#31746=CARTESIAN_POINT('Ctrl Pts',(-0.610560911689899,-1.,-2.11012443807238));
#31747=CARTESIAN_POINT('Ctrl Pts',(-0.610560911689899,1.,-2.11012443807238));
#31748=CARTESIAN_POINT('Ctrl Pts',(-0.6124673655618,-1.,-2.11187554259986));
#31749=CARTESIAN_POINT('Ctrl Pts',(-0.6124673655618,1.,-2.11187554259986));
#31750=CARTESIAN_POINT('Ctrl Pts',(-0.61342227326009,-1.,-2.11275013067528));
#31751=CARTESIAN_POINT('Ctrl Pts',(-0.61342227326009,1.,-2.11275013067528));
#31752=CARTESIAN_POINT('',(-0.383122945602004,1.,-1.7075470150345));
#31753=CARTESIAN_POINT('Ctrl Pts',(-0.383122945602004,1.,-1.7075470150345));
#31754=CARTESIAN_POINT('Ctrl Pts',(-0.384119047315542,1.,-1.71231062891958));
#31755=CARTESIAN_POINT('Ctrl Pts',(-0.38607079032701,1.,-1.72162022246158));
#31756=CARTESIAN_POINT('Ctrl Pts',(-0.388877023509191,1.,-1.7349317097561));
#31757=CARTESIAN_POINT('Ctrl Pts',(-0.392375812294307,1.,-1.75137405313962));
#31758=CARTESIAN_POINT('Ctrl Pts',(-0.39634619612042,1.,-1.7697556004756));
#31759=CARTESIAN_POINT('Ctrl Pts',(-0.39991940378308,1.,-1.78598826347533));
#31760=CARTESIAN_POINT('Ctrl Pts',(-0.403107976170441,1.,-1.80012077176221));
#31761=CARTESIAN_POINT('Ctrl Pts',(-0.405933518411838,1.,-1.81223801813988));
#31762=CARTESIAN_POINT('Ctrl Pts',(-0.408428948108533,1.,-1.8224702267854));
#31763=CARTESIAN_POINT('Ctrl Pts',(-0.410641256301675,1.,-1.83100408895216));
#31764=CARTESIAN_POINT('Ctrl Pts',(-0.412633125322162,1.,-1.83808953475839));
#31765=CARTESIAN_POINT('Ctrl Pts',(-0.41448743825434,1.,-1.8440575707371));
#31766=CARTESIAN_POINT('Ctrl Pts',(-0.416300022038864,1.,-1.84929312929882));
#31767=CARTESIAN_POINT('Ctrl Pts',(-0.418164129143534,1.,-1.85417632856234));
#31768=CARTESIAN_POINT('Ctrl Pts',(-0.420157287975619,1.,-1.85903281096686));
#31769=CARTESIAN_POINT('Ctrl Pts',(-0.422327307418275,1.,-1.86408083334028));
#31770=CARTESIAN_POINT('Ctrl Pts',(-0.424678177291359,1.,-1.86937803944323));
#31771=CARTESIAN_POINT('Ctrl Pts',(-0.427183828519102,1.,-1.87486989291484));
#31772=CARTESIAN_POINT('Ctrl Pts',(-0.429803062482344,1.,-1.88044229001832));
#31773=CARTESIAN_POINT('Ctrl Pts',(-0.432493038548748,1.,-1.88596913666793));
#31774=CARTESIAN_POINT('Ctrl Pts',(-0.435225660963383,1.,-1.89136993975504));
#31775=CARTESIAN_POINT('Ctrl Pts',(-0.437995003948244,1.,-1.89663648956466));
#31776=CARTESIAN_POINT('Ctrl Pts',(-0.440807833704038,1.,-1.90180124389086));
#31777=CARTESIAN_POINT('Ctrl Pts',(-0.443677556849151,1.,-1.90691756144898));
#31778=CARTESIAN_POINT('Ctrl Pts',(-0.446617343485711,1.,-1.9120369998112));
#31779=CARTESIAN_POINT('Ctrl Pts',(-0.449632260106662,1.,-1.91718342555755));
#31780=CARTESIAN_POINT('Ctrl Pts',(-0.452719478359432,1.,-1.92235380648502));
#31781=CARTESIAN_POINT('Ctrl Pts',(-0.455872005174371,1.,-1.92753067150476));
#31782=CARTESIAN_POINT('Ctrl Pts',(-0.459081234547926,1.,-1.93269066517934));
#31783=CARTESIAN_POINT('Ctrl Pts',(-0.462340031009056,1.,-1.93781486640821));
#31784=CARTESIAN_POINT('Ctrl Pts',(-0.46564546202603,1.,-1.9428979419619));
#31785=CARTESIAN_POINT('Ctrl Pts',(-0.468997482913135,1.,-1.94794381136514));
#31786=CARTESIAN_POINT('Ctrl Pts',(-0.472397672264072,1.,-1.95296148278133));
#31787=CARTESIAN_POINT('Ctrl Pts',(-0.475848034683176,1.,-1.95796111148177));
#31788=CARTESIAN_POINT('Ctrl Pts',(-0.479349583074855,1.,-1.96294933055943));
#31789=CARTESIAN_POINT('Ctrl Pts',(-0.482901662120691,1.,-1.96792703422362));
#31790=CARTESIAN_POINT('Ctrl Pts',(-0.486502692907659,1.,-1.97289186263272));
#31791=CARTESIAN_POINT('Ctrl Pts',(-0.490150627860952,1.,-1.97783973019229));
#31792=CARTESIAN_POINT('Ctrl Pts',(-0.493843476541495,1.,-1.98276658761821));
#31793=CARTESIAN_POINT('Ctrl Pts',(-0.497579909545574,1.,-1.98767044752932));
#31794=CARTESIAN_POINT('Ctrl Pts',(-0.501359287727146,1.,-1.99255149126155));
#31795=CARTESIAN_POINT('Ctrl Pts',(-0.505181361323026,1.,-1.99741107463572));
#31796=CARTESIAN_POINT('Ctrl Pts',(-0.509046069886157,1.,-2.00225107134734));
#31797=CARTESIAN_POINT('Ctrl Pts',(-0.512953306961792,1.,-2.00707309946949));
#31798=CARTESIAN_POINT('Ctrl Pts',(-0.516902681728687,1.,-2.01187773939242));
#31799=CARTESIAN_POINT('Ctrl Pts',(-0.52089359039937,1.,-2.01666477917286));
#31800=CARTESIAN_POINT('Ctrl Pts',(-0.524925318333476,1.,-2.02143356304698));
#31801=CARTESIAN_POINT('Ctrl Pts',(-0.528997127241914,1.,-2.0261832908329));
#31802=CARTESIAN_POINT('Ctrl Pts',(-0.533108355132977,1.,-2.03091336214426));
#31803=CARTESIAN_POINT('Ctrl Pts',(-0.537258489833262,1.,-2.03562362954037));
#31804=CARTESIAN_POINT('Ctrl Pts',(-0.541447120615659,1.,-2.04031422690527));
#31805=CARTESIAN_POINT('Ctrl Pts',(-0.54567390381743,1.,-2.04498544714588));
#31806=CARTESIAN_POINT('Ctrl Pts',(-0.549938525150295,1.,-2.04963761077958));
#31807=CARTESIAN_POINT('Ctrl Pts',(-0.554240657463906,1.,-2.05427091604413));
#31808=CARTESIAN_POINT('Ctrl Pts',(-0.558579940185151,1.,-2.05888537756462));
#31809=CARTESIAN_POINT('Ctrl Pts',(-0.562955993082261,1.,-2.06348090160589));
#31810=CARTESIAN_POINT('Ctrl Pts',(-0.567368421181087,1.,-2.06805732997334));
#31811=CARTESIAN_POINT('Ctrl Pts',(-0.571816823242603,1.,-2.07261449292824));
#31812=CARTESIAN_POINT('Ctrl Pts',(-0.576300797416844,1.,-2.07715226767559));
#31813=CARTESIAN_POINT('Ctrl Pts',(-0.580819952108063,1.,-2.08167059018418));
#31814=CARTESIAN_POINT('Ctrl Pts',(-0.585373918991617,1.,-2.08616943727951));
#31815=CARTESIAN_POINT('Ctrl Pts',(-0.589962365403406,1.,-2.09064881812129));
#31816=CARTESIAN_POINT('Ctrl Pts',(-0.594585006052162,1.,-2.0951087622027));
#31817=CARTESIAN_POINT('Ctrl Pts',(-0.599241616420533,1.,-2.0995493086477));
#31818=CARTESIAN_POINT('Ctrl Pts',(-0.60393203073603,1.,-2.10397049886949));
#31819=CARTESIAN_POINT('Ctrl Pts',(-0.607711315454876,1.,-2.1074919961518));
#31820=CARTESIAN_POINT('Ctrl Pts',(-0.610560911689899,1.,-2.11012443807238));
#31821=CARTESIAN_POINT('Ctrl Pts',(-0.6124673655618,1.,-2.11187554259986));
#31822=CARTESIAN_POINT('Ctrl Pts',(-0.61342227326009,1.,-2.11275013067528));
#31823=CARTESIAN_POINT('',(-0.383122945602003,0.,-1.7075470150345));
#31824=CARTESIAN_POINT('Origin',(0.,0.,0.));
#31825=CARTESIAN_POINT('',(-0.163289472382896,1.,-1.74236521665491));
#31826=CARTESIAN_POINT('Origin',(0.,1.,0.));
#31827=CARTESIAN_POINT('',(-0.163289472382896,0.,-1.74236521665491));
#31828=CARTESIAN_POINT('Ctrl Pts',(-0.0694764450219581,-1.,-2.19890268624765));
#31829=CARTESIAN_POINT('Ctrl Pts',(-0.0694764450219581,1.,-2.19890268624765));
#31830=CARTESIAN_POINT('Ctrl Pts',(-0.070114353632549,-1.,-2.19777582085423));
#31831=CARTESIAN_POINT('Ctrl Pts',(-0.070114353632549,1.,-2.19777582085423));
#31832=CARTESIAN_POINT('Ctrl Pts',(-0.0713863779526154,-1.,-2.19552129484002));
#31833=CARTESIAN_POINT('Ctrl Pts',(-0.0713863779526154,1.,-2.19552129484002));
#31834=CARTESIAN_POINT('Ctrl Pts',(-0.0732830357306725,-1.,-2.19213712013662));
#31835=CARTESIAN_POINT('Ctrl Pts',(-0.0732830357306725,1.,-2.19213712013662));
#31836=CARTESIAN_POINT('Ctrl Pts',(-0.0757891465836148,-1.,-2.1876201139953));
#31837=CARTESIAN_POINT('Ctrl Pts',(-0.0757891465836148,1.,-2.1876201139953));
#31838=CARTESIAN_POINT('Ctrl Pts',(-0.0788837727685243,-1.,-2.18196589448887));
#31839=CARTESIAN_POINT('Ctrl Pts',(-0.0788837727685243,1.,-2.18196589448887));
#31840=CARTESIAN_POINT('Ctrl Pts',(-0.0819402680872765,-1.,-2.176303712113));
#31841=CARTESIAN_POINT('Ctrl Pts',(-0.0819402680872765,1.,-2.176303712113));
#31842=CARTESIAN_POINT('Ctrl Pts',(-0.0849584620835372,-1.,-2.17063357870952));
#31843=CARTESIAN_POINT('Ctrl Pts',(-0.0849584620835372,1.,-2.17063357870952));
#31844=CARTESIAN_POINT('Ctrl Pts',(-0.0879381291386923,-1.,-2.16495552645014));
#31845=CARTESIAN_POINT('Ctrl Pts',(-0.0879381291386923,1.,-2.16495552645014));
#31846=CARTESIAN_POINT('Ctrl Pts',(-0.0908789888107265,-1.,-2.15926961544516));
#31847=CARTESIAN_POINT('Ctrl Pts',(-0.0908789888107265,1.,-2.15926961544516));
#31848=CARTESIAN_POINT('Ctrl Pts',(-0.0937807218867643,-1.,-2.1535759397817));
#31849=CARTESIAN_POINT('Ctrl Pts',(-0.0937807218867643,1.,-2.1535759397817));
#31850=CARTESIAN_POINT('Ctrl Pts',(-0.0966429852305459,-1.,-2.14787463531795));
#31851=CARTESIAN_POINT('Ctrl Pts',(-0.0966429852305459,1.,-2.14787463531795));
#31852=CARTESIAN_POINT('Ctrl Pts',(-0.0994654261990915,-1.,-2.14216588396025));
#31853=CARTESIAN_POINT('Ctrl Pts',(-0.0994654261990915,1.,-2.14216588396025));
#31854=CARTESIAN_POINT('Ctrl Pts',(-0.1022477005561,-1.,-2.13644992667165));
#31855=CARTESIAN_POINT('Ctrl Pts',(-0.1022477005561,1.,-2.13644992667165));
#31856=CARTESIAN_POINT('Ctrl Pts',(-0.104989479152739,-1.,-2.13072704887293));
#31857=CARTESIAN_POINT('Ctrl Pts',(-0.104989479152739,1.,-2.13072704887293));
#31858=CARTESIAN_POINT('Ctrl Pts',(-0.10769043523109,-1.,-2.12499752307));
#31859=CARTESIAN_POINT('Ctrl Pts',(-0.10769043523109,1.,-2.12499752307));
#31860=CARTESIAN_POINT('Ctrl Pts',(-0.110350236135025,-1.,-2.11926155590865));
#31861=CARTESIAN_POINT('Ctrl Pts',(-0.110350236135025,1.,-2.11926155590865));
#31862=CARTESIAN_POINT('Ctrl Pts',(-0.112968534419737,-1.,-2.11351924490306));
#31863=CARTESIAN_POINT('Ctrl Pts',(-0.112968534419737,1.,-2.11351924490306));
#31864=CARTESIAN_POINT('Ctrl Pts',(-0.115544957687926,-1.,-2.10777050261309));
#31865=CARTESIAN_POINT('Ctrl Pts',(-0.115544957687926,1.,-2.10777050261309));
#31866=CARTESIAN_POINT('Ctrl Pts',(-0.118079107988355,-1.,-2.102015121329));
#31867=CARTESIAN_POINT('Ctrl Pts',(-0.118079107988355,1.,-2.102015121329));
#31868=CARTESIAN_POINT('Ctrl Pts',(-0.120570567965122,-1.,-2.0962529286773));
#31869=CARTESIAN_POINT('Ctrl Pts',(-0.120570567965122,1.,-2.0962529286773));
#31870=CARTESIAN_POINT('Ctrl Pts',(-0.123018905621083,-1.,-2.09048392424825));
#31871=CARTESIAN_POINT('Ctrl Pts',(-0.123018905621083,1.,-2.09048392424825));
#31872=CARTESIAN_POINT('Ctrl Pts',(-0.125423679412061,-1.,-2.08470840653643));
#31873=CARTESIAN_POINT('Ctrl Pts',(-0.125423679412061,1.,-2.08470840653643));
#31874=CARTESIAN_POINT('Ctrl Pts',(-0.12778444527612,-1.,-2.07892715110987));
#31875=CARTESIAN_POINT('Ctrl Pts',(-0.12778444527612,1.,-2.07892715110987));
#31876=CARTESIAN_POINT('Ctrl Pts',(-0.130100748328403,-1.,-2.07314114713063));
#31877=CARTESIAN_POINT('Ctrl Pts',(-0.130100748328403,1.,-2.07314114713063));
#31878=CARTESIAN_POINT('Ctrl Pts',(-0.13237211154771,-1.,-2.06735123910326));
#31879=CARTESIAN_POINT('Ctrl Pts',(-0.13237211154771,1.,-2.06735123910326));
#31880=CARTESIAN_POINT('Ctrl Pts',(-0.134598026192106,-1.,-2.06155781517842));
#31881=CARTESIAN_POINT('Ctrl Pts',(-0.134598026192106,1.,-2.06155781517842));
#31882=CARTESIAN_POINT('Ctrl Pts',(-0.136777941218044,-1.,-2.05576044414264));
#31883=CARTESIAN_POINT('Ctrl Pts',(-0.136777941218044,1.,-2.05576044414264));
#31884=CARTESIAN_POINT('Ctrl Pts',(-0.138911255368966,-1.,-2.04995762001328));
#31885=CARTESIAN_POINT('Ctrl Pts',(-0.138911255368966,1.,-2.04995762001328));
#31886=CARTESIAN_POINT('Ctrl Pts',(-0.140997332152546,-1.,-2.04414757947916));
#31887=CARTESIAN_POINT('Ctrl Pts',(-0.140997332152546,1.,-2.04414757947916));
#31888=CARTESIAN_POINT('Ctrl Pts',(-0.143035515058209,-1.,-2.03832911025912));
#31889=CARTESIAN_POINT('Ctrl Pts',(-0.143035515058209,1.,-2.03832911025912));
#31890=CARTESIAN_POINT('Ctrl Pts',(-0.145025140186057,-1.,-2.03250223739942));
#31891=CARTESIAN_POINT('Ctrl Pts',(-0.145025140186057,1.,-2.03250223739942));
#31892=CARTESIAN_POINT('Ctrl Pts',(-0.146965557332583,-1.,-2.02666926182017));
#31893=CARTESIAN_POINT('Ctrl Pts',(-0.146965557332583,1.,-2.02666926182017));
#31894=CARTESIAN_POINT('Ctrl Pts',(-0.148856124775337,-1.,-2.02083464969894));
#31895=CARTESIAN_POINT('Ctrl Pts',(-0.148856124775337,1.,-2.02083464969894));
#31896=CARTESIAN_POINT('Ctrl Pts',(-0.150696157673078,-1.,-2.01500291940238));
#31897=CARTESIAN_POINT('Ctrl Pts',(-0.150696157673078,1.,-2.01500291940238));
#31898=CARTESIAN_POINT('Ctrl Pts',(-0.15248488362145,-1.,-2.00917680318424));
#31899=CARTESIAN_POINT('Ctrl Pts',(-0.15248488362145,1.,-2.00917680318424));
#31900=CARTESIAN_POINT('Ctrl Pts',(-0.154221403049722,-1.,-2.00335565310543));
#31901=CARTESIAN_POINT('Ctrl Pts',(-0.154221403049722,1.,-2.00335565310543));
#31902=CARTESIAN_POINT('Ctrl Pts',(-0.155904629548783,-1.,-1.99753284771497));
#31903=CARTESIAN_POINT('Ctrl Pts',(-0.155904629548783,1.,-1.99753284771497));
#31904=CARTESIAN_POINT('Ctrl Pts',(-0.157533331459227,-1.,-1.99169810931908));
#31905=CARTESIAN_POINT('Ctrl Pts',(-0.157533331459227,1.,-1.99169810931908));
#31906=CARTESIAN_POINT('Ctrl Pts',(-0.159106226437299,-1.,-1.98584238283292));
#31907=CARTESIAN_POINT('Ctrl Pts',(-0.159106226437299,1.,-1.98584238283292));
#31908=CARTESIAN_POINT('Ctrl Pts',(-0.160622060784611,-1.,-1.97996195437559));
#31909=CARTESIAN_POINT('Ctrl Pts',(-0.160622060784611,1.,-1.97996195437559));
#31910=CARTESIAN_POINT('Ctrl Pts',(-0.162079693556289,-1.,-1.97406280235188));
#31911=CARTESIAN_POINT('Ctrl Pts',(-0.162079693556289,1.,-1.97406280235188));
#31912=CARTESIAN_POINT('Ctrl Pts',(-0.163478185457734,-1.,-1.96816512677967));
#31913=CARTESIAN_POINT('Ctrl Pts',(-0.163478185457734,1.,-1.96816512677967));
#31914=CARTESIAN_POINT('Ctrl Pts',(-0.164816568920269,-1.,-1.96229379940136));
#31915=CARTESIAN_POINT('Ctrl Pts',(-0.164816568920269,1.,-1.96229379940136));
#31916=CARTESIAN_POINT('Ctrl Pts',(-0.166093592002812,-1.,-1.9564675971873));
#31917=CARTESIAN_POINT('Ctrl Pts',(-0.166093592002812,1.,-1.9564675971873));
#31918=CARTESIAN_POINT('Ctrl Pts',(-0.167307501784475,-1.,-1.95069027794294));
#31919=CARTESIAN_POINT('Ctrl Pts',(-0.167307501784475,1.,-1.95069027794294));
#31920=CARTESIAN_POINT('Ctrl Pts',(-0.168455741607556,-1.,-1.94493757756931));
#31921=CARTESIAN_POINT('Ctrl Pts',(-0.168455741607556,1.,-1.94493757756931));
#31922=CARTESIAN_POINT('Ctrl Pts',(-0.169534904817491,-1.,-1.93915639211581));
#31923=CARTESIAN_POINT('Ctrl Pts',(-0.169534904817491,1.,-1.93915639211581));
#31924=CARTESIAN_POINT('Ctrl Pts',(-0.170541253116202,-1.,-1.93329183155539));
#31925=CARTESIAN_POINT('Ctrl Pts',(-0.170541253116202,1.,-1.93329183155539));
#31926=CARTESIAN_POINT('Ctrl Pts',(-0.171471191532988,-1.,-1.92731093582036));
#31927=CARTESIAN_POINT('Ctrl Pts',(-0.171471191532988,1.,-1.92731093582036));
#31928=CARTESIAN_POINT('Ctrl Pts',(-0.172321621259514,-1.,-1.9212233439798));
#31929=CARTESIAN_POINT('Ctrl Pts',(-0.172321621259514,1.,-1.9212233439798));
#31930=CARTESIAN_POINT('Ctrl Pts',(-0.173090695383496,-1.,-1.91511429159527));
#31931=CARTESIAN_POINT('Ctrl Pts',(-0.173090695383496,1.,-1.91511429159527));
#31932=CARTESIAN_POINT('Ctrl Pts',(-0.173776635257817,-1.,-1.90911693975267));
#31933=CARTESIAN_POINT('Ctrl Pts',(-0.173776635257817,1.,-1.90911693975267));
#31934=CARTESIAN_POINT('Ctrl Pts',(-0.174375518661085,-1.,-1.90335253862834));
#31935=CARTESIAN_POINT('Ctrl Pts',(-0.174375518661085,1.,-1.90335253862834));
#31936=CARTESIAN_POINT('Ctrl Pts',(-0.174879405091263,-1.,-1.89788101117132));
#31937=CARTESIAN_POINT('Ctrl Pts',(-0.174879405091263,1.,-1.89788101117132));
#31938=CARTESIAN_POINT('Ctrl Pts',(-0.175274276190844,-1.,-1.892646301985));
#31939=CARTESIAN_POINT('Ctrl Pts',(-0.175274276190844,1.,-1.892646301985));
#31940=CARTESIAN_POINT('Ctrl Pts',(-0.175538155840648,-1.,-1.88742606273259));
#31941=CARTESIAN_POINT('Ctrl Pts',(-0.175538155840648,1.,-1.88742606273259));
#31942=CARTESIAN_POINT('Ctrl Pts',(-0.175644148889699,-1.,-1.88188663145367));
#31943=CARTESIAN_POINT('Ctrl Pts',(-0.175644148889699,1.,-1.88188663145367));
#31944=CARTESIAN_POINT('Ctrl Pts',(-0.175563480746485,-1.,-1.87563767773588));
#31945=CARTESIAN_POINT('Ctrl Pts',(-0.175563480746485,1.,-1.87563767773588));
#31946=CARTESIAN_POINT('Ctrl Pts',(-0.175268337590758,-1.,-1.86828349694799));
#31947=CARTESIAN_POINT('Ctrl Pts',(-0.175268337590758,1.,-1.86828349694799));
#31948=CARTESIAN_POINT('Ctrl Pts',(-0.17473525927603,-1.,-1.85948367088837));
#31949=CARTESIAN_POINT('Ctrl Pts',(-0.17473525927603,1.,-1.85948367088837));
#31950=CARTESIAN_POINT('Ctrl Pts',(-0.173946627587731,-1.,-1.8489811319852));
#31951=CARTESIAN_POINT('Ctrl Pts',(-0.173946627587731,1.,-1.8489811319852));
#31952=CARTESIAN_POINT('Ctrl Pts',(-0.1728894428919,-1.,-1.83658380527692));
#31953=CARTESIAN_POINT('Ctrl Pts',(-0.1728894428919,1.,-1.83658380527692));
#31954=CARTESIAN_POINT('Ctrl Pts',(-0.171554770204119,-1.,-1.82215766811545));
#31955=CARTESIAN_POINT('Ctrl Pts',(-0.171554770204119,1.,-1.82215766811545));
#31956=CARTESIAN_POINT('Ctrl Pts',(-0.169936923904608,-1.,-1.80561530629706));
#31957=CARTESIAN_POINT('Ctrl Pts',(-0.169936923904608,1.,-1.80561530629706));
#31958=CARTESIAN_POINT('Ctrl Pts',(-0.168032772805197,-1.,-1.7869064998507));
#31959=CARTESIAN_POINT('Ctrl Pts',(-0.168032772805197,1.,-1.7869064998507));
#31960=CARTESIAN_POINT('Ctrl Pts',(-0.1662793551464,-1.,-1.77018771684844));
#31961=CARTESIAN_POINT('Ctrl Pts',(-0.1662793551464,1.,-1.77018771684844));
#31962=CARTESIAN_POINT('Ctrl Pts',(-0.164834765707158,-1.,-1.75666056638427));
#31963=CARTESIAN_POINT('Ctrl Pts',(-0.164834765707158,1.,-1.75666056638427));
#31964=CARTESIAN_POINT('Ctrl Pts',(-0.163814161002002,-1.,-1.7472034950333));
#31965=CARTESIAN_POINT('Ctrl Pts',(-0.163814161002002,1.,-1.7472034950333));
#31966=CARTESIAN_POINT('Ctrl Pts',(-0.163289472382896,-1.,-1.74236521665491));
#31967=CARTESIAN_POINT('Ctrl Pts',(-0.163289472382896,1.,-1.74236521665491));
#31968=CARTESIAN_POINT('',(-0.0694764450219581,1.,-2.19890268624765));
#31969=CARTESIAN_POINT('Ctrl Pts',(-0.0694764450219581,1.,-2.19890268624765));
#31970=CARTESIAN_POINT('Ctrl Pts',(-0.070114353632549,1.,-2.19777582085423));
#31971=CARTESIAN_POINT('Ctrl Pts',(-0.0713863779526154,1.,-2.19552129484002));
#31972=CARTESIAN_POINT('Ctrl Pts',(-0.0732830357306725,1.,-2.19213712013662));
#31973=CARTESIAN_POINT('Ctrl Pts',(-0.0757891465836148,1.,-2.1876201139953));
#31974=CARTESIAN_POINT('Ctrl Pts',(-0.0788837727685243,1.,-2.18196589448887));
#31975=CARTESIAN_POINT('Ctrl Pts',(-0.0819402680872765,1.,-2.176303712113));
#31976=CARTESIAN_POINT('Ctrl Pts',(-0.0849584620835372,1.,-2.17063357870952));
#31977=CARTESIAN_POINT('Ctrl Pts',(-0.0879381291386923,1.,-2.16495552645014));
#31978=CARTESIAN_POINT('Ctrl Pts',(-0.0908789888107265,1.,-2.15926961544516));
#31979=CARTESIAN_POINT('Ctrl Pts',(-0.0937807218867643,1.,-2.1535759397817));
#31980=CARTESIAN_POINT('Ctrl Pts',(-0.0966429852305459,1.,-2.14787463531795));
#31981=CARTESIAN_POINT('Ctrl Pts',(-0.0994654261990915,1.,-2.14216588396025));
#31982=CARTESIAN_POINT('Ctrl Pts',(-0.1022477005561,1.,-2.13644992667165));
#31983=CARTESIAN_POINT('Ctrl Pts',(-0.104989479152739,1.,-2.13072704887293));
#31984=CARTESIAN_POINT('Ctrl Pts',(-0.10769043523109,1.,-2.12499752307));
#31985=CARTESIAN_POINT('Ctrl Pts',(-0.110350236135025,1.,-2.11926155590865));
#31986=CARTESIAN_POINT('Ctrl Pts',(-0.112968534419737,1.,-2.11351924490306));
#31987=CARTESIAN_POINT('Ctrl Pts',(-0.115544957687926,1.,-2.10777050261309));
#31988=CARTESIAN_POINT('Ctrl Pts',(-0.118079107988355,1.,-2.102015121329));
#31989=CARTESIAN_POINT('Ctrl Pts',(-0.120570567965122,1.,-2.0962529286773));
#31990=CARTESIAN_POINT('Ctrl Pts',(-0.123018905621083,1.,-2.09048392424825));
#31991=CARTESIAN_POINT('Ctrl Pts',(-0.125423679412061,1.,-2.08470840653643));
#31992=CARTESIAN_POINT('Ctrl Pts',(-0.12778444527612,1.,-2.07892715110987));
#31993=CARTESIAN_POINT('Ctrl Pts',(-0.130100748328403,1.,-2.07314114713063));
#31994=CARTESIAN_POINT('Ctrl Pts',(-0.13237211154771,1.,-2.06735123910326));
#31995=CARTESIAN_POINT('Ctrl Pts',(-0.134598026192106,1.,-2.06155781517842));
#31996=CARTESIAN_POINT('Ctrl Pts',(-0.136777941218044,1.,-2.05576044414264));
#31997=CARTESIAN_POINT('Ctrl Pts',(-0.138911255368966,1.,-2.04995762001328));
#31998=CARTESIAN_POINT('Ctrl Pts',(-0.140997332152546,1.,-2.04414757947916));
#31999=CARTESIAN_POINT('Ctrl Pts',(-0.143035515058209,1.,-2.03832911025912));
#32000=CARTESIAN_POINT('Ctrl Pts',(-0.145025140186057,1.,-2.03250223739942));
#32001=CARTESIAN_POINT('Ctrl Pts',(-0.146965557332583,1.,-2.02666926182017));
#32002=CARTESIAN_POINT('Ctrl Pts',(-0.148856124775337,1.,-2.02083464969894));
#32003=CARTESIAN_POINT('Ctrl Pts',(-0.150696157673078,1.,-2.01500291940238));
#32004=CARTESIAN_POINT('Ctrl Pts',(-0.15248488362145,1.,-2.00917680318424));
#32005=CARTESIAN_POINT('Ctrl Pts',(-0.154221403049722,1.,-2.00335565310543));
#32006=CARTESIAN_POINT('Ctrl Pts',(-0.155904629548783,1.,-1.99753284771497));
#32007=CARTESIAN_POINT('Ctrl Pts',(-0.157533331459227,1.,-1.99169810931908));
#32008=CARTESIAN_POINT('Ctrl Pts',(-0.159106226437299,1.,-1.98584238283292));
#32009=CARTESIAN_POINT('Ctrl Pts',(-0.160622060784611,1.,-1.97996195437559));
#32010=CARTESIAN_POINT('Ctrl Pts',(-0.162079693556289,1.,-1.97406280235188));
#32011=CARTESIAN_POINT('Ctrl Pts',(-0.163478185457734,1.,-1.96816512677967));
#32012=CARTESIAN_POINT('Ctrl Pts',(-0.164816568920269,1.,-1.96229379940136));
#32013=CARTESIAN_POINT('Ctrl Pts',(-0.166093592002812,1.,-1.9564675971873));
#32014=CARTESIAN_POINT('Ctrl Pts',(-0.167307501784475,1.,-1.95069027794294));
#32015=CARTESIAN_POINT('Ctrl Pts',(-0.168455741607556,1.,-1.94493757756931));
#32016=CARTESIAN_POINT('Ctrl Pts',(-0.169534904817491,1.,-1.93915639211581));
#32017=CARTESIAN_POINT('Ctrl Pts',(-0.170541253116202,1.,-1.93329183155539));
#32018=CARTESIAN_POINT('Ctrl Pts',(-0.171471191532988,1.,-1.92731093582036));
#32019=CARTESIAN_POINT('Ctrl Pts',(-0.172321621259514,1.,-1.9212233439798));
#32020=CARTESIAN_POINT('Ctrl Pts',(-0.173090695383496,1.,-1.91511429159527));
#32021=CARTESIAN_POINT('Ctrl Pts',(-0.173776635257817,1.,-1.90911693975267));
#32022=CARTESIAN_POINT('Ctrl Pts',(-0.174375518661085,1.,-1.90335253862834));
#32023=CARTESIAN_POINT('Ctrl Pts',(-0.174879405091263,1.,-1.89788101117132));
#32024=CARTESIAN_POINT('Ctrl Pts',(-0.175274276190844,1.,-1.892646301985));
#32025=CARTESIAN_POINT('Ctrl Pts',(-0.175538155840648,1.,-1.88742606273259));
#32026=CARTESIAN_POINT('Ctrl Pts',(-0.175644148889699,1.,-1.88188663145367));
#32027=CARTESIAN_POINT('Ctrl Pts',(-0.175563480746485,1.,-1.87563767773588));
#32028=CARTESIAN_POINT('Ctrl Pts',(-0.175268337590758,1.,-1.86828349694799));
#32029=CARTESIAN_POINT('Ctrl Pts',(-0.17473525927603,1.,-1.85948367088837));
#32030=CARTESIAN_POINT('Ctrl Pts',(-0.173946627587731,1.,-1.8489811319852));
#32031=CARTESIAN_POINT('Ctrl Pts',(-0.1728894428919,1.,-1.83658380527692));
#32032=CARTESIAN_POINT('Ctrl Pts',(-0.171554770204119,1.,-1.82215766811545));
#32033=CARTESIAN_POINT('Ctrl Pts',(-0.169936923904608,1.,-1.80561530629706));
#32034=CARTESIAN_POINT('Ctrl Pts',(-0.168032772805197,1.,-1.7869064998507));
#32035=CARTESIAN_POINT('Ctrl Pts',(-0.1662793551464,1.,-1.77018771684844));
#32036=CARTESIAN_POINT('Ctrl Pts',(-0.164834765707158,1.,-1.75666056638427));
#32037=CARTESIAN_POINT('Ctrl Pts',(-0.163814161002002,1.,-1.7472034950333));
#32038=CARTESIAN_POINT('Ctrl Pts',(-0.163289472382896,1.,-1.74236521665491));
#32039=CARTESIAN_POINT('',(-0.0694764450219581,0.,-2.19890268624765));
#32040=CARTESIAN_POINT('Origin',(0.0694764450219584,0.,-2.19890268624765));
#32041=CARTESIAN_POINT('',(0.0694764450219584,1.,-2.19890268624765));
#32042=CARTESIAN_POINT('',(-0.0694764450219581,1.,-2.19890268624765));
#32043=CARTESIAN_POINT('',(0.0694764450219584,0.,-2.19890268624765));
#32044=CARTESIAN_POINT('Ctrl Pts',(0.163289472382896,-1.,-1.74236521665491));
#32045=CARTESIAN_POINT('Ctrl Pts',(0.163289472382896,1.,-1.74236521665491));
#32046=CARTESIAN_POINT('Ctrl Pts',(0.163814161002474,-1.,-1.74720349503904));
#32047=CARTESIAN_POINT('Ctrl Pts',(0.163814161002474,1.,-1.74720349503904));
#32048=CARTESIAN_POINT('Ctrl Pts',(0.164834765708484,-1.,-1.75666056640041));
#32049=CARTESIAN_POINT('Ctrl Pts',(0.164834765708484,1.,-1.75666056640041));
#32050=CARTESIAN_POINT('Ctrl Pts',(0.166279355148738,-1.,-1.77018771687692));
#32051=CARTESIAN_POINT('Ctrl Pts',(0.166279355148738,1.,-1.77018771687692));
#32052=CARTESIAN_POINT('Ctrl Pts',(0.16803277280837,-1.,-1.78690649988931));
#32053=CARTESIAN_POINT('Ctrl Pts',(0.16803277280837,1.,-1.78690649988931));
#32054=CARTESIAN_POINT('Ctrl Pts',(0.169936923908078,-1.,-1.80561530633924));
#32055=CARTESIAN_POINT('Ctrl Pts',(0.169936923908078,1.,-1.80561530633924));
#32056=CARTESIAN_POINT('Ctrl Pts',(0.171554770207306,-1.,-1.82215766815414));
#32057=CARTESIAN_POINT('Ctrl Pts',(0.171554770207306,1.,-1.82215766815414));
#32058=CARTESIAN_POINT('Ctrl Pts',(0.17288944289442,-1.,-1.83658380530747));
#32059=CARTESIAN_POINT('Ctrl Pts',(0.17288944289442,1.,-1.83658380530747));
#32060=CARTESIAN_POINT('Ctrl Pts',(0.173946627589401,-1.,-1.84898113200543));
#32061=CARTESIAN_POINT('Ctrl Pts',(0.173946627589401,1.,-1.84898113200543));
#32062=CARTESIAN_POINT('Ctrl Pts',(0.174735259276856,-1.,-1.85948367089838));
#32063=CARTESIAN_POINT('Ctrl Pts',(0.174735259276856,1.,-1.85948367089838));
#32064=CARTESIAN_POINT('Ctrl Pts',(0.175268337590901,-1.,-1.86828349694972));
#32065=CARTESIAN_POINT('Ctrl Pts',(0.175268337590901,1.,-1.86828349694972));
#32066=CARTESIAN_POINT('Ctrl Pts',(0.175563480746205,-1.,-1.87563767773249));
#32067=CARTESIAN_POINT('Ctrl Pts',(0.175563480746205,1.,-1.87563767773249));
#32068=CARTESIAN_POINT('Ctrl Pts',(0.175644148889271,-1.,-1.88188663144846));
#32069=CARTESIAN_POINT('Ctrl Pts',(0.175644148889271,1.,-1.88188663144846));
#32070=CARTESIAN_POINT('Ctrl Pts',(0.175538155840286,-1.,-1.88742606272818));
#32071=CARTESIAN_POINT('Ctrl Pts',(0.175538155840286,1.,-1.88742606272818));
#32072=CARTESIAN_POINT('Ctrl Pts',(0.175274276190664,-1.,-1.89264630198279));
#32073=CARTESIAN_POINT('Ctrl Pts',(0.175274276190664,1.,-1.89264630198279));
#32074=CARTESIAN_POINT('Ctrl Pts',(0.174879405091277,-1.,-1.89788101117148));
#32075=CARTESIAN_POINT('Ctrl Pts',(0.174879405091277,1.,-1.89788101117148));
#32076=CARTESIAN_POINT('Ctrl Pts',(0.174375518661222,-1.,-1.90335253863003));
#32077=CARTESIAN_POINT('Ctrl Pts',(0.174375518661222,1.,-1.90335253863003));
#32078=CARTESIAN_POINT('Ctrl Pts',(0.173776635257984,-1.,-1.90911693975475));
#32079=CARTESIAN_POINT('Ctrl Pts',(0.173776635257984,1.,-1.90911693975475));
#32080=CARTESIAN_POINT('Ctrl Pts',(0.173090695383619,-1.,-1.91511429159681));
#32081=CARTESIAN_POINT('Ctrl Pts',(0.173090695383619,1.,-1.91511429159681));
#32082=CARTESIAN_POINT('Ctrl Pts',(0.172321621259557,-1.,-1.92122334398034));
#32083=CARTESIAN_POINT('Ctrl Pts',(0.172321621259557,1.,-1.92122334398034));
#32084=CARTESIAN_POINT('Ctrl Pts',(0.17147119153296,-1.,-1.92731093582));
#32085=CARTESIAN_POINT('Ctrl Pts',(0.17147119153296,1.,-1.92731093582));
#32086=CARTESIAN_POINT('Ctrl Pts',(0.170541253116136,-1.,-1.93329183155455));
#32087=CARTESIAN_POINT('Ctrl Pts',(0.170541253116136,1.,-1.93329183155455));
#32088=CARTESIAN_POINT('Ctrl Pts',(0.169534904817425,-1.,-1.93915639211497));
#32089=CARTESIAN_POINT('Ctrl Pts',(0.169534904817425,1.,-1.93915639211497));
#32090=CARTESIAN_POINT('Ctrl Pts',(0.168455741607516,-1.,-1.94493757756879));
#32091=CARTESIAN_POINT('Ctrl Pts',(0.168455741607516,1.,-1.94493757756879));
#32092=CARTESIAN_POINT('Ctrl Pts',(0.167307501784469,-1.,-1.95069027794286));
#32093=CARTESIAN_POINT('Ctrl Pts',(0.167307501784469,1.,-1.95069027794286));
#32094=CARTESIAN_POINT('Ctrl Pts',(0.166093592002833,-1.,-1.95646759718755));
#32095=CARTESIAN_POINT('Ctrl Pts',(0.166093592002833,1.,-1.95646759718755));
#32096=CARTESIAN_POINT('Ctrl Pts',(0.1648165689203,-1.,-1.96229379940174));
#32097=CARTESIAN_POINT('Ctrl Pts',(0.1648165689203,1.,-1.96229379940174));
#32098=CARTESIAN_POINT('Ctrl Pts',(0.16347818545776,-1.,-1.96816512678));
#32099=CARTESIAN_POINT('Ctrl Pts',(0.16347818545776,1.,-1.96816512678));
#32100=CARTESIAN_POINT('Ctrl Pts',(0.162079693556302,-1.,-1.97406280235204));
#32101=CARTESIAN_POINT('Ctrl Pts',(0.162079693556302,1.,-1.97406280235204));
#32102=CARTESIAN_POINT('Ctrl Pts',(0.16062206078461,-1.,-1.97996195437557));
#32103=CARTESIAN_POINT('Ctrl Pts',(0.16062206078461,1.,-1.97996195437557));
#32104=CARTESIAN_POINT('Ctrl Pts',(0.159106226437288,-1.,-1.98584238283279));
#32105=CARTESIAN_POINT('Ctrl Pts',(0.159106226437288,1.,-1.98584238283279));
#32106=CARTESIAN_POINT('Ctrl Pts',(0.157533331459215,-1.,-1.99169810931893));
#32107=CARTESIAN_POINT('Ctrl Pts',(0.157533331459215,1.,-1.99169810931893));
#32108=CARTESIAN_POINT('Ctrl Pts',(0.155904629548774,-1.,-1.99753284771487));
#32109=CARTESIAN_POINT('Ctrl Pts',(0.155904629548774,1.,-1.99753284771487));
#32110=CARTESIAN_POINT('Ctrl Pts',(0.154221403049719,-1.,-2.00335565310539));
#32111=CARTESIAN_POINT('Ctrl Pts',(0.154221403049719,1.,-2.00335565310539));
#32112=CARTESIAN_POINT('Ctrl Pts',(0.152484883621452,-1.,-2.00917680318426));
#32113=CARTESIAN_POINT('Ctrl Pts',(0.152484883621452,1.,-2.00917680318426));
#32114=CARTESIAN_POINT('Ctrl Pts',(0.150696157673084,-1.,-2.01500291940243));
#32115=CARTESIAN_POINT('Ctrl Pts',(0.150696157673084,1.,-2.01500291940243));
#32116=CARTESIAN_POINT('Ctrl Pts',(0.148856124775343,-1.,-2.02083464969897));
#32117=CARTESIAN_POINT('Ctrl Pts',(0.148856124775343,1.,-2.02083464969897));
#32118=CARTESIAN_POINT('Ctrl Pts',(0.146965557332586,-1.,-2.02666926182017));
#32119=CARTESIAN_POINT('Ctrl Pts',(0.146965557332586,1.,-2.02666926182017));
#32120=CARTESIAN_POINT('Ctrl Pts',(0.145025140186058,-1.,-2.03250223739941));
#32121=CARTESIAN_POINT('Ctrl Pts',(0.145025140186058,1.,-2.03250223739941));
#32122=CARTESIAN_POINT('Ctrl Pts',(0.143035515058208,-1.,-2.03832911025913));
#32123=CARTESIAN_POINT('Ctrl Pts',(0.143035515058208,1.,-2.03832911025913));
#32124=CARTESIAN_POINT('Ctrl Pts',(0.140997332152545,-1.,-2.04414757947919));
#32125=CARTESIAN_POINT('Ctrl Pts',(0.140997332152545,1.,-2.04414757947919));
#32126=CARTESIAN_POINT('Ctrl Pts',(0.138911255368966,-1.,-2.04995762001333));
#32127=CARTESIAN_POINT('Ctrl Pts',(0.138911255368966,1.,-2.04995762001333));
#32128=CARTESIAN_POINT('Ctrl Pts',(0.136777941218044,-1.,-2.0557604441427));
#32129=CARTESIAN_POINT('Ctrl Pts',(0.136777941218044,1.,-2.0557604441427));
#32130=CARTESIAN_POINT('Ctrl Pts',(0.134598026192107,-1.,-2.06155781517844));
#32131=CARTESIAN_POINT('Ctrl Pts',(0.134598026192107,1.,-2.06155781517844));
#32132=CARTESIAN_POINT('Ctrl Pts',(0.13237211154771,-1.,-2.06735123910319));
#32133=CARTESIAN_POINT('Ctrl Pts',(0.13237211154771,1.,-2.06735123910319));
#32134=CARTESIAN_POINT('Ctrl Pts',(0.1301007483284,-1.,-2.07314114713047));
#32135=CARTESIAN_POINT('Ctrl Pts',(0.1301007483284,1.,-2.07314114713047));
#32136=CARTESIAN_POINT('Ctrl Pts',(0.127784445276116,-1.,-2.07892715110967));
#32137=CARTESIAN_POINT('Ctrl Pts',(0.127784445276116,1.,-2.07892715110967));
#32138=CARTESIAN_POINT('Ctrl Pts',(0.125423679412058,-1.,-2.08470840653628));
#32139=CARTESIAN_POINT('Ctrl Pts',(0.125423679412058,1.,-2.08470840653628));
#32140=CARTESIAN_POINT('Ctrl Pts',(0.123018905621083,-1.,-2.09048392424826));
#32141=CARTESIAN_POINT('Ctrl Pts',(0.123018905621083,1.,-2.09048392424826));
#32142=CARTESIAN_POINT('Ctrl Pts',(0.120570567965129,-1.,-2.09625292867756));
#32143=CARTESIAN_POINT('Ctrl Pts',(0.120570567965129,1.,-2.09625292867756));
#32144=CARTESIAN_POINT('Ctrl Pts',(0.118079107988368,-1.,-2.10201512132945));
#32145=CARTESIAN_POINT('Ctrl Pts',(0.118079107988368,1.,-2.10201512132945));
#32146=CARTESIAN_POINT('Ctrl Pts',(0.11554495768794,-1.,-2.10777050261359));
#32147=CARTESIAN_POINT('Ctrl Pts',(0.11554495768794,1.,-2.10777050261359));
#32148=CARTESIAN_POINT('Ctrl Pts',(0.112968534419746,-1.,-2.11351924490335));
#32149=CARTESIAN_POINT('Ctrl Pts',(0.112968534419746,1.,-2.11351924490335));
#32150=CARTESIAN_POINT('Ctrl Pts',(0.11035023613502,-1.,-2.11926155590849));
#32151=CARTESIAN_POINT('Ctrl Pts',(0.11035023613502,1.,-2.11926155590849));
#32152=CARTESIAN_POINT('Ctrl Pts',(0.107690435231068,-1.,-2.12499752306927));
#32153=CARTESIAN_POINT('Ctrl Pts',(0.107690435231068,1.,-2.12499752306927));
#32154=CARTESIAN_POINT('Ctrl Pts',(0.104989479152703,-1.,-2.1307270488718));
#32155=CARTESIAN_POINT('Ctrl Pts',(0.104989479152703,1.,-2.1307270488718));
#32156=CARTESIAN_POINT('Ctrl Pts',(0.102247700556064,-1.,-2.13644992667052));
#32157=CARTESIAN_POINT('Ctrl Pts',(0.102247700556064,1.,-2.13644992667052));
#32158=CARTESIAN_POINT('Ctrl Pts',(0.0994654261990743,-1.,-2.14216588395974));
#32159=CARTESIAN_POINT('Ctrl Pts',(0.0994654261990743,1.,-2.14216588395974));
#32160=CARTESIAN_POINT('Ctrl Pts',(0.0966429852305689,-1.,-2.14787463531864));
#32161=CARTESIAN_POINT('Ctrl Pts',(0.0966429852305689,1.,-2.14787463531864));
#32162=CARTESIAN_POINT('Ctrl Pts',(0.0937807218868345,-1.,-2.15357593978377));
#32163=CARTESIAN_POINT('Ctrl Pts',(0.0937807218868345,1.,-2.15357593978377));
#32164=CARTESIAN_POINT('Ctrl Pts',(0.0908789888108266,-1.,-2.15926961544808));
#32165=CARTESIAN_POINT('Ctrl Pts',(0.0908789888108266,1.,-2.15926961544808));
#32166=CARTESIAN_POINT('Ctrl Pts',(0.0879381291387823,-1.,-2.16495552645275));
#32167=CARTESIAN_POINT('Ctrl Pts',(0.0879381291387823,1.,-2.16495552645275));
#32168=CARTESIAN_POINT('Ctrl Pts',(0.0849584620835643,-1.,-2.17063357871031));
#32169=CARTESIAN_POINT('Ctrl Pts',(0.0849584620835643,1.,-2.17063357871031));
#32170=CARTESIAN_POINT('Ctrl Pts',(0.0819402680871939,-1.,-2.1763037121106));
#32171=CARTESIAN_POINT('Ctrl Pts',(0.0819402680871939,1.,-2.1763037121106));
#32172=CARTESIAN_POINT('Ctrl Pts',(0.0788837727683228,-1.,-2.18196589448304));
#32173=CARTESIAN_POINT('Ctrl Pts',(0.0788837727683228,1.,-2.18196589448304));
#32174=CARTESIAN_POINT('Ctrl Pts',(0.0757891465833411,-1.,-2.1876201139874));
#32175=CARTESIAN_POINT('Ctrl Pts',(0.0757891465833411,1.,-2.1876201139874));
#32176=CARTESIAN_POINT('Ctrl Pts',(0.0732830357304276,-1.,-2.19213712012956));
#32177=CARTESIAN_POINT('Ctrl Pts',(0.0732830357304276,1.,-2.19213712012956));
#32178=CARTESIAN_POINT('Ctrl Pts',(0.0713863779524627,-1.,-2.19552129483562));
#32179=CARTESIAN_POINT('Ctrl Pts',(0.0713863779524627,1.,-2.19552129483562));
#32180=CARTESIAN_POINT('Ctrl Pts',(0.0701143536324926,-1.,-2.19777582085261));
#32181=CARTESIAN_POINT('Ctrl Pts',(0.0701143536324926,1.,-2.19777582085261));
#32182=CARTESIAN_POINT('Ctrl Pts',(0.0694764450219584,-1.,-2.19890268624765));
#32183=CARTESIAN_POINT('Ctrl Pts',(0.0694764450219584,1.,-2.19890268624765));
#32184=CARTESIAN_POINT('',(0.163289472382896,1.,-1.74236521665491));
#32185=CARTESIAN_POINT('Ctrl Pts',(0.163289472382896,1.,-1.74236521665491));
#32186=CARTESIAN_POINT('Ctrl Pts',(0.163814161002474,1.,-1.74720349503904));
#32187=CARTESIAN_POINT('Ctrl Pts',(0.164834765708484,1.,-1.75666056640041));
#32188=CARTESIAN_POINT('Ctrl Pts',(0.166279355148738,1.,-1.77018771687692));
#32189=CARTESIAN_POINT('Ctrl Pts',(0.16803277280837,1.,-1.78690649988931));
#32190=CARTESIAN_POINT('Ctrl Pts',(0.169936923908078,1.,-1.80561530633924));
#32191=CARTESIAN_POINT('Ctrl Pts',(0.171554770207306,1.,-1.82215766815414));
#32192=CARTESIAN_POINT('Ctrl Pts',(0.17288944289442,1.,-1.83658380530747));
#32193=CARTESIAN_POINT('Ctrl Pts',(0.173946627589401,1.,-1.84898113200543));
#32194=CARTESIAN_POINT('Ctrl Pts',(0.174735259276856,1.,-1.85948367089838));
#32195=CARTESIAN_POINT('Ctrl Pts',(0.175268337590901,1.,-1.86828349694972));
#32196=CARTESIAN_POINT('Ctrl Pts',(0.175563480746205,1.,-1.87563767773249));
#32197=CARTESIAN_POINT('Ctrl Pts',(0.175644148889271,1.,-1.88188663144846));
#32198=CARTESIAN_POINT('Ctrl Pts',(0.175538155840286,1.,-1.88742606272818));
#32199=CARTESIAN_POINT('Ctrl Pts',(0.175274276190664,1.,-1.89264630198279));
#32200=CARTESIAN_POINT('Ctrl Pts',(0.174879405091277,1.,-1.89788101117148));
#32201=CARTESIAN_POINT('Ctrl Pts',(0.174375518661222,1.,-1.90335253863003));
#32202=CARTESIAN_POINT('Ctrl Pts',(0.173776635257984,1.,-1.90911693975475));
#32203=CARTESIAN_POINT('Ctrl Pts',(0.173090695383619,1.,-1.91511429159681));
#32204=CARTESIAN_POINT('Ctrl Pts',(0.172321621259557,1.,-1.92122334398034));
#32205=CARTESIAN_POINT('Ctrl Pts',(0.17147119153296,1.,-1.92731093582));
#32206=CARTESIAN_POINT('Ctrl Pts',(0.170541253116136,1.,-1.93329183155455));
#32207=CARTESIAN_POINT('Ctrl Pts',(0.169534904817425,1.,-1.93915639211497));
#32208=CARTESIAN_POINT('Ctrl Pts',(0.168455741607516,1.,-1.94493757756879));
#32209=CARTESIAN_POINT('Ctrl Pts',(0.167307501784469,1.,-1.95069027794286));
#32210=CARTESIAN_POINT('Ctrl Pts',(0.166093592002833,1.,-1.95646759718755));
#32211=CARTESIAN_POINT('Ctrl Pts',(0.1648165689203,1.,-1.96229379940174));
#32212=CARTESIAN_POINT('Ctrl Pts',(0.16347818545776,1.,-1.96816512678));
#32213=CARTESIAN_POINT('Ctrl Pts',(0.162079693556302,1.,-1.97406280235204));
#32214=CARTESIAN_POINT('Ctrl Pts',(0.16062206078461,1.,-1.97996195437557));
#32215=CARTESIAN_POINT('Ctrl Pts',(0.159106226437288,1.,-1.98584238283279));
#32216=CARTESIAN_POINT('Ctrl Pts',(0.157533331459215,1.,-1.99169810931893));
#32217=CARTESIAN_POINT('Ctrl Pts',(0.155904629548774,1.,-1.99753284771487));
#32218=CARTESIAN_POINT('Ctrl Pts',(0.154221403049719,1.,-2.00335565310539));
#32219=CARTESIAN_POINT('Ctrl Pts',(0.152484883621452,1.,-2.00917680318426));
#32220=CARTESIAN_POINT('Ctrl Pts',(0.150696157673084,1.,-2.01500291940243));
#32221=CARTESIAN_POINT('Ctrl Pts',(0.148856124775343,1.,-2.02083464969897));
#32222=CARTESIAN_POINT('Ctrl Pts',(0.146965557332586,1.,-2.02666926182017));
#32223=CARTESIAN_POINT('Ctrl Pts',(0.145025140186058,1.,-2.03250223739941));
#32224=CARTESIAN_POINT('Ctrl Pts',(0.143035515058208,1.,-2.03832911025913));
#32225=CARTESIAN_POINT('Ctrl Pts',(0.140997332152545,1.,-2.04414757947919));
#32226=CARTESIAN_POINT('Ctrl Pts',(0.138911255368966,1.,-2.04995762001333));
#32227=CARTESIAN_POINT('Ctrl Pts',(0.136777941218044,1.,-2.0557604441427));
#32228=CARTESIAN_POINT('Ctrl Pts',(0.134598026192107,1.,-2.06155781517844));
#32229=CARTESIAN_POINT('Ctrl Pts',(0.13237211154771,1.,-2.06735123910319));
#32230=CARTESIAN_POINT('Ctrl Pts',(0.1301007483284,1.,-2.07314114713047));
#32231=CARTESIAN_POINT('Ctrl Pts',(0.127784445276116,1.,-2.07892715110967));
#32232=CARTESIAN_POINT('Ctrl Pts',(0.125423679412058,1.,-2.08470840653628));
#32233=CARTESIAN_POINT('Ctrl Pts',(0.123018905621083,1.,-2.09048392424826));
#32234=CARTESIAN_POINT('Ctrl Pts',(0.120570567965129,1.,-2.09625292867756));
#32235=CARTESIAN_POINT('Ctrl Pts',(0.118079107988368,1.,-2.10201512132945));
#32236=CARTESIAN_POINT('Ctrl Pts',(0.11554495768794,1.,-2.10777050261359));
#32237=CARTESIAN_POINT('Ctrl Pts',(0.112968534419746,1.,-2.11351924490335));
#32238=CARTESIAN_POINT('Ctrl Pts',(0.11035023613502,1.,-2.11926155590849));
#32239=CARTESIAN_POINT('Ctrl Pts',(0.107690435231068,1.,-2.12499752306927));
#32240=CARTESIAN_POINT('Ctrl Pts',(0.104989479152703,1.,-2.1307270488718));
#32241=CARTESIAN_POINT('Ctrl Pts',(0.102247700556064,1.,-2.13644992667052));
#32242=CARTESIAN_POINT('Ctrl Pts',(0.0994654261990743,1.,-2.14216588395974));
#32243=CARTESIAN_POINT('Ctrl Pts',(0.0966429852305689,1.,-2.14787463531864));
#32244=CARTESIAN_POINT('Ctrl Pts',(0.0937807218868345,1.,-2.15357593978377));
#32245=CARTESIAN_POINT('Ctrl Pts',(0.0908789888108266,1.,-2.15926961544808));
#32246=CARTESIAN_POINT('Ctrl Pts',(0.0879381291387823,1.,-2.16495552645275));
#32247=CARTESIAN_POINT('Ctrl Pts',(0.0849584620835643,1.,-2.17063357871031));
#32248=CARTESIAN_POINT('Ctrl Pts',(0.0819402680871939,1.,-2.1763037121106));
#32249=CARTESIAN_POINT('Ctrl Pts',(0.0788837727683228,1.,-2.18196589448304));
#32250=CARTESIAN_POINT('Ctrl Pts',(0.0757891465833411,1.,-2.1876201139874));
#32251=CARTESIAN_POINT('Ctrl Pts',(0.0732830357304276,1.,-2.19213712012956));
#32252=CARTESIAN_POINT('Ctrl Pts',(0.0713863779524627,1.,-2.19552129483562));
#32253=CARTESIAN_POINT('Ctrl Pts',(0.0701143536324926,1.,-2.19777582085261));
#32254=CARTESIAN_POINT('Ctrl Pts',(0.0694764450219584,1.,-2.19890268624765));
#32255=CARTESIAN_POINT('',(0.163289472382896,0.,-1.74236521665491));
#32256=CARTESIAN_POINT('Origin',(0.,0.,0.));
#32257=CARTESIAN_POINT('',(0.383122945602004,1.,-1.7075470150345));
#32258=CARTESIAN_POINT('Origin',(0.,1.,0.));
#32259=CARTESIAN_POINT('',(0.383122945602004,0.,-1.7075470150345));
#32260=CARTESIAN_POINT('Ctrl Pts',(0.61342227326009,-1.,-2.11275013067528));
#32261=CARTESIAN_POINT('Ctrl Pts',(0.61342227326009,1.,-2.11275013067528));
#32262=CARTESIAN_POINT('Ctrl Pts',(0.61246736556225,-1.,-2.11187554260142));
#32263=CARTESIAN_POINT('Ctrl Pts',(0.61246736556225,1.,-2.11187554260142));
#32264=CARTESIAN_POINT('Ctrl Pts',(0.610560911691113,-1.,-2.11012443807661));
#32265=CARTESIAN_POINT('Ctrl Pts',(0.610560911691113,1.,-2.11012443807661));
#32266=CARTESIAN_POINT('Ctrl Pts',(0.607711315456826,-1.,-2.10749199615859));
#32267=CARTESIAN_POINT('Ctrl Pts',(0.607711315456826,1.,-2.10749199615859));
#32268=CARTESIAN_POINT('Ctrl Pts',(0.603932030738212,-1.,-2.10397049887709));
#32269=CARTESIAN_POINT('Ctrl Pts',(0.603932030738212,1.,-2.10397049887709));
#32270=CARTESIAN_POINT('Ctrl Pts',(0.599241616422144,-1.,-2.09954930865331));
#32271=CARTESIAN_POINT('Ctrl Pts',(0.599241616422144,1.,-2.09954930865331));
#32272=CARTESIAN_POINT('Ctrl Pts',(0.594585006052823,-1.,-2.09510876220501));
#32273=CARTESIAN_POINT('Ctrl Pts',(0.594585006052823,1.,-2.09510876220501));
#32274=CARTESIAN_POINT('Ctrl Pts',(0.589962365403189,-1.,-2.09064881812053));
#32275=CARTESIAN_POINT('Ctrl Pts',(0.589962365403189,1.,-2.09064881812053));
#32276=CARTESIAN_POINT('Ctrl Pts',(0.585373918990895,-1.,-2.086169437277));
#32277=CARTESIAN_POINT('Ctrl Pts',(0.585373918990895,1.,-2.086169437277));
#32278=CARTESIAN_POINT('Ctrl Pts',(0.580819952107256,-1.,-2.08167059018138));
#32279=CARTESIAN_POINT('Ctrl Pts',(0.580819952107256,1.,-2.08167059018138));
#32280=CARTESIAN_POINT('Ctrl Pts',(0.576300797416274,-1.,-2.07715226767361));
#32281=CARTESIAN_POINT('Ctrl Pts',(0.576300797416274,1.,-2.07715226767361));
#32282=CARTESIAN_POINT('Ctrl Pts',(0.571816823242411,-1.,-2.07261449292758));
#32283=CARTESIAN_POINT('Ctrl Pts',(0.571816823242411,1.,-2.07261449292758));
#32284=CARTESIAN_POINT('Ctrl Pts',(0.567368421181229,-1.,-2.06805732997383));
#32285=CARTESIAN_POINT('Ctrl Pts',(0.567368421181229,1.,-2.06805732997383));
#32286=CARTESIAN_POINT('Ctrl Pts',(0.562955993082574,-1.,-2.06348090160697));
#32287=CARTESIAN_POINT('Ctrl Pts',(0.562955993082574,1.,-2.06348090160697));
#32288=CARTESIAN_POINT('Ctrl Pts',(0.558579940185467,-1.,-2.05888537756571));
#32289=CARTESIAN_POINT('Ctrl Pts',(0.558579940185467,1.,-2.05888537756571));
#32290=CARTESIAN_POINT('Ctrl Pts',(0.554240657464109,-1.,-2.05427091604482));
#32291=CARTESIAN_POINT('Ctrl Pts',(0.554240657464109,1.,-2.05427091604482));
#32292=CARTESIAN_POINT('Ctrl Pts',(0.549938525150342,-1.,-2.04963761077974));
#32293=CARTESIAN_POINT('Ctrl Pts',(0.549938525150342,1.,-2.04963761077974));
#32294=CARTESIAN_POINT('Ctrl Pts',(0.545673903817348,-1.,-2.0449854471456));
#32295=CARTESIAN_POINT('Ctrl Pts',(0.545673903817348,1.,-2.0449854471456));
#32296=CARTESIAN_POINT('Ctrl Pts',(0.54144712061552,-1.,-2.0403142269048));
#32297=CARTESIAN_POINT('Ctrl Pts',(0.54144712061552,1.,-2.0403142269048));
#32298=CARTESIAN_POINT('Ctrl Pts',(0.537258489833134,-1.,-2.03562362953993));
#32299=CARTESIAN_POINT('Ctrl Pts',(0.537258489833134,1.,-2.03562362953993));
#32300=CARTESIAN_POINT('Ctrl Pts',(0.533108355132905,-1.,-2.03091336214401));
#32301=CARTESIAN_POINT('Ctrl Pts',(0.533108355132905,1.,-2.03091336214401));
#32302=CARTESIAN_POINT('Ctrl Pts',(0.52899712724191,-1.,-2.02618329083289));
#32303=CARTESIAN_POINT('Ctrl Pts',(0.52899712724191,1.,-2.02618329083289));
#32304=CARTESIAN_POINT('Ctrl Pts',(0.524925318333518,-1.,-2.02143356304712));
#32305=CARTESIAN_POINT('Ctrl Pts',(0.524925318333518,1.,-2.02143356304712));
#32306=CARTESIAN_POINT('Ctrl Pts',(0.520893590399428,-1.,-2.01666477917306));
#32307=CARTESIAN_POINT('Ctrl Pts',(0.520893590399428,1.,-2.01666477917306));
#32308=CARTESIAN_POINT('Ctrl Pts',(0.516902681728733,-1.,-2.01187773939257));
#32309=CARTESIAN_POINT('Ctrl Pts',(0.516902681728733,1.,-2.01187773939257));
#32310=CARTESIAN_POINT('Ctrl Pts',(0.512953306961813,-1.,-2.00707309946955));
#32311=CARTESIAN_POINT('Ctrl Pts',(0.512953306961813,1.,-2.00707309946955));
#32312=CARTESIAN_POINT('Ctrl Pts',(0.509046069886152,-1.,-2.00225107134733));
#32313=CARTESIAN_POINT('Ctrl Pts',(0.509046069886152,1.,-2.00225107134733));
#32314=CARTESIAN_POINT('Ctrl Pts',(0.505181361323011,-1.,-1.99741107463567));
#32315=CARTESIAN_POINT('Ctrl Pts',(0.505181361323011,1.,-1.99741107463567));
#32316=CARTESIAN_POINT('Ctrl Pts',(0.501359287727129,-1.,-1.9925514912615));
#32317=CARTESIAN_POINT('Ctrl Pts',(0.501359287727129,1.,-1.9925514912615));
#32318=CARTESIAN_POINT('Ctrl Pts',(0.497579909545564,-1.,-1.98767044752929));
#32319=CARTESIAN_POINT('Ctrl Pts',(0.497579909545564,1.,-1.98767044752929));
#32320=CARTESIAN_POINT('Ctrl Pts',(0.493843476541492,-1.,-1.9827665876182));
#32321=CARTESIAN_POINT('Ctrl Pts',(0.493843476541492,1.,-1.9827665876182));
#32322=CARTESIAN_POINT('Ctrl Pts',(0.490150627860955,-1.,-1.97783973019229));
#32323=CARTESIAN_POINT('Ctrl Pts',(0.490150627860955,1.,-1.97783973019229));
#32324=CARTESIAN_POINT('Ctrl Pts',(0.486502692907661,-1.,-1.97289186263272));
#32325=CARTESIAN_POINT('Ctrl Pts',(0.486502692907661,1.,-1.97289186263272));
#32326=CARTESIAN_POINT('Ctrl Pts',(0.482901662120686,-1.,-1.96792703422358));
#32327=CARTESIAN_POINT('Ctrl Pts',(0.482901662120686,1.,-1.96792703422358));
#32328=CARTESIAN_POINT('Ctrl Pts',(0.479349583074846,-1.,-1.96294933055938));
#32329=CARTESIAN_POINT('Ctrl Pts',(0.479349583074846,1.,-1.96294933055938));
#32330=CARTESIAN_POINT('Ctrl Pts',(0.475848034683171,-1.,-1.95796111148175));
#32331=CARTESIAN_POINT('Ctrl Pts',(0.475848034683171,1.,-1.95796111148175));
#32332=CARTESIAN_POINT('Ctrl Pts',(0.472397672264079,-1.,-1.95296148278136));
#32333=CARTESIAN_POINT('Ctrl Pts',(0.472397672264079,1.,-1.95296148278136));
#32334=CARTESIAN_POINT('Ctrl Pts',(0.468997482913158,-1.,-1.94794381136524));
#32335=CARTESIAN_POINT('Ctrl Pts',(0.468997482913158,1.,-1.94794381136524));
#32336=CARTESIAN_POINT('Ctrl Pts',(0.465645462026064,-1.,-1.94289794196205));
#32337=CARTESIAN_POINT('Ctrl Pts',(0.465645462026064,1.,-1.94289794196205));
#32338=CARTESIAN_POINT('Ctrl Pts',(0.462340031009087,-1.,-1.93781486640834));
#32339=CARTESIAN_POINT('Ctrl Pts',(0.462340031009087,1.,-1.93781486640834));
#32340=CARTESIAN_POINT('Ctrl Pts',(0.459081234547931,-1.,-1.93269066517936));
#32341=CARTESIAN_POINT('Ctrl Pts',(0.459081234547931,1.,-1.93269066517936));
#32342=CARTESIAN_POINT('Ctrl Pts',(0.455872005174335,-1.,-1.92753067150461));
#32343=CARTESIAN_POINT('Ctrl Pts',(0.455872005174335,1.,-1.92753067150461));
#32344=CARTESIAN_POINT('Ctrl Pts',(0.452719478359356,-1.,-1.9223538064847));
#32345=CARTESIAN_POINT('Ctrl Pts',(0.452719478359356,1.,-1.9223538064847));
#32346=CARTESIAN_POINT('Ctrl Pts',(0.449632260106572,-1.,-1.91718342555717));
#32347=CARTESIAN_POINT('Ctrl Pts',(0.449632260106572,1.,-1.91718342555717));
#32348=CARTESIAN_POINT('Ctrl Pts',(0.446617343485651,-1.,-1.91203699981095));
#32349=CARTESIAN_POINT('Ctrl Pts',(0.446617343485651,1.,-1.91203699981095));
#32350=CARTESIAN_POINT('Ctrl Pts',(0.44367755684917,-1.,-1.90691756144906));
#32351=CARTESIAN_POINT('Ctrl Pts',(0.44367755684917,1.,-1.90691756144906));
#32352=CARTESIAN_POINT('Ctrl Pts',(0.44080783370416,-1.,-1.90180124389137));
#32353=CARTESIAN_POINT('Ctrl Pts',(0.44080783370416,1.,-1.90180124389137));
#32354=CARTESIAN_POINT('Ctrl Pts',(0.437995003948443,-1.,-1.89663648956549));
#32355=CARTESIAN_POINT('Ctrl Pts',(0.437995003948443,1.,-1.89663648956549));
#32356=CARTESIAN_POINT('Ctrl Pts',(0.43522566096358,-1.,-1.89136993975585));
#32357=CARTESIAN_POINT('Ctrl Pts',(0.43522566096358,1.,-1.89136993975585));
#32358=CARTESIAN_POINT('Ctrl Pts',(0.432493038548833,-1.,-1.88596913666828));
#32359=CARTESIAN_POINT('Ctrl Pts',(0.432493038548833,1.,-1.88596913666828));
#32360=CARTESIAN_POINT('Ctrl Pts',(0.429803062482217,-1.,-1.88044229001779));
#32361=CARTESIAN_POINT('Ctrl Pts',(0.429803062482217,1.,-1.88044229001779));
#32362=CARTESIAN_POINT('Ctrl Pts',(0.427183828518743,-1.,-1.87486989291334));
#32363=CARTESIAN_POINT('Ctrl Pts',(0.427183828518743,1.,-1.87486989291334));
#32364=CARTESIAN_POINT('Ctrl Pts',(0.424678177290876,-1.,-1.8693780394412));
#32365=CARTESIAN_POINT('Ctrl Pts',(0.424678177290876,1.,-1.8693780394412));
#32366=CARTESIAN_POINT('Ctrl Pts',(0.422327307417884,-1.,-1.86408083333863));
#32367=CARTESIAN_POINT('Ctrl Pts',(0.422327307417884,1.,-1.86408083333863));
#32368=CARTESIAN_POINT('Ctrl Pts',(0.420157287975583,-1.,-1.8590328109667));
#32369=CARTESIAN_POINT('Ctrl Pts',(0.420157287975583,1.,-1.8590328109667));
#32370=CARTESIAN_POINT('Ctrl Pts',(0.418164129144045,-1.,-1.8541763285645));
#32371=CARTESIAN_POINT('Ctrl Pts',(0.418164129144045,1.,-1.8541763285645));
#32372=CARTESIAN_POINT('Ctrl Pts',(0.416300022039885,-1.,-1.84929312930314));
#32373=CARTESIAN_POINT('Ctrl Pts',(0.416300022039885,1.,-1.84929312930314));
#32374=CARTESIAN_POINT('Ctrl Pts',(0.414487438255542,-1.,-1.84405757074218));
#32375=CARTESIAN_POINT('Ctrl Pts',(0.414487438255542,1.,-1.84405757074218));
#32376=CARTESIAN_POINT('Ctrl Pts',(0.412633125322945,-1.,-1.8380895347617));
#32377=CARTESIAN_POINT('Ctrl Pts',(0.412633125322945,1.,-1.8380895347617));
#32378=CARTESIAN_POINT('Ctrl Pts',(0.410641256301276,-1.,-1.83100408895047));
#32379=CARTESIAN_POINT('Ctrl Pts',(0.410641256301276,1.,-1.83100408895047));
#32380=CARTESIAN_POINT('Ctrl Pts',(0.408428948106227,-1.,-1.82247022677562));
#32381=CARTESIAN_POINT('Ctrl Pts',(0.408428948106227,1.,-1.82247022677562));
#32382=CARTESIAN_POINT('Ctrl Pts',(0.405933518407175,-1.,-1.81223801812013));
#32383=CARTESIAN_POINT('Ctrl Pts',(0.405933518407175,1.,-1.81223801812013));
#32384=CARTESIAN_POINT('Ctrl Pts',(0.403107976163396,-1.,-1.80012077173238));
#32385=CARTESIAN_POINT('Ctrl Pts',(0.403107976163396,1.,-1.80012077173238));
#32386=CARTESIAN_POINT('Ctrl Pts',(0.399919403774155,-1.,-1.78598826343754));
#32387=CARTESIAN_POINT('Ctrl Pts',(0.399919403774155,1.,-1.78598826343754));
#32388=CARTESIAN_POINT('Ctrl Pts',(0.396346196110688,-1.,-1.76975560043442));
#32389=CARTESIAN_POINT('Ctrl Pts',(0.396346196110688,1.,-1.76975560043442));
#32390=CARTESIAN_POINT('Ctrl Pts',(0.392375812285395,-1.,-1.75137405310193));
#32391=CARTESIAN_POINT('Ctrl Pts',(0.392375812285395,1.,-1.75137405310193));
#32392=CARTESIAN_POINT('Ctrl Pts',(0.388877023502615,-1.,-1.73493170972829));
#32393=CARTESIAN_POINT('Ctrl Pts',(0.388877023502615,1.,-1.73493170972829));
#32394=CARTESIAN_POINT('Ctrl Pts',(0.386070790323281,-1.,-1.72162022244582));
#32395=CARTESIAN_POINT('Ctrl Pts',(0.386070790323281,1.,-1.72162022244582));
#32396=CARTESIAN_POINT('Ctrl Pts',(0.384119047314215,-1.,-1.71231062891398));
#32397=CARTESIAN_POINT('Ctrl Pts',(0.384119047314215,1.,-1.71231062891398));
#32398=CARTESIAN_POINT('Ctrl Pts',(0.383122945602004,-1.,-1.7075470150345));
#32399=CARTESIAN_POINT('Ctrl Pts',(0.383122945602004,1.,-1.7075470150345));
#32400=CARTESIAN_POINT('',(0.61342227326009,1.,-2.11275013067528));
#32401=CARTESIAN_POINT('Ctrl Pts',(0.61342227326009,1.,-2.11275013067528));
#32402=CARTESIAN_POINT('Ctrl Pts',(0.61246736556225,1.,-2.11187554260142));
#32403=CARTESIAN_POINT('Ctrl Pts',(0.610560911691113,1.,-2.11012443807661));
#32404=CARTESIAN_POINT('Ctrl Pts',(0.607711315456826,1.,-2.10749199615859));
#32405=CARTESIAN_POINT('Ctrl Pts',(0.603932030738212,1.,-2.10397049887709));
#32406=CARTESIAN_POINT('Ctrl Pts',(0.599241616422144,1.,-2.09954930865331));
#32407=CARTESIAN_POINT('Ctrl Pts',(0.594585006052823,1.,-2.09510876220501));
#32408=CARTESIAN_POINT('Ctrl Pts',(0.589962365403189,1.,-2.09064881812053));
#32409=CARTESIAN_POINT('Ctrl Pts',(0.585373918990895,1.,-2.086169437277));
#32410=CARTESIAN_POINT('Ctrl Pts',(0.580819952107256,1.,-2.08167059018138));
#32411=CARTESIAN_POINT('Ctrl Pts',(0.576300797416274,1.,-2.07715226767361));
#32412=CARTESIAN_POINT('Ctrl Pts',(0.571816823242411,1.,-2.07261449292758));
#32413=CARTESIAN_POINT('Ctrl Pts',(0.567368421181229,1.,-2.06805732997383));
#32414=CARTESIAN_POINT('Ctrl Pts',(0.562955993082574,1.,-2.06348090160697));
#32415=CARTESIAN_POINT('Ctrl Pts',(0.558579940185467,1.,-2.05888537756571));
#32416=CARTESIAN_POINT('Ctrl Pts',(0.554240657464109,1.,-2.05427091604482));
#32417=CARTESIAN_POINT('Ctrl Pts',(0.549938525150342,1.,-2.04963761077974));
#32418=CARTESIAN_POINT('Ctrl Pts',(0.545673903817348,1.,-2.0449854471456));
#32419=CARTESIAN_POINT('Ctrl Pts',(0.54144712061552,1.,-2.0403142269048));
#32420=CARTESIAN_POINT('Ctrl Pts',(0.537258489833134,1.,-2.03562362953993));
#32421=CARTESIAN_POINT('Ctrl Pts',(0.533108355132905,1.,-2.03091336214401));
#32422=CARTESIAN_POINT('Ctrl Pts',(0.52899712724191,1.,-2.02618329083289));
#32423=CARTESIAN_POINT('Ctrl Pts',(0.524925318333518,1.,-2.02143356304712));
#32424=CARTESIAN_POINT('Ctrl Pts',(0.520893590399428,1.,-2.01666477917306));
#32425=CARTESIAN_POINT('Ctrl Pts',(0.516902681728733,1.,-2.01187773939257));
#32426=CARTESIAN_POINT('Ctrl Pts',(0.512953306961813,1.,-2.00707309946955));
#32427=CARTESIAN_POINT('Ctrl Pts',(0.509046069886152,1.,-2.00225107134733));
#32428=CARTESIAN_POINT('Ctrl Pts',(0.505181361323011,1.,-1.99741107463567));
#32429=CARTESIAN_POINT('Ctrl Pts',(0.501359287727129,1.,-1.9925514912615));
#32430=CARTESIAN_POINT('Ctrl Pts',(0.497579909545564,1.,-1.98767044752929));
#32431=CARTESIAN_POINT('Ctrl Pts',(0.493843476541492,1.,-1.9827665876182));
#32432=CARTESIAN_POINT('Ctrl Pts',(0.490150627860955,1.,-1.97783973019229));
#32433=CARTESIAN_POINT('Ctrl Pts',(0.486502692907661,1.,-1.97289186263272));
#32434=CARTESIAN_POINT('Ctrl Pts',(0.482901662120686,1.,-1.96792703422358));
#32435=CARTESIAN_POINT('Ctrl Pts',(0.479349583074846,1.,-1.96294933055938));
#32436=CARTESIAN_POINT('Ctrl Pts',(0.475848034683171,1.,-1.95796111148175));
#32437=CARTESIAN_POINT('Ctrl Pts',(0.472397672264079,1.,-1.95296148278136));
#32438=CARTESIAN_POINT('Ctrl Pts',(0.468997482913158,1.,-1.94794381136524));
#32439=CARTESIAN_POINT('Ctrl Pts',(0.465645462026064,1.,-1.94289794196205));
#32440=CARTESIAN_POINT('Ctrl Pts',(0.462340031009087,1.,-1.93781486640834));
#32441=CARTESIAN_POINT('Ctrl Pts',(0.459081234547931,1.,-1.93269066517936));
#32442=CARTESIAN_POINT('Ctrl Pts',(0.455872005174335,1.,-1.92753067150461));
#32443=CARTESIAN_POINT('Ctrl Pts',(0.452719478359356,1.,-1.9223538064847));
#32444=CARTESIAN_POINT('Ctrl Pts',(0.449632260106572,1.,-1.91718342555717));
#32445=CARTESIAN_POINT('Ctrl Pts',(0.446617343485651,1.,-1.91203699981095));
#32446=CARTESIAN_POINT('Ctrl Pts',(0.44367755684917,1.,-1.90691756144906));
#32447=CARTESIAN_POINT('Ctrl Pts',(0.44080783370416,1.,-1.90180124389137));
#32448=CARTESIAN_POINT('Ctrl Pts',(0.437995003948443,1.,-1.89663648956549));
#32449=CARTESIAN_POINT('Ctrl Pts',(0.43522566096358,1.,-1.89136993975585));
#32450=CARTESIAN_POINT('Ctrl Pts',(0.432493038548833,1.,-1.88596913666828));
#32451=CARTESIAN_POINT('Ctrl Pts',(0.429803062482217,1.,-1.88044229001779));
#32452=CARTESIAN_POINT('Ctrl Pts',(0.427183828518743,1.,-1.87486989291334));
#32453=CARTESIAN_POINT('Ctrl Pts',(0.424678177290876,1.,-1.8693780394412));
#32454=CARTESIAN_POINT('Ctrl Pts',(0.422327307417884,1.,-1.86408083333863));
#32455=CARTESIAN_POINT('Ctrl Pts',(0.420157287975583,1.,-1.8590328109667));
#32456=CARTESIAN_POINT('Ctrl Pts',(0.418164129144045,1.,-1.8541763285645));
#32457=CARTESIAN_POINT('Ctrl Pts',(0.416300022039885,1.,-1.84929312930314));
#32458=CARTESIAN_POINT('Ctrl Pts',(0.414487438255542,1.,-1.84405757074218));
#32459=CARTESIAN_POINT('Ctrl Pts',(0.412633125322945,1.,-1.8380895347617));
#32460=CARTESIAN_POINT('Ctrl Pts',(0.410641256301276,1.,-1.83100408895047));
#32461=CARTESIAN_POINT('Ctrl Pts',(0.408428948106227,1.,-1.82247022677562));
#32462=CARTESIAN_POINT('Ctrl Pts',(0.405933518407175,1.,-1.81223801812013));
#32463=CARTESIAN_POINT('Ctrl Pts',(0.403107976163396,1.,-1.80012077173238));
#32464=CARTESIAN_POINT('Ctrl Pts',(0.399919403774155,1.,-1.78598826343754));
#32465=CARTESIAN_POINT('Ctrl Pts',(0.396346196110688,1.,-1.76975560043442));
#32466=CARTESIAN_POINT('Ctrl Pts',(0.392375812285395,1.,-1.75137405310193));
#32467=CARTESIAN_POINT('Ctrl Pts',(0.388877023502615,1.,-1.73493170972829));
#32468=CARTESIAN_POINT('Ctrl Pts',(0.386070790323281,1.,-1.72162022244582));
#32469=CARTESIAN_POINT('Ctrl Pts',(0.384119047314215,1.,-1.71231062891398));
#32470=CARTESIAN_POINT('Ctrl Pts',(0.383122945602004,1.,-1.7075470150345));
#32471=CARTESIAN_POINT('',(0.61342227326009,0.,-2.11275013067528));
#32472=CARTESIAN_POINT('Origin',(0.745574324794401,0.,-2.0698113262342));
#32473=CARTESIAN_POINT('',(0.745574324794401,1.,-2.0698113262342));
#32474=CARTESIAN_POINT('',(0.61342227326009,1.,-2.11275013067528));
#32475=CARTESIAN_POINT('',(0.745574324794401,0.,-2.0698113262342));
#32476=CARTESIAN_POINT('Ctrl Pts',(0.693717979106306,-1.,-1.60662857109684));
#32477=CARTESIAN_POINT('Ctrl Pts',(0.693717979106306,1.,-1.60662857109684));
#32478=CARTESIAN_POINT('Ctrl Pts',(0.695712097881194,-1.,-1.61106790958151));
#32479=CARTESIAN_POINT('Ctrl Pts',(0.695712097881194,1.,-1.61106790958151));
#32480=CARTESIAN_POINT('Ctrl Pts',(0.699605146405088,-1.,-1.61974673472612));
#32481=CARTESIAN_POINT('Ctrl Pts',(0.699605146405088,1.,-1.61974673472612));
#32482=CARTESIAN_POINT('Ctrl Pts',(0.705159151988319,-1.,-1.63216541664676));
#32483=CARTESIAN_POINT('Ctrl Pts',(0.705159151988319,1.,-1.63216541664676));
#32484=CARTESIAN_POINT('Ctrl Pts',(0.711993139355394,-1.,-1.64752408832016));
#32485=CARTESIAN_POINT('Ctrl Pts',(0.711993139355394,1.,-1.64752408832016));
#32486=CARTESIAN_POINT('Ctrl Pts',(0.719585433804282,-1.,-1.6647288055568));
#32487=CARTESIAN_POINT('Ctrl Pts',(0.719585433804282,1.,-1.6647288055568));
#32488=CARTESIAN_POINT('Ctrl Pts',(0.726235967997433,-1.,-1.67996158455503));
#32489=CARTESIAN_POINT('Ctrl Pts',(0.726235967997433,1.,-1.67996158455503));
#32490=CARTESIAN_POINT('Ctrl Pts',(0.731963238697195,-1.,-1.69326921975743));
#32491=CARTESIAN_POINT('Ctrl Pts',(0.731963238697195,1.,-1.69326921975743));
#32492=CARTESIAN_POINT('Ctrl Pts',(0.736799665724771,-1.,-1.70473309006121));
#32493=CARTESIAN_POINT('Ctrl Pts',(0.736799665724771,1.,-1.70473309006121));
#32494=CARTESIAN_POINT('Ctrl Pts',(0.740795162032087,-1.,-1.71447789751927));
#32495=CARTESIAN_POINT('Ctrl Pts',(0.740795162032087,1.,-1.71447789751927));
#32496=CARTESIAN_POINT('Ctrl Pts',(0.744021445433764,-1.,-1.7226822991693));
#32497=CARTESIAN_POINT('Ctrl Pts',(0.744021445433764,1.,-1.7226822991693));
#32498=CARTESIAN_POINT('Ctrl Pts',(0.746574710096436,-1.,-1.72958533647399));
#32499=CARTESIAN_POINT('Ctrl Pts',(0.746574710096436,1.,-1.72958533647399));
#32500=CARTESIAN_POINT('Ctrl Pts',(0.748582462954854,-1.,-1.73550351679848));
#32501=CARTESIAN_POINT('Ctrl Pts',(0.748582462954854,1.,-1.73550351679848));
#32502=CARTESIAN_POINT('Ctrl Pts',(0.75019343597954,-1.,-1.74080458266705));
#32503=CARTESIAN_POINT('Ctrl Pts',(0.75019343597954,1.,-1.74080458266705));
#32504=CARTESIAN_POINT('Ctrl Pts',(0.751555614163629,-1.,-1.74585086852298));
#32505=CARTESIAN_POINT('Ctrl Pts',(0.751555614163629,1.,-1.74585086852298));
#32506=CARTESIAN_POINT('Ctrl Pts',(0.752797683531377,-1.,-1.75095139468809));
#32507=CARTESIAN_POINT('Ctrl Pts',(0.752797683531377,1.,-1.75095139468809));
#32508=CARTESIAN_POINT('Ctrl Pts',(0.75400925402848,-1.,-1.75631083600175));
#32509=CARTESIAN_POINT('Ctrl Pts',(0.75400925402848,1.,-1.75631083600175));
#32510=CARTESIAN_POINT('Ctrl Pts',(0.755220979975262,-1.,-1.7619781724032));
#32511=CARTESIAN_POINT('Ctrl Pts',(0.755220979975262,1.,-1.7619781724032));
#32512=CARTESIAN_POINT('Ctrl Pts',(0.756421896028403,-1.,-1.76789396003141));
#32513=CARTESIAN_POINT('Ctrl Pts',(0.756421896028403,1.,-1.76789396003141));
#32514=CARTESIAN_POINT('Ctrl Pts',(0.757578264077238,-1.,-1.77394167108342));
#32515=CARTESIAN_POINT('Ctrl Pts',(0.757578264077238,1.,-1.77394167108342));
#32516=CARTESIAN_POINT('Ctrl Pts',(0.75865062667738,-1.,-1.77999411220912));
#32517=CARTESIAN_POINT('Ctrl Pts',(0.75865062667738,1.,-1.77999411220912));
#32518=CARTESIAN_POINT('Ctrl Pts',(0.759614401109868,-1.,-1.78596964884527));
#32519=CARTESIAN_POINT('Ctrl Pts',(0.759614401109868,1.,-1.78596964884527));
#32520=CARTESIAN_POINT('Ctrl Pts',(0.760469555880425,-1.,-1.79185815610802));
#32521=CARTESIAN_POINT('Ctrl Pts',(0.760469555880425,1.,-1.79185815610802));
#32522=CARTESIAN_POINT('Ctrl Pts',(0.761229695230359,-1.,-1.79768986997735));
#32523=CARTESIAN_POINT('Ctrl Pts',(0.761229695230359,1.,-1.79768986997735));
#32524=CARTESIAN_POINT('Ctrl Pts',(0.761915336443515,-1.,-1.80351583877334));
#32525=CARTESIAN_POINT('Ctrl Pts',(0.761915336443515,1.,-1.80351583877334));
#32526=CARTESIAN_POINT('Ctrl Pts',(0.762546129464036,-1.,-1.80938551463989));
#32527=CARTESIAN_POINT('Ctrl Pts',(0.762546129464036,1.,-1.80938551463989));
#32528=CARTESIAN_POINT('Ctrl Pts',(0.763132003836783,-1.,-1.81532118405566));
#32529=CARTESIAN_POINT('Ctrl Pts',(0.763132003836783,1.,-1.81532118405566));
#32530=CARTESIAN_POINT('Ctrl Pts',(0.763673465462854,-1.,-1.82131873145297));
#32531=CARTESIAN_POINT('Ctrl Pts',(0.763673465462854,1.,-1.82131873145297));
#32532=CARTESIAN_POINT('Ctrl Pts',(0.764165902606055,-1.,-1.8273599120008));
#32533=CARTESIAN_POINT('Ctrl Pts',(0.764165902606055,1.,-1.8273599120008));
#32534=CARTESIAN_POINT('Ctrl Pts',(0.764602549687845,-1.,-1.8334207722714));
#32535=CARTESIAN_POINT('Ctrl Pts',(0.764602549687845,1.,-1.8334207722714));
#32536=CARTESIAN_POINT('Ctrl Pts',(0.764978057881687,-1.,-1.83948181064823));
#32537=CARTESIAN_POINT('Ctrl Pts',(0.764978057881687,1.,-1.83948181064823));
#32538=CARTESIAN_POINT('Ctrl Pts',(0.765291664861971,-1.,-1.84553698875911));
#32539=CARTESIAN_POINT('Ctrl Pts',(0.765291664861971,1.,-1.84553698875911));
#32540=CARTESIAN_POINT('Ctrl Pts',(0.765545710619023,-1.,-1.85158945130054));
#32541=CARTESIAN_POINT('Ctrl Pts',(0.765545710619023,1.,-1.85158945130054));
#32542=CARTESIAN_POINT('Ctrl Pts',(0.765744212909305,-1.,-1.85764741390391));
#32543=CARTESIAN_POINT('Ctrl Pts',(0.765744212909305,1.,-1.85764741390391));
#32544=CARTESIAN_POINT('Ctrl Pts',(0.765891519092557,-1.,-1.86372027063315));
#32545=CARTESIAN_POINT('Ctrl Pts',(0.765891519092557,1.,-1.86372027063315));
#32546=CARTESIAN_POINT('Ctrl Pts',(0.765990708546111,-1.,-1.86981398314345));
#32547=CARTESIAN_POINT('Ctrl Pts',(0.765990708546111,1.,-1.86981398314345));
#32548=CARTESIAN_POINT('Ctrl Pts',(0.766042837036759,-1.,-1.87592888967886));
#32549=CARTESIAN_POINT('Ctrl Pts',(0.766042837036759,1.,-1.87592888967886));
#32550=CARTESIAN_POINT('Ctrl Pts',(0.766047794851868,-1.,-1.88206215302561));
#32551=CARTESIAN_POINT('Ctrl Pts',(0.766047794851868,1.,-1.88206215302561));
#32552=CARTESIAN_POINT('Ctrl Pts',(0.76600483706209,-1.,-1.88820926433409));
#32553=CARTESIAN_POINT('Ctrl Pts',(0.76600483706209,1.,-1.88820926433409));
#32554=CARTESIAN_POINT('Ctrl Pts',(0.765913193856979,-1.,-1.89436577771389));
#32555=CARTESIAN_POINT('Ctrl Pts',(0.765913193856979,1.,-1.89436577771389));
#32556=CARTESIAN_POINT('Ctrl Pts',(0.765772772593395,-1.,-1.90052930393599));
#32557=CARTESIAN_POINT('Ctrl Pts',(0.765772772593395,1.,-1.90052930393599));
#32558=CARTESIAN_POINT('Ctrl Pts',(0.765584196937936,-1.,-1.90669961402362));
#32559=CARTESIAN_POINT('Ctrl Pts',(0.765584196937936,1.,-1.90669961402362));
#32560=CARTESIAN_POINT('Ctrl Pts',(0.765348465884739,-1.,-1.91287765805174));
#32561=CARTESIAN_POINT('Ctrl Pts',(0.765348465884739,1.,-1.91287765805174));
#32562=CARTESIAN_POINT('Ctrl Pts',(0.765066729667095,-1.,-1.91906491634197));
#32563=CARTESIAN_POINT('Ctrl Pts',(0.765066729667095,1.,-1.91906491634197));
#32564=CARTESIAN_POINT('Ctrl Pts',(0.764740025488189,-1.,-1.92526263537041));
#32565=CARTESIAN_POINT('Ctrl Pts',(0.764740025488189,1.,-1.92526263537041));
#32566=CARTESIAN_POINT('Ctrl Pts',(0.764369010673889,-1.,-1.93147105496367));
#32567=CARTESIAN_POINT('Ctrl Pts',(0.764369010673889,1.,-1.93147105496367));
#32568=CARTESIAN_POINT('Ctrl Pts',(0.763954049121393,-1.,-1.93768964875867));
#32569=CARTESIAN_POINT('Ctrl Pts',(0.763954049121393,1.,-1.93768964875867));
#32570=CARTESIAN_POINT('Ctrl Pts',(0.76349533353858,-1.,-1.94391746617626));
#32571=CARTESIAN_POINT('Ctrl Pts',(0.76349533353858,1.,-1.94391746617626));
#32572=CARTESIAN_POINT('Ctrl Pts',(0.762992990878774,-1.,-1.95015342590025));
#32573=CARTESIAN_POINT('Ctrl Pts',(0.762992990878774,1.,-1.95015342590025));
#32574=CARTESIAN_POINT('Ctrl Pts',(0.762447203806263,-1.,-1.95639665309893));
#32575=CARTESIAN_POINT('Ctrl Pts',(0.762447203806263,1.,-1.95639665309893));
#32576=CARTESIAN_POINT('Ctrl Pts',(0.761858300014575,-1.,-1.96264672744229));
#32577=CARTESIAN_POINT('Ctrl Pts',(0.761858300014575,1.,-1.96264672744229));
#32578=CARTESIAN_POINT('Ctrl Pts',(0.761226690483986,-1.,-1.96890351582545));
#32579=CARTESIAN_POINT('Ctrl Pts',(0.761226690483986,1.,-1.96890351582545));
#32580=CARTESIAN_POINT('Ctrl Pts',(0.760552825409855,-1.,-1.97516705321521));
#32581=CARTESIAN_POINT('Ctrl Pts',(0.760552825409855,1.,-1.97516705321521));
#32582=CARTESIAN_POINT('Ctrl Pts',(0.759837147452135,-1.,-1.98143741418156));
#32583=CARTESIAN_POINT('Ctrl Pts',(0.759837147452135,1.,-1.98143741418156));
#32584=CARTESIAN_POINT('Ctrl Pts',(0.759080037802242,-1.,-1.98771456680806));
#32585=CARTESIAN_POINT('Ctrl Pts',(0.759080037802242,1.,-1.98771456680806));
#32586=CARTESIAN_POINT('Ctrl Pts',(0.758281796766377,-1.,-1.9939983109871));
#32587=CARTESIAN_POINT('Ctrl Pts',(0.758281796766377,1.,-1.9939983109871));
#32588=CARTESIAN_POINT('Ctrl Pts',(0.757442676862341,-1.,-2.00028834739072));
#32589=CARTESIAN_POINT('Ctrl Pts',(0.757442676862341,1.,-2.00028834739072));
#32590=CARTESIAN_POINT('Ctrl Pts',(0.756562904646496,-1.,-2.00658431587682));
#32591=CARTESIAN_POINT('Ctrl Pts',(0.756562904646496,1.,-2.00658431587682));
#32592=CARTESIAN_POINT('Ctrl Pts',(0.7556427049581,-1.,-2.01288584328149));
#32593=CARTESIAN_POINT('Ctrl Pts',(0.7556427049581,1.,-2.01288584328149));
#32594=CARTESIAN_POINT('Ctrl Pts',(0.75468233072352,-1.,-2.01919259406003));
#32595=CARTESIAN_POINT('Ctrl Pts',(0.75468233072352,1.,-2.01919259406003));
#32596=CARTESIAN_POINT('Ctrl Pts',(0.753682061113765,-1.,-2.02550428623587));
#32597=CARTESIAN_POINT('Ctrl Pts',(0.753682061113765,1.,-2.02550428623587));
#32598=CARTESIAN_POINT('Ctrl Pts',(0.752642180488104,-1.,-2.03182068456467));
#32599=CARTESIAN_POINT('Ctrl Pts',(0.752642180488104,1.,-2.03182068456467));
#32600=CARTESIAN_POINT('Ctrl Pts',(0.751562963361383,-1.,-2.03814160092173));
#32601=CARTESIAN_POINT('Ctrl Pts',(0.751562963361383,1.,-2.03814160092173));
#32602=CARTESIAN_POINT('Ctrl Pts',(0.750444657874758,-1.,-2.04446689147754));
#32603=CARTESIAN_POINT('Ctrl Pts',(0.750444657874758,1.,-2.04446689147754));
#32604=CARTESIAN_POINT('Ctrl Pts',(0.749287468663053,-1.,-2.05079645591606));
#32605=CARTESIAN_POINT('Ctrl Pts',(0.749287468663053,1.,-2.05079645591606));
#32606=CARTESIAN_POINT('Ctrl Pts',(0.748091554181101,-1.,-2.05713023030263));
#32607=CARTESIAN_POINT('Ctrl Pts',(0.748091554181101,1.,-2.05713023030263));
#32608=CARTESIAN_POINT('Ctrl Pts',(0.747103932785504,-1.,-2.06220058927162));
#32609=CARTESIAN_POINT('Ctrl Pts',(0.747103932785504,1.,-2.06220058927162));
#32610=CARTESIAN_POINT('Ctrl Pts',(0.746345871542695,-1.,-2.06600523016401));
#32611=CARTESIAN_POINT('Ctrl Pts',(0.746345871542695,1.,-2.06600523016401));
#32612=CARTESIAN_POINT('Ctrl Pts',(0.74583279137781,-1.,-2.06854248895575));
#32613=CARTESIAN_POINT('Ctrl Pts',(0.74583279137781,1.,-2.06854248895575));
#32614=CARTESIAN_POINT('Ctrl Pts',(0.745574324794401,-1.,-2.0698113262342));
#32615=CARTESIAN_POINT('Ctrl Pts',(0.745574324794401,1.,-2.0698113262342));
#32616=CARTESIAN_POINT('',(0.693717979106306,1.,-1.60662857109684));
#32617=CARTESIAN_POINT('Ctrl Pts',(0.693717979106306,1.,-1.60662857109684));
#32618=CARTESIAN_POINT('Ctrl Pts',(0.695712097881194,1.,-1.61106790958151));
#32619=CARTESIAN_POINT('Ctrl Pts',(0.699605146405088,1.,-1.61974673472612));
#32620=CARTESIAN_POINT('Ctrl Pts',(0.705159151988319,1.,-1.63216541664676));
#32621=CARTESIAN_POINT('Ctrl Pts',(0.711993139355394,1.,-1.64752408832016));
#32622=CARTESIAN_POINT('Ctrl Pts',(0.719585433804282,1.,-1.6647288055568));
#32623=CARTESIAN_POINT('Ctrl Pts',(0.726235967997433,1.,-1.67996158455503));
#32624=CARTESIAN_POINT('Ctrl Pts',(0.731963238697195,1.,-1.69326921975743));
#32625=CARTESIAN_POINT('Ctrl Pts',(0.736799665724771,1.,-1.70473309006121));
#32626=CARTESIAN_POINT('Ctrl Pts',(0.740795162032087,1.,-1.71447789751927));
#32627=CARTESIAN_POINT('Ctrl Pts',(0.744021445433764,1.,-1.7226822991693));
#32628=CARTESIAN_POINT('Ctrl Pts',(0.746574710096436,1.,-1.72958533647399));
#32629=CARTESIAN_POINT('Ctrl Pts',(0.748582462954854,1.,-1.73550351679848));
#32630=CARTESIAN_POINT('Ctrl Pts',(0.75019343597954,1.,-1.74080458266705));
#32631=CARTESIAN_POINT('Ctrl Pts',(0.751555614163629,1.,-1.74585086852298));
#32632=CARTESIAN_POINT('Ctrl Pts',(0.752797683531377,1.,-1.75095139468809));
#32633=CARTESIAN_POINT('Ctrl Pts',(0.75400925402848,1.,-1.75631083600175));
#32634=CARTESIAN_POINT('Ctrl Pts',(0.755220979975262,1.,-1.7619781724032));
#32635=CARTESIAN_POINT('Ctrl Pts',(0.756421896028403,1.,-1.76789396003141));
#32636=CARTESIAN_POINT('Ctrl Pts',(0.757578264077238,1.,-1.77394167108342));
#32637=CARTESIAN_POINT('Ctrl Pts',(0.75865062667738,1.,-1.77999411220912));
#32638=CARTESIAN_POINT('Ctrl Pts',(0.759614401109868,1.,-1.78596964884527));
#32639=CARTESIAN_POINT('Ctrl Pts',(0.760469555880425,1.,-1.79185815610802));
#32640=CARTESIAN_POINT('Ctrl Pts',(0.761229695230359,1.,-1.79768986997735));
#32641=CARTESIAN_POINT('Ctrl Pts',(0.761915336443515,1.,-1.80351583877334));
#32642=CARTESIAN_POINT('Ctrl Pts',(0.762546129464036,1.,-1.80938551463989));
#32643=CARTESIAN_POINT('Ctrl Pts',(0.763132003836783,1.,-1.81532118405566));
#32644=CARTESIAN_POINT('Ctrl Pts',(0.763673465462854,1.,-1.82131873145297));
#32645=CARTESIAN_POINT('Ctrl Pts',(0.764165902606055,1.,-1.8273599120008));
#32646=CARTESIAN_POINT('Ctrl Pts',(0.764602549687845,1.,-1.8334207722714));
#32647=CARTESIAN_POINT('Ctrl Pts',(0.764978057881687,1.,-1.83948181064823));
#32648=CARTESIAN_POINT('Ctrl Pts',(0.765291664861971,1.,-1.84553698875911));
#32649=CARTESIAN_POINT('Ctrl Pts',(0.765545710619023,1.,-1.85158945130054));
#32650=CARTESIAN_POINT('Ctrl Pts',(0.765744212909305,1.,-1.85764741390391));
#32651=CARTESIAN_POINT('Ctrl Pts',(0.765891519092557,1.,-1.86372027063315));
#32652=CARTESIAN_POINT('Ctrl Pts',(0.765990708546111,1.,-1.86981398314345));
#32653=CARTESIAN_POINT('Ctrl Pts',(0.766042837036759,1.,-1.87592888967886));
#32654=CARTESIAN_POINT('Ctrl Pts',(0.766047794851868,1.,-1.88206215302561));
#32655=CARTESIAN_POINT('Ctrl Pts',(0.76600483706209,1.,-1.88820926433409));
#32656=CARTESIAN_POINT('Ctrl Pts',(0.765913193856979,1.,-1.89436577771389));
#32657=CARTESIAN_POINT('Ctrl Pts',(0.765772772593395,1.,-1.90052930393599));
#32658=CARTESIAN_POINT('Ctrl Pts',(0.765584196937936,1.,-1.90669961402362));
#32659=CARTESIAN_POINT('Ctrl Pts',(0.765348465884739,1.,-1.91287765805174));
#32660=CARTESIAN_POINT('Ctrl Pts',(0.765066729667095,1.,-1.91906491634197));
#32661=CARTESIAN_POINT('Ctrl Pts',(0.764740025488189,1.,-1.92526263537041));
#32662=CARTESIAN_POINT('Ctrl Pts',(0.764369010673889,1.,-1.93147105496367));
#32663=CARTESIAN_POINT('Ctrl Pts',(0.763954049121393,1.,-1.93768964875867));
#32664=CARTESIAN_POINT('Ctrl Pts',(0.76349533353858,1.,-1.94391746617626));
#32665=CARTESIAN_POINT('Ctrl Pts',(0.762992990878774,1.,-1.95015342590025));
#32666=CARTESIAN_POINT('Ctrl Pts',(0.762447203806263,1.,-1.95639665309893));
#32667=CARTESIAN_POINT('Ctrl Pts',(0.761858300014575,1.,-1.96264672744229));
#32668=CARTESIAN_POINT('Ctrl Pts',(0.761226690483986,1.,-1.96890351582545));
#32669=CARTESIAN_POINT('Ctrl Pts',(0.760552825409855,1.,-1.97516705321521));
#32670=CARTESIAN_POINT('Ctrl Pts',(0.759837147452135,1.,-1.98143741418156));
#32671=CARTESIAN_POINT('Ctrl Pts',(0.759080037802242,1.,-1.98771456680806));
#32672=CARTESIAN_POINT('Ctrl Pts',(0.758281796766377,1.,-1.9939983109871));
#32673=CARTESIAN_POINT('Ctrl Pts',(0.757442676862341,1.,-2.00028834739072));
#32674=CARTESIAN_POINT('Ctrl Pts',(0.756562904646496,1.,-2.00658431587682));
#32675=CARTESIAN_POINT('Ctrl Pts',(0.7556427049581,1.,-2.01288584328149));
#32676=CARTESIAN_POINT('Ctrl Pts',(0.75468233072352,1.,-2.01919259406003));
#32677=CARTESIAN_POINT('Ctrl Pts',(0.753682061113765,1.,-2.02550428623587));
#32678=CARTESIAN_POINT('Ctrl Pts',(0.752642180488104,1.,-2.03182068456467));
#32679=CARTESIAN_POINT('Ctrl Pts',(0.751562963361383,1.,-2.03814160092173));
#32680=CARTESIAN_POINT('Ctrl Pts',(0.750444657874758,1.,-2.04446689147754));
#32681=CARTESIAN_POINT('Ctrl Pts',(0.749287468663053,1.,-2.05079645591606));
#32682=CARTESIAN_POINT('Ctrl Pts',(0.748091554181101,1.,-2.05713023030263));
#32683=CARTESIAN_POINT('Ctrl Pts',(0.747103932785504,1.,-2.06220058927162));
#32684=CARTESIAN_POINT('Ctrl Pts',(0.746345871542695,1.,-2.06600523016401));
#32685=CARTESIAN_POINT('Ctrl Pts',(0.74583279137781,1.,-2.06854248895575));
#32686=CARTESIAN_POINT('Ctrl Pts',(0.745574324794401,1.,-2.0698113262342));
#32687=CARTESIAN_POINT('',(0.693717979106306,0.,-1.60662857109684));
#32688=CARTESIAN_POINT('Origin',(0.,0.,0.));
#32689=CARTESIAN_POINT('',(0.892032620296855,1.,-1.5055822144029));
#32690=CARTESIAN_POINT('Origin',(0.,1.,0.));
#32691=CARTESIAN_POINT('',(0.892032620296855,0.,-1.5055822144029));
#32692=CARTESIAN_POINT('Ctrl Pts',(1.23627494547115,-1.,-1.81978687191668));
#32693=CARTESIAN_POINT('Ctrl Pts',(1.23627494547115,1.,-1.81978687191668));
#32694=CARTESIAN_POINT('Ctrl Pts',(1.23509651170476,-1.,-1.81925017193666));
#32695=CARTESIAN_POINT('Ctrl Pts',(1.23509651170476,1.,-1.81925017193666));
#32696=CARTESIAN_POINT('Ctrl Pts',(1.2327422452705,-1.,-1.81817389921279));
#32697=CARTESIAN_POINT('Ctrl Pts',(1.2327422452705,1.,-1.81817389921279));
#32698=CARTESIAN_POINT('Ctrl Pts',(1.2292186489137,-1.,-1.8165508718364));
#32699=CARTESIAN_POINT('Ctrl Pts',(1.2292186489137,1.,-1.8165508718364));
#32700=CARTESIAN_POINT('Ctrl Pts',(1.2245361330495,-1.,-1.81436959210434));
#32701=CARTESIAN_POINT('Ctrl Pts',(1.2245361330495,1.,-1.81436959210434));
#32702=CARTESIAN_POINT('Ctrl Pts',(1.21870906103557,-1.,-1.81161420806656));
#32703=CARTESIAN_POINT('Ctrl Pts',(1.21870906103557,1.,-1.81161420806656));
#32704=CARTESIAN_POINT('Ctrl Pts',(1.21290815708314,-1.,-1.80882996917129));
#32705=CARTESIAN_POINT('Ctrl Pts',(1.21290815708314,1.,-1.80882996917129));
#32706=CARTESIAN_POINT('Ctrl Pts',(1.20713356605475,-1.,-1.80601678480707));
#32707=CARTESIAN_POINT('Ctrl Pts',(1.20713356605475,1.,-1.80601678480707));
#32708=CARTESIAN_POINT('Ctrl Pts',(1.20138548938974,-1.,-1.80317454838603));
#32709=CARTESIAN_POINT('Ctrl Pts',(1.20138548938974,1.,-1.80317454838603));
#32710=CARTESIAN_POINT('Ctrl Pts',(1.19566418930242,-1.,-1.80030314369879));
#32711=CARTESIAN_POINT('Ctrl Pts',(1.19566418930242,1.,-1.80030314369879));
#32712=CARTESIAN_POINT('Ctrl Pts',(1.18996997934445,-1.,-1.79740245923478));
#32713=CARTESIAN_POINT('Ctrl Pts',(1.18996997934445,1.,-1.79740245923478));
#32714=CARTESIAN_POINT('Ctrl Pts',(1.18430321697432,-1.,-1.79447240321515));
#32715=CARTESIAN_POINT('Ctrl Pts',(1.18430321697432,1.,-1.79447240321515));
#32716=CARTESIAN_POINT('Ctrl Pts',(1.17866429440809,-1.,-1.79151291552689));
#32717=CARTESIAN_POINT('Ctrl Pts',(1.17866429440809,1.,-1.79151291552689));
#32718=CARTESIAN_POINT('Ctrl Pts',(1.17305363177328,-1.,-1.78852398877617));
#32719=CARTESIAN_POINT('Ctrl Pts',(1.17305363177328,1.,-1.78852398877617));
#32720=CARTESIAN_POINT('Ctrl Pts',(1.16747166312303,-1.,-1.78550566040443));
#32721=CARTESIAN_POINT('Ctrl Pts',(1.16747166312303,1.,-1.78550566040443));
#32722=CARTESIAN_POINT('Ctrl Pts',(1.16191881298499,-1.,-1.78245795881009));
#32723=CARTESIAN_POINT('Ctrl Pts',(1.16191881298499,1.,-1.78245795881009));
#32724=CARTESIAN_POINT('Ctrl Pts',(1.15639547194698,-1.,-1.77938085564275));
#32725=CARTESIAN_POINT('Ctrl Pts',(1.15639547194698,1.,-1.77938085564275));
#32726=CARTESIAN_POINT('Ctrl Pts',(1.15090197841514,-1.,-1.7762742255701));
#32727=CARTESIAN_POINT('Ctrl Pts',(1.15090197841514,1.,-1.7762742255701));
#32728=CARTESIAN_POINT('Ctrl Pts',(1.1454385822692,-1.,-1.77313777896194));
#32729=CARTESIAN_POINT('Ctrl Pts',(1.1454385822692,1.,-1.77313777896194));
#32730=CARTESIAN_POINT('Ctrl Pts',(1.14000548336975,-1.,-1.76997111386769));
#32731=CARTESIAN_POINT('Ctrl Pts',(1.14000548336975,1.,-1.76997111386769));
#32732=CARTESIAN_POINT('Ctrl Pts',(1.1346029180462,-1.,-1.76677384551862));
#32733=CARTESIAN_POINT('Ctrl Pts',(1.1346029180462,1.,-1.76677384551862));
#32734=CARTESIAN_POINT('Ctrl Pts',(1.12923123555075,-1.,-1.7635457196617));
#32735=CARTESIAN_POINT('Ctrl Pts',(1.12923123555075,1.,-1.7635457196617));
#32736=CARTESIAN_POINT('Ctrl Pts',(1.12389096855086,-1.,-1.76028671825096));
#32737=CARTESIAN_POINT('Ctrl Pts',(1.12389096855086,1.,-1.76028671825096));
#32738=CARTESIAN_POINT('Ctrl Pts',(1.11858293216763,-1.,-1.75699720772105));
#32739=CARTESIAN_POINT('Ctrl Pts',(1.11858293216763,1.,-1.75699720772105));
#32740=CARTESIAN_POINT('Ctrl Pts',(1.11330807582551,-1.,-1.7536777209463));
#32741=CARTESIAN_POINT('Ctrl Pts',(1.11330807582551,1.,-1.7536777209463));
#32742=CARTESIAN_POINT('Ctrl Pts',(1.10806728183007,-1.,-1.7503286607592));
#32743=CARTESIAN_POINT('Ctrl Pts',(1.10806728183007,1.,-1.7503286607592));
#32744=CARTESIAN_POINT('Ctrl Pts',(1.10286118991143,-1.,-1.74695004214923));
#32745=CARTESIAN_POINT('Ctrl Pts',(1.10286118991143,1.,-1.74695004214923));
#32746=CARTESIAN_POINT('Ctrl Pts',(1.09768999241225,-1.,-1.74354119236208));
#32747=CARTESIAN_POINT('Ctrl Pts',(1.09768999241225,1.,-1.74354119236208));
#32748=CARTESIAN_POINT('Ctrl Pts',(1.09255329056493,-1.,-1.74010053962247));
#32749=CARTESIAN_POINT('Ctrl Pts',(1.09255329056493,1.,-1.74010053962247));
#32750=CARTESIAN_POINT('Ctrl Pts',(1.08745056285427,-1.,-1.73662628326091));
#32751=CARTESIAN_POINT('Ctrl Pts',(1.08745056285427,1.,-1.73662628326091));
#32752=CARTESIAN_POINT('Ctrl Pts',(1.08238162784749,-1.,-1.73311705663407));
#32753=CARTESIAN_POINT('Ctrl Pts',(1.08238162784749,1.,-1.73311705663407));
#32754=CARTESIAN_POINT('Ctrl Pts',(1.0773470373727,-1.,-1.72957248977424));
#32755=CARTESIAN_POINT('Ctrl Pts',(1.0773470373727,1.,-1.72957248977424));
#32756=CARTESIAN_POINT('Ctrl Pts',(1.07234866990252,-1.,-1.72599406198488));
#32757=CARTESIAN_POINT('Ctrl Pts',(1.07234866990252,1.,-1.72599406198488));
#32758=CARTESIAN_POINT('Ctrl Pts',(1.06738966975462,-1.,-1.72238500928453));
#32759=CARTESIAN_POINT('Ctrl Pts',(1.06738966975462,1.,-1.72238500928453));
#32760=CARTESIAN_POINT('Ctrl Pts',(1.06247324680647,-1.,-1.71874858456904));
#32761=CARTESIAN_POINT('Ctrl Pts',(1.06247324680647,1.,-1.71874858456904));
#32762=CARTESIAN_POINT('Ctrl Pts',(1.05760163192479,-1.,-1.7150865442702));
#32763=CARTESIAN_POINT('Ctrl Pts',(1.05760163192479,1.,-1.7150865442702));
#32764=CARTESIAN_POINT('Ctrl Pts',(1.05277517202855,-1.,-1.71139783543989));
#32765=CARTESIAN_POINT('Ctrl Pts',(1.05277517202855,1.,-1.71139783543989));
#32766=CARTESIAN_POINT('Ctrl Pts',(1.04799085404995,-1.,-1.70767646263649));
#32767=CARTESIAN_POINT('Ctrl Pts',(1.04799085404995,1.,-1.70767646263649));
#32768=CARTESIAN_POINT('Ctrl Pts',(1.04324363334554,-1.,-1.70391338707982));
#32769=CARTESIAN_POINT('Ctrl Pts',(1.04324363334554,1.,-1.70391338707982));
#32770=CARTESIAN_POINT('Ctrl Pts',(1.03852922490789,-1.,-1.70010052930962));
#32771=CARTESIAN_POINT('Ctrl Pts',(1.03852922490789,1.,-1.70010052930962));
#32772=CARTESIAN_POINT('Ctrl Pts',(1.03384646003588,-1.,-1.69623414782771));
#32773=CARTESIAN_POINT('Ctrl Pts',(1.03384646003588,1.,-1.69623414782771));
#32774=CARTESIAN_POINT('Ctrl Pts',(1.02919977579147,-1.,-1.69231840863458));
#32775=CARTESIAN_POINT('Ctrl Pts',(1.02919977579147,1.,-1.69231840863458));
#32776=CARTESIAN_POINT('Ctrl Pts',(1.02460180535255,-1.,-1.68836910178447));
#32777=CARTESIAN_POINT('Ctrl Pts',(1.02460180535255,1.,-1.68836910178447));
#32778=CARTESIAN_POINT('Ctrl Pts',(1.02006795074201,-1.,-1.68440578021706));
#32779=CARTESIAN_POINT('Ctrl Pts',(1.02006795074201,1.,-1.68440578021706));
#32780=CARTESIAN_POINT('Ctrl Pts',(1.01561026162773,-1.,-1.68044289894798));
#32781=CARTESIAN_POINT('Ctrl Pts',(1.01561026162773,1.,-1.68044289894798));
#32782=CARTESIAN_POINT('Ctrl Pts',(1.01123236493511,-1.,-1.67648246776464));
#32783=CARTESIAN_POINT('Ctrl Pts',(1.01123236493511,1.,-1.67648246776464));
#32784=CARTESIAN_POINT('Ctrl Pts',(1.00692206696414,-1.,-1.67250335383293));
#32785=CARTESIAN_POINT('Ctrl Pts',(1.00692206696414,1.,-1.67250335383293));
#32786=CARTESIAN_POINT('Ctrl Pts',(1.00265091003727,-1.,-1.66846059277303));
#32787=CARTESIAN_POINT('Ctrl Pts',(1.00265091003727,1.,-1.66846059277303));
#32788=CARTESIAN_POINT('Ctrl Pts',(0.998389654952757,-1.,-1.66430758030376));
#32789=CARTESIAN_POINT('Ctrl Pts',(0.998389654952757,1.,-1.66430758030376));
#32790=CARTESIAN_POINT('Ctrl Pts',(0.994121836661305,-1.,-1.66001553809947));
#32791=CARTESIAN_POINT('Ctrl Pts',(0.994121836661305,1.,-1.66001553809947));
#32792=CARTESIAN_POINT('Ctrl Pts',(0.989855627854164,-1.,-1.65559044289699));
#32793=CARTESIAN_POINT('Ctrl Pts',(0.989855627854164,1.,-1.65559044289699));
#32794=CARTESIAN_POINT('Ctrl Pts',(0.98564262292082,-1.,-1.65110016612638));
#32795=CARTESIAN_POINT('Ctrl Pts',(0.98564262292082,1.,-1.65110016612638));
#32796=CARTESIAN_POINT('Ctrl Pts',(0.981562530939489,-1.,-1.64665139190656));
#32797=CARTESIAN_POINT('Ctrl Pts',(0.981562530939489,1.,-1.64665139190656));
#32798=CARTESIAN_POINT('Ctrl Pts',(0.977689794119416,-1.,-1.64233990826687));
#32799=CARTESIAN_POINT('Ctrl Pts',(0.977689794119416,1.,-1.64233990826687));
#32800=CARTESIAN_POINT('Ctrl Pts',(0.974066058287418,-1.,-1.63820952658144));
#32801=CARTESIAN_POINT('Ctrl Pts',(0.974066058287418,1.,-1.63820952658144));
#32802=CARTESIAN_POINT('Ctrl Pts',(0.970669715997509,-1.,-1.63420665729798));
#32803=CARTESIAN_POINT('Ctrl Pts',(0.970669715997509,1.,-1.63420665729798));
#32804=CARTESIAN_POINT('Ctrl Pts',(0.967387853230345,-1.,-1.63013849959462));
#32805=CARTESIAN_POINT('Ctrl Pts',(0.967387853230345,1.,-1.63013849959462));
#32806=CARTESIAN_POINT('Ctrl Pts',(0.964046107040535,-1.,-1.62571930670187));
#32807=CARTESIAN_POINT('Ctrl Pts',(0.964046107040535,1.,-1.62571930670187));
#32808=CARTESIAN_POINT('Ctrl Pts',(0.960438326101728,-1.,-1.62061638140221));
#32809=CARTESIAN_POINT('Ctrl Pts',(0.960438326101728,1.,-1.62061638140221));
#32810=CARTESIAN_POINT('Ctrl Pts',(0.95635442292067,-1.,-1.61449324337085));
#32811=CARTESIAN_POINT('Ctrl Pts',(0.95635442292067,1.,-1.61449324337085));
#32812=CARTESIAN_POINT('Ctrl Pts',(0.951613284356035,-1.,-1.60706069896936));
#32813=CARTESIAN_POINT('Ctrl Pts',(0.951613284356035,1.,-1.60706069896936));
#32814=CARTESIAN_POINT('Ctrl Pts',(0.946078063315257,-1.,-1.59810042043673));
#32815=CARTESIAN_POINT('Ctrl Pts',(0.946078063315257,1.,-1.59810042043673));
#32816=CARTESIAN_POINT('Ctrl Pts',(0.939646377893399,-1.,-1.58744937487176));
#32817=CARTESIAN_POINT('Ctrl Pts',(0.939646377893399,1.,-1.58744937487176));
#32818=CARTESIAN_POINT('Ctrl Pts',(0.932246680108685,-1.,-1.57499388382243));
#32819=CARTESIAN_POINT('Ctrl Pts',(0.932246680108685,1.,-1.57499388382243));
#32820=CARTESIAN_POINT('Ctrl Pts',(0.923832188944341,-1.,-1.56065988578893));
#32821=CARTESIAN_POINT('Ctrl Pts',(0.923832188944341,1.,-1.56065988578893));
#32822=CARTESIAN_POINT('Ctrl Pts',(0.914375919026456,-1.,-1.54440491149498));
#32823=CARTESIAN_POINT('Ctrl Pts',(0.914375919026456,1.,-1.54440491149498));
#32824=CARTESIAN_POINT('Ctrl Pts',(0.905967409625651,-1.,-1.52984849887993));
#32825=CARTESIAN_POINT('Ctrl Pts',(0.905967409625651,1.,-1.52984849887993));
#32826=CARTESIAN_POINT('Ctrl Pts',(0.89918504748351,-1.,-1.51805569590094));
#32827=CARTESIAN_POINT('Ctrl Pts',(0.89918504748351,1.,-1.51805569590094));
#32828=CARTESIAN_POINT('Ctrl Pts',(0.894452006964543,-1.,-1.50980486806688));
#32829=CARTESIAN_POINT('Ctrl Pts',(0.894452006964543,1.,-1.50980486806688));
#32830=CARTESIAN_POINT('Ctrl Pts',(0.892032620296855,-1.,-1.5055822144029));
#32831=CARTESIAN_POINT('Ctrl Pts',(0.892032620296855,1.,-1.5055822144029));
#32832=CARTESIAN_POINT('',(1.23627494547115,1.,-1.81978687191668));
#32833=CARTESIAN_POINT('Ctrl Pts',(1.23627494547115,1.,-1.81978687191668));
#32834=CARTESIAN_POINT('Ctrl Pts',(1.23509651170476,1.,-1.81925017193666));
#32835=CARTESIAN_POINT('Ctrl Pts',(1.2327422452705,1.,-1.81817389921279));
#32836=CARTESIAN_POINT('Ctrl Pts',(1.2292186489137,1.,-1.8165508718364));
#32837=CARTESIAN_POINT('Ctrl Pts',(1.2245361330495,1.,-1.81436959210434));
#32838=CARTESIAN_POINT('Ctrl Pts',(1.21870906103557,1.,-1.81161420806656));
#32839=CARTESIAN_POINT('Ctrl Pts',(1.21290815708314,1.,-1.80882996917129));
#32840=CARTESIAN_POINT('Ctrl Pts',(1.20713356605475,1.,-1.80601678480707));
#32841=CARTESIAN_POINT('Ctrl Pts',(1.20138548938974,1.,-1.80317454838603));
#32842=CARTESIAN_POINT('Ctrl Pts',(1.19566418930242,1.,-1.80030314369879));
#32843=CARTESIAN_POINT('Ctrl Pts',(1.18996997934445,1.,-1.79740245923478));
#32844=CARTESIAN_POINT('Ctrl Pts',(1.18430321697432,1.,-1.79447240321515));
#32845=CARTESIAN_POINT('Ctrl Pts',(1.17866429440809,1.,-1.79151291552689));
#32846=CARTESIAN_POINT('Ctrl Pts',(1.17305363177328,1.,-1.78852398877617));
#32847=CARTESIAN_POINT('Ctrl Pts',(1.16747166312303,1.,-1.78550566040443));
#32848=CARTESIAN_POINT('Ctrl Pts',(1.16191881298499,1.,-1.78245795881009));
#32849=CARTESIAN_POINT('Ctrl Pts',(1.15639547194698,1.,-1.77938085564275));
#32850=CARTESIAN_POINT('Ctrl Pts',(1.15090197841514,1.,-1.7762742255701));
#32851=CARTESIAN_POINT('Ctrl Pts',(1.1454385822692,1.,-1.77313777896194));
#32852=CARTESIAN_POINT('Ctrl Pts',(1.14000548336975,1.,-1.76997111386769));
#32853=CARTESIAN_POINT('Ctrl Pts',(1.1346029180462,1.,-1.76677384551862));
#32854=CARTESIAN_POINT('Ctrl Pts',(1.12923123555075,1.,-1.7635457196617));
#32855=CARTESIAN_POINT('Ctrl Pts',(1.12389096855086,1.,-1.76028671825096));
#32856=CARTESIAN_POINT('Ctrl Pts',(1.11858293216763,1.,-1.75699720772105));
#32857=CARTESIAN_POINT('Ctrl Pts',(1.11330807582551,1.,-1.7536777209463));
#32858=CARTESIAN_POINT('Ctrl Pts',(1.10806728183007,1.,-1.7503286607592));
#32859=CARTESIAN_POINT('Ctrl Pts',(1.10286118991143,1.,-1.74695004214923));
#32860=CARTESIAN_POINT('Ctrl Pts',(1.09768999241225,1.,-1.74354119236208));
#32861=CARTESIAN_POINT('Ctrl Pts',(1.09255329056493,1.,-1.74010053962247));
#32862=CARTESIAN_POINT('Ctrl Pts',(1.08745056285427,1.,-1.73662628326091));
#32863=CARTESIAN_POINT('Ctrl Pts',(1.08238162784749,1.,-1.73311705663407));
#32864=CARTESIAN_POINT('Ctrl Pts',(1.0773470373727,1.,-1.72957248977424));
#32865=CARTESIAN_POINT('Ctrl Pts',(1.07234866990252,1.,-1.72599406198488));
#32866=CARTESIAN_POINT('Ctrl Pts',(1.06738966975462,1.,-1.72238500928453));
#32867=CARTESIAN_POINT('Ctrl Pts',(1.06247324680647,1.,-1.71874858456904));
#32868=CARTESIAN_POINT('Ctrl Pts',(1.05760163192479,1.,-1.7150865442702));
#32869=CARTESIAN_POINT('Ctrl Pts',(1.05277517202855,1.,-1.71139783543989));
#32870=CARTESIAN_POINT('Ctrl Pts',(1.04799085404995,1.,-1.70767646263649));
#32871=CARTESIAN_POINT('Ctrl Pts',(1.04324363334554,1.,-1.70391338707982));
#32872=CARTESIAN_POINT('Ctrl Pts',(1.03852922490789,1.,-1.70010052930962));
#32873=CARTESIAN_POINT('Ctrl Pts',(1.03384646003588,1.,-1.69623414782771));
#32874=CARTESIAN_POINT('Ctrl Pts',(1.02919977579147,1.,-1.69231840863458));
#32875=CARTESIAN_POINT('Ctrl Pts',(1.02460180535255,1.,-1.68836910178447));
#32876=CARTESIAN_POINT('Ctrl Pts',(1.02006795074201,1.,-1.68440578021706));
#32877=CARTESIAN_POINT('Ctrl Pts',(1.01561026162773,1.,-1.68044289894798));
#32878=CARTESIAN_POINT('Ctrl Pts',(1.01123236493511,1.,-1.67648246776464));
#32879=CARTESIAN_POINT('Ctrl Pts',(1.00692206696414,1.,-1.67250335383293));
#32880=CARTESIAN_POINT('Ctrl Pts',(1.00265091003727,1.,-1.66846059277303));
#32881=CARTESIAN_POINT('Ctrl Pts',(0.998389654952757,1.,-1.66430758030376));
#32882=CARTESIAN_POINT('Ctrl Pts',(0.994121836661305,1.,-1.66001553809947));
#32883=CARTESIAN_POINT('Ctrl Pts',(0.989855627854164,1.,-1.65559044289699));
#32884=CARTESIAN_POINT('Ctrl Pts',(0.98564262292082,1.,-1.65110016612638));
#32885=CARTESIAN_POINT('Ctrl Pts',(0.981562530939489,1.,-1.64665139190656));
#32886=CARTESIAN_POINT('Ctrl Pts',(0.977689794119416,1.,-1.64233990826687));
#32887=CARTESIAN_POINT('Ctrl Pts',(0.974066058287418,1.,-1.63820952658144));
#32888=CARTESIAN_POINT('Ctrl Pts',(0.970669715997509,1.,-1.63420665729798));
#32889=CARTESIAN_POINT('Ctrl Pts',(0.967387853230345,1.,-1.63013849959462));
#32890=CARTESIAN_POINT('Ctrl Pts',(0.964046107040535,1.,-1.62571930670187));
#32891=CARTESIAN_POINT('Ctrl Pts',(0.960438326101728,1.,-1.62061638140221));
#32892=CARTESIAN_POINT('Ctrl Pts',(0.95635442292067,1.,-1.61449324337085));
#32893=CARTESIAN_POINT('Ctrl Pts',(0.951613284356035,1.,-1.60706069896936));
#32894=CARTESIAN_POINT('Ctrl Pts',(0.946078063315257,1.,-1.59810042043673));
#32895=CARTESIAN_POINT('Ctrl Pts',(0.939646377893399,1.,-1.58744937487176));
#32896=CARTESIAN_POINT('Ctrl Pts',(0.932246680108685,1.,-1.57499388382243));
#32897=CARTESIAN_POINT('Ctrl Pts',(0.923832188944341,1.,-1.56065988578893));
#32898=CARTESIAN_POINT('Ctrl Pts',(0.914375919026456,1.,-1.54440491149498));
#32899=CARTESIAN_POINT('Ctrl Pts',(0.905967409625651,1.,-1.52984849887993));
#32900=CARTESIAN_POINT('Ctrl Pts',(0.89918504748351,1.,-1.51805569590094));
#32901=CARTESIAN_POINT('Ctrl Pts',(0.894452006964543,1.,-1.50980486806688));
#32902=CARTESIAN_POINT('Ctrl Pts',(0.892032620296855,1.,-1.5055822144029));
#32903=CARTESIAN_POINT('',(1.23627494547115,0.,-1.81978687191668));
#32904=CARTESIAN_POINT('Origin',(1.34869019493419,0.,-1.73811241238545));
#32905=CARTESIAN_POINT('',(1.34869019493419,1.,-1.73811241238545));
#32906=CARTESIAN_POINT('',(1.23627494547115,1.,-1.81978687191668));
#32907=CARTESIAN_POINT('',(1.34869019493419,0.,-1.73811241238545));
#32908=CARTESIAN_POINT('Ctrl Pts',(1.15624053661742,-1.,-1.31362392696032));
#32909=CARTESIAN_POINT('Ctrl Pts',(1.15624053661742,1.,-1.31362392696032));
#32910=CARTESIAN_POINT('Ctrl Pts',(1.15950888730809,-1.,-1.31722977216397));
#32911=CARTESIAN_POINT('Ctrl Pts',(1.15950888730809,1.,-1.31722977216397));
#32912=CARTESIAN_POINT('Ctrl Pts',(1.16589330093588,-1.,-1.32428080721772));
#32913=CARTESIAN_POINT('Ctrl Pts',(1.16589330093588,1.,-1.32428080721772));
#32914=CARTESIAN_POINT('Ctrl Pts',(1.17501305789857,-1.,-1.33437539347008));
#32915=CARTESIAN_POINT('Ctrl Pts',(1.17501305789857,1.,-1.33437539347008));
#32916=CARTESIAN_POINT('Ctrl Pts',(1.18625865667441,-1.,-1.34687054001093));
#32917=CARTESIAN_POINT('Ctrl Pts',(1.18625865667441,1.,-1.34687054001093));
#32918=CARTESIAN_POINT('Ctrl Pts',(1.1987959077932,-1.,-1.36088705043885));
#32919=CARTESIAN_POINT('Ctrl Pts',(1.1987959077932,1.,-1.36088705043885));
#32920=CARTESIAN_POINT('Ctrl Pts',(1.20982812925645,-1.,-1.37331915607905));
#32921=CARTESIAN_POINT('Ctrl Pts',(1.20982812925645,1.,-1.37331915607905));
#32922=CARTESIAN_POINT('Ctrl Pts',(1.21938737280852,-1.,-1.38420564527715));
#32923=CARTESIAN_POINT('Ctrl Pts',(1.21938737280852,1.,-1.38420564527715));
#32924=CARTESIAN_POINT('Ctrl Pts',(1.22752961899387,-1.,-1.39361389568796));
#32925=CARTESIAN_POINT('Ctrl Pts',(1.22752961899387,1.,-1.39361389568796));
#32926=CARTESIAN_POINT('Ctrl Pts',(1.23434087290423,-1.,-1.40164708206106));
#32927=CARTESIAN_POINT('Ctrl Pts',(1.23434087290423,1.,-1.40164708206106));
#32928=CARTESIAN_POINT('Ctrl Pts',(1.23994455029534,-1.,-1.40845295531283));
#32929=CARTESIAN_POINT('Ctrl Pts',(1.23994455029534,1.,-1.40845295531283));
#32930=CARTESIAN_POINT('Ctrl Pts',(1.24450600513056,-1.,-1.41422913175179));
#32931=CARTESIAN_POINT('Ctrl Pts',(1.24450600513056,1.,-1.41422913175179));
#32932=CARTESIAN_POINT('Ctrl Pts',(1.24824430986571,-1.,-1.41923722596025));
#32933=CARTESIAN_POINT('Ctrl Pts',(1.24824430986571,1.,-1.41923722596025));
#32934=CARTESIAN_POINT('Ctrl Pts',(1.2514145557001,-1.,-1.42378102115575));
#32935=CARTESIAN_POINT('Ctrl Pts',(1.2514145557001,1.,-1.42378102115575));
#32936=CARTESIAN_POINT('Ctrl Pts',(1.25426945222639,-1.,-1.42815938799387));
#32937=CARTESIAN_POINT('Ctrl Pts',(1.25426945222639,1.,-1.42815938799387));
#32938=CARTESIAN_POINT('Ctrl Pts',(1.25702687965755,-1.,-1.43262645609691));
#32939=CARTESIAN_POINT('Ctrl Pts',(1.25702687965755,1.,-1.43262645609691));
#32940=CARTESIAN_POINT('Ctrl Pts',(1.25983531012005,-1.,-1.43734919180848));
#32941=CARTESIAN_POINT('Ctrl Pts',(1.25983531012005,1.,-1.43734919180848));
#32942=CARTESIAN_POINT('Ctrl Pts',(1.26273903323858,-1.,-1.44236470511303));
#32943=CARTESIAN_POINT('Ctrl Pts',(1.26273903323858,1.,-1.44236470511303));
#32944=CARTESIAN_POINT('Ctrl Pts',(1.26570925118868,-1.,-1.44761985001662));
#32945=CARTESIAN_POINT('Ctrl Pts',(1.26570925118868,1.,-1.44761985001662));
#32946=CARTESIAN_POINT('Ctrl Pts',(1.2686778680489,-1.,-1.45301422764247));
#32947=CARTESIAN_POINT('Ctrl Pts',(1.2686778680489,1.,-1.45301422764247));
#32948=CARTESIAN_POINT('Ctrl Pts',(1.27156805265289,-1.,-1.45843906294697));
#32949=CARTESIAN_POINT('Ctrl Pts',(1.27156805265289,1.,-1.45843906294697));
#32950=CARTESIAN_POINT('Ctrl Pts',(1.27433119897822,-1.,-1.46382431332476));
#32951=CARTESIAN_POINT('Ctrl Pts',(1.27433119897822,1.,-1.46382431332476));
#32952=CARTESIAN_POINT('Ctrl Pts',(1.27696414831089,-1.,-1.46916035917133));
#32953=CARTESIAN_POINT('Ctrl Pts',(1.27696414831089,1.,-1.46916035917133));
#32954=CARTESIAN_POINT('Ctrl Pts',(1.2794891824849,-1.,-1.4744717526707));
#32955=CARTESIAN_POINT('Ctrl Pts',(1.2794891824849,1.,-1.4744717526707));
#32956=CARTESIAN_POINT('Ctrl Pts',(1.28194158939517,-1.,-1.47980070347096));
#32957=CARTESIAN_POINT('Ctrl Pts',(1.28194158939517,1.,-1.47980070347096));
#32958=CARTESIAN_POINT('Ctrl Pts',(1.28435533880201,-1.,-1.4851881711891));
#32959=CARTESIAN_POINT('Ctrl Pts',(1.28435533880201,1.,-1.4851881711891));
#32960=CARTESIAN_POINT('Ctrl Pts',(1.2867467611644,-1.,-1.4906522831278));
#32961=CARTESIAN_POINT('Ctrl Pts',(1.2867467611644,1.,-1.4906522831278));
#32962=CARTESIAN_POINT('Ctrl Pts',(1.28911506584254,-1.,-1.49618896881754));
#32963=CARTESIAN_POINT('Ctrl Pts',(1.28911506584254,1.,-1.49618896881754));
#32964=CARTESIAN_POINT('Ctrl Pts',(1.29145022885181,-1.,-1.50178230149776));
#32965=CARTESIAN_POINT('Ctrl Pts',(1.29145022885181,1.,-1.50178230149776));
#32966=CARTESIAN_POINT('Ctrl Pts',(1.29373841372842,-1.,-1.50741159078365));
#32967=CARTESIAN_POINT('Ctrl Pts',(1.29373841372842,1.,-1.50741159078365));
#32968=CARTESIAN_POINT('Ctrl Pts',(1.29596850710509,-1.,-1.51305994241402));
#32969=CARTESIAN_POINT('Ctrl Pts',(1.29596850710509,1.,-1.51305994241402));
#32970=CARTESIAN_POINT('Ctrl Pts',(1.29813791800747,-1.,-1.51872184912724));
#32971=CARTESIAN_POINT('Ctrl Pts',(1.29813791800747,1.,-1.51872184912724));
#32972=CARTESIAN_POINT('Ctrl Pts',(1.30024984366328,-1.,-1.52439957861062));
#32973=CARTESIAN_POINT('Ctrl Pts',(1.30024984366328,1.,-1.52439957861062));
#32974=CARTESIAN_POINT('Ctrl Pts',(1.30231064395568,-1.,-1.53009970283891));
#32975=CARTESIAN_POINT('Ctrl Pts',(1.30231064395568,1.,-1.53009970283891));
#32976=CARTESIAN_POINT('Ctrl Pts',(1.30432735639489,-1.,-1.53582981268977));
#32977=CARTESIAN_POINT('Ctrl Pts',(1.30432735639489,1.,-1.53582981268977));
#32978=CARTESIAN_POINT('Ctrl Pts',(1.30630475189556,-1.,-1.54159462645432));
#32979=CARTESIAN_POINT('Ctrl Pts',(1.30630475189556,1.,-1.54159462645432));
#32980=CARTESIAN_POINT('Ctrl Pts',(1.30824393907473,-1.,-1.54739413957185));
#32981=CARTESIAN_POINT('Ctrl Pts',(1.30824393907473,1.,-1.54739413957185));
#32982=CARTESIAN_POINT('Ctrl Pts',(1.31014393684222,-1.,-1.55322568759481));
#32983=CARTESIAN_POINT('Ctrl Pts',(1.31014393684222,1.,-1.55322568759481));
#32984=CARTESIAN_POINT('Ctrl Pts',(1.31200264341696,-1.,-1.55908521254821));
#32985=CARTESIAN_POINT('Ctrl Pts',(1.31200264341696,1.,-1.55908521254821));
#32986=CARTESIAN_POINT('Ctrl Pts',(1.31381795281002,-1.,-1.56496872402353));
#32987=CARTESIAN_POINT('Ctrl Pts',(1.31381795281002,1.,-1.56496872402353));
#32988=CARTESIAN_POINT('Ctrl Pts',(1.31558903860016,-1.,-1.57087397835723));
#32989=CARTESIAN_POINT('Ctrl Pts',(1.31558903860016,1.,-1.57087397835723));
#32990=CARTESIAN_POINT('Ctrl Pts',(1.31731642317187,-1.,-1.5768005650559));
#32991=CARTESIAN_POINT('Ctrl Pts',(1.31731642317187,1.,-1.5768005650559));
#32992=CARTESIAN_POINT('Ctrl Pts',(1.31900135021432,-1.,-1.58274907898834));
#32993=CARTESIAN_POINT('Ctrl Pts',(1.31900135021432,1.,-1.58274907898834));
#32994=CARTESIAN_POINT('Ctrl Pts',(1.32064537110892,-1.,-1.58872057258245));
#32995=CARTESIAN_POINT('Ctrl Pts',(1.32064537110892,1.,-1.58872057258245));
#32996=CARTESIAN_POINT('Ctrl Pts',(1.32224985747682,-1.,-1.59471591079403));
#32997=CARTESIAN_POINT('Ctrl Pts',(1.32224985747682,1.,-1.59471591079403));
#32998=CARTESIAN_POINT('Ctrl Pts',(1.32381550858256,-1.,-1.60073511858687));
#32999=CARTESIAN_POINT('Ctrl Pts',(1.32381550858256,1.,-1.60073511858687));
#33000=CARTESIAN_POINT('Ctrl Pts',(1.32534250785782,-1.,-1.60677758290954));
#33001=CARTESIAN_POINT('Ctrl Pts',(1.32534250785782,1.,-1.60677758290954));
#33002=CARTESIAN_POINT('Ctrl Pts',(1.32683074483356,-1.,-1.6128423401575));
#33003=CARTESIAN_POINT('Ctrl Pts',(1.32683074483356,1.,-1.6128423401575));
#33004=CARTESIAN_POINT('Ctrl Pts',(1.32828000610449,-1.,-1.61892832270724));
#33005=CARTESIAN_POINT('Ctrl Pts',(1.32828000610449,1.,-1.61892832270724));
#33006=CARTESIAN_POINT('Ctrl Pts',(1.3296901950568,-1.,-1.62503464209797));
#33007=CARTESIAN_POINT('Ctrl Pts',(1.3296901950568,1.,-1.62503464209797));
#33008=CARTESIAN_POINT('Ctrl Pts',(1.33106149345645,-1.,-1.63116079730923));
#33009=CARTESIAN_POINT('Ctrl Pts',(1.33106149345645,1.,-1.63116079730923));
#33010=CARTESIAN_POINT('Ctrl Pts',(1.33239425103724,-1.,-1.63730653475089));
#33011=CARTESIAN_POINT('Ctrl Pts',(1.33239425103724,1.,-1.63730653475089));
#33012=CARTESIAN_POINT('Ctrl Pts',(1.33368890676572,-1.,-1.6434717485603));
#33013=CARTESIAN_POINT('Ctrl Pts',(1.33368890676572,1.,-1.6434717485603));
#33014=CARTESIAN_POINT('Ctrl Pts',(1.33494590467993,-1.,-1.6496563728683));
#33015=CARTESIAN_POINT('Ctrl Pts',(1.33494590467993,1.,-1.6496563728683));
#33016=CARTESIAN_POINT('Ctrl Pts',(1.33616559745172,-1.,-1.65586025952593));
#33017=CARTESIAN_POINT('Ctrl Pts',(1.33616559745172,1.,-1.65586025952593));
#33018=CARTESIAN_POINT('Ctrl Pts',(1.33734820885262,-1.,-1.66208312541983));
#33019=CARTESIAN_POINT('Ctrl Pts',(1.33734820885262,1.,-1.66208312541983));
#33020=CARTESIAN_POINT('Ctrl Pts',(1.33849388654388,-1.,-1.66832460783989));
#33021=CARTESIAN_POINT('Ctrl Pts',(1.33849388654388,1.,-1.66832460783989));
#33022=CARTESIAN_POINT('Ctrl Pts',(1.3396027347034,-1.,-1.67458429426086));
#33023=CARTESIAN_POINT('Ctrl Pts',(1.3396027347034,1.,-1.67458429426086));
#33024=CARTESIAN_POINT('Ctrl Pts',(1.34067485185203,-1.,-1.68086176030362));
#33025=CARTESIAN_POINT('Ctrl Pts',(1.34067485185203,1.,-1.68086176030362));
#33026=CARTESIAN_POINT('Ctrl Pts',(1.341710374848,-1.,-1.68715660868764));
#33027=CARTESIAN_POINT('Ctrl Pts',(1.341710374848,1.,-1.68715660868764));
#33028=CARTESIAN_POINT('Ctrl Pts',(1.34270948206319,-1.,-1.6934684849687));
#33029=CARTESIAN_POINT('Ctrl Pts',(1.34270948206319,1.,-1.6934684849687));
#33030=CARTESIAN_POINT('Ctrl Pts',(1.34367237124483,-1.,-1.69979707754427));
#33031=CARTESIAN_POINT('Ctrl Pts',(1.34367237124483,1.,-1.69979707754427));
#33032=CARTESIAN_POINT('Ctrl Pts',(1.34459924533831,-1.,-1.70614212266738));
#33033=CARTESIAN_POINT('Ctrl Pts',(1.34459924533831,1.,-1.70614212266738));
#33034=CARTESIAN_POINT('Ctrl Pts',(1.34549029589416,-1.,-1.71250340686822));
#33035=CARTESIAN_POINT('Ctrl Pts',(1.34549029589416,1.,-1.71250340686822));
#33036=CARTESIAN_POINT('Ctrl Pts',(1.34634568653227,-1.,-1.7188807715049));
#33037=CARTESIAN_POINT('Ctrl Pts',(1.34634568653227,1.,-1.7188807715049));
#33038=CARTESIAN_POINT('Ctrl Pts',(1.34716554819527,-1.,-1.72527410680674));
#33039=CARTESIAN_POINT('Ctrl Pts',(1.34716554819527,1.,-1.72527410680674));
#33040=CARTESIAN_POINT('Ctrl Pts',(1.34779309152035,-1.,-1.7304014965394));
#33041=CARTESIAN_POINT('Ctrl Pts',(1.34779309152035,1.,-1.7304014965394));
#33042=CARTESIAN_POINT('Ctrl Pts',(1.34824783112887,-1.,-1.73425417885907));
#33043=CARTESIAN_POINT('Ctrl Pts',(1.34824783112887,1.,-1.73425417885907));
#33044=CARTESIAN_POINT('Ctrl Pts',(1.34854391898045,-1.,-1.73682580585691));
#33045=CARTESIAN_POINT('Ctrl Pts',(1.34854391898045,1.,-1.73682580585691));
#33046=CARTESIAN_POINT('Ctrl Pts',(1.34869019493419,-1.,-1.73811241238545));
#33047=CARTESIAN_POINT('Ctrl Pts',(1.34869019493419,1.,-1.73811241238545));
#33048=CARTESIAN_POINT('',(1.15624053661742,1.,-1.31362392696032));
#33049=CARTESIAN_POINT('Ctrl Pts',(1.15624053661742,1.,-1.31362392696032));
#33050=CARTESIAN_POINT('Ctrl Pts',(1.15950888730809,1.,-1.31722977216397));
#33051=CARTESIAN_POINT('Ctrl Pts',(1.16589330093588,1.,-1.32428080721772));
#33052=CARTESIAN_POINT('Ctrl Pts',(1.17501305789857,1.,-1.33437539347008));
#33053=CARTESIAN_POINT('Ctrl Pts',(1.18625865667441,1.,-1.34687054001093));
#33054=CARTESIAN_POINT('Ctrl Pts',(1.1987959077932,1.,-1.36088705043885));
#33055=CARTESIAN_POINT('Ctrl Pts',(1.20982812925645,1.,-1.37331915607905));
#33056=CARTESIAN_POINT('Ctrl Pts',(1.21938737280852,1.,-1.38420564527715));
#33057=CARTESIAN_POINT('Ctrl Pts',(1.22752961899387,1.,-1.39361389568796));
#33058=CARTESIAN_POINT('Ctrl Pts',(1.23434087290423,1.,-1.40164708206106));
#33059=CARTESIAN_POINT('Ctrl Pts',(1.23994455029534,1.,-1.40845295531283));
#33060=CARTESIAN_POINT('Ctrl Pts',(1.24450600513056,1.,-1.41422913175179));
#33061=CARTESIAN_POINT('Ctrl Pts',(1.24824430986571,1.,-1.41923722596025));
#33062=CARTESIAN_POINT('Ctrl Pts',(1.2514145557001,1.,-1.42378102115575));
#33063=CARTESIAN_POINT('Ctrl Pts',(1.25426945222639,1.,-1.42815938799387));
#33064=CARTESIAN_POINT('Ctrl Pts',(1.25702687965755,1.,-1.43262645609691));
#33065=CARTESIAN_POINT('Ctrl Pts',(1.25983531012005,1.,-1.43734919180848));
#33066=CARTESIAN_POINT('Ctrl Pts',(1.26273903323858,1.,-1.44236470511303));
#33067=CARTESIAN_POINT('Ctrl Pts',(1.26570925118868,1.,-1.44761985001662));
#33068=CARTESIAN_POINT('Ctrl Pts',(1.2686778680489,1.,-1.45301422764247));
#33069=CARTESIAN_POINT('Ctrl Pts',(1.27156805265289,1.,-1.45843906294697));
#33070=CARTESIAN_POINT('Ctrl Pts',(1.27433119897822,1.,-1.46382431332476));
#33071=CARTESIAN_POINT('Ctrl Pts',(1.27696414831089,1.,-1.46916035917133));
#33072=CARTESIAN_POINT('Ctrl Pts',(1.2794891824849,1.,-1.4744717526707));
#33073=CARTESIAN_POINT('Ctrl Pts',(1.28194158939517,1.,-1.47980070347096));
#33074=CARTESIAN_POINT('Ctrl Pts',(1.28435533880201,1.,-1.4851881711891));
#33075=CARTESIAN_POINT('Ctrl Pts',(1.2867467611644,1.,-1.4906522831278));
#33076=CARTESIAN_POINT('Ctrl Pts',(1.28911506584254,1.,-1.49618896881754));
#33077=CARTESIAN_POINT('Ctrl Pts',(1.29145022885181,1.,-1.50178230149776));
#33078=CARTESIAN_POINT('Ctrl Pts',(1.29373841372842,1.,-1.50741159078365));
#33079=CARTESIAN_POINT('Ctrl Pts',(1.29596850710509,1.,-1.51305994241402));
#33080=CARTESIAN_POINT('Ctrl Pts',(1.29813791800747,1.,-1.51872184912724));
#33081=CARTESIAN_POINT('Ctrl Pts',(1.30024984366328,1.,-1.52439957861062));
#33082=CARTESIAN_POINT('Ctrl Pts',(1.30231064395568,1.,-1.53009970283891));
#33083=CARTESIAN_POINT('Ctrl Pts',(1.30432735639489,1.,-1.53582981268977));
#33084=CARTESIAN_POINT('Ctrl Pts',(1.30630475189556,1.,-1.54159462645432));
#33085=CARTESIAN_POINT('Ctrl Pts',(1.30824393907473,1.,-1.54739413957185));
#33086=CARTESIAN_POINT('Ctrl Pts',(1.31014393684222,1.,-1.55322568759481));
#33087=CARTESIAN_POINT('Ctrl Pts',(1.31200264341696,1.,-1.55908521254821));
#33088=CARTESIAN_POINT('Ctrl Pts',(1.31381795281002,1.,-1.56496872402353));
#33089=CARTESIAN_POINT('Ctrl Pts',(1.31558903860016,1.,-1.57087397835723));
#33090=CARTESIAN_POINT('Ctrl Pts',(1.31731642317187,1.,-1.5768005650559));
#33091=CARTESIAN_POINT('Ctrl Pts',(1.31900135021432,1.,-1.58274907898834));
#33092=CARTESIAN_POINT('Ctrl Pts',(1.32064537110892,1.,-1.58872057258245));
#33093=CARTESIAN_POINT('Ctrl Pts',(1.32224985747682,1.,-1.59471591079403));
#33094=CARTESIAN_POINT('Ctrl Pts',(1.32381550858256,1.,-1.60073511858687));
#33095=CARTESIAN_POINT('Ctrl Pts',(1.32534250785782,1.,-1.60677758290954));
#33096=CARTESIAN_POINT('Ctrl Pts',(1.32683074483356,1.,-1.6128423401575));
#33097=CARTESIAN_POINT('Ctrl Pts',(1.32828000610449,1.,-1.61892832270724));
#33098=CARTESIAN_POINT('Ctrl Pts',(1.3296901950568,1.,-1.62503464209797));
#33099=CARTESIAN_POINT('Ctrl Pts',(1.33106149345645,1.,-1.63116079730923));
#33100=CARTESIAN_POINT('Ctrl Pts',(1.33239425103724,1.,-1.63730653475089));
#33101=CARTESIAN_POINT('Ctrl Pts',(1.33368890676572,1.,-1.6434717485603));
#33102=CARTESIAN_POINT('Ctrl Pts',(1.33494590467993,1.,-1.6496563728683));
#33103=CARTESIAN_POINT('Ctrl Pts',(1.33616559745172,1.,-1.65586025952593));
#33104=CARTESIAN_POINT('Ctrl Pts',(1.33734820885262,1.,-1.66208312541983));
#33105=CARTESIAN_POINT('Ctrl Pts',(1.33849388654388,1.,-1.66832460783989));
#33106=CARTESIAN_POINT('Ctrl Pts',(1.3396027347034,1.,-1.67458429426086));
#33107=CARTESIAN_POINT('Ctrl Pts',(1.34067485185203,1.,-1.68086176030362));
#33108=CARTESIAN_POINT('Ctrl Pts',(1.341710374848,1.,-1.68715660868764));
#33109=CARTESIAN_POINT('Ctrl Pts',(1.34270948206319,1.,-1.6934684849687));
#33110=CARTESIAN_POINT('Ctrl Pts',(1.34367237124483,1.,-1.69979707754427));
#33111=CARTESIAN_POINT('Ctrl Pts',(1.34459924533831,1.,-1.70614212266738));
#33112=CARTESIAN_POINT('Ctrl Pts',(1.34549029589416,1.,-1.71250340686822));
#33113=CARTESIAN_POINT('Ctrl Pts',(1.34634568653227,1.,-1.7188807715049));
#33114=CARTESIAN_POINT('Ctrl Pts',(1.34716554819527,1.,-1.72527410680674));
#33115=CARTESIAN_POINT('Ctrl Pts',(1.34779309152035,1.,-1.7304014965394));
#33116=CARTESIAN_POINT('Ctrl Pts',(1.34824783112887,1.,-1.73425417885907));
#33117=CARTESIAN_POINT('Ctrl Pts',(1.34854391898045,1.,-1.73682580585691));
#33118=CARTESIAN_POINT('Ctrl Pts',(1.34869019493419,1.,-1.73811241238545));
#33119=CARTESIAN_POINT('',(1.15624053661742,0.,-1.31362392696032));
#33120=CARTESIAN_POINT('Origin',(0.,0.,0.));
#33121=CARTESIAN_POINT('',(1.31362392696032,1.,-1.15624053661742));
#33122=CARTESIAN_POINT('Origin',(0.,1.,0.));
#33123=CARTESIAN_POINT('',(1.31362392696032,0.,-1.15624053661742));
#33124=CARTESIAN_POINT('Ctrl Pts',(1.73811241238545,-1.,-1.34869019493419));
#33125=CARTESIAN_POINT('Ctrl Pts',(1.73811241238545,1.,-1.34869019493419));
#33126=CARTESIAN_POINT('Ctrl Pts',(1.73682580585819,-1.,-1.34854391898145));
#33127=CARTESIAN_POINT('Ctrl Pts',(1.73682580585819,1.,-1.34854391898145));
#33128=CARTESIAN_POINT('Ctrl Pts',(1.73425417886254,-1.,-1.34824783113158));
#33129=CARTESIAN_POINT('Ctrl Pts',(1.73425417886254,1.,-1.34824783113158));
#33130=CARTESIAN_POINT('Ctrl Pts',(1.73040149654497,-1.,-1.3477930915247));
#33131=CARTESIAN_POINT('Ctrl Pts',(1.73040149654497,1.,-1.3477930915247));
#33132=CARTESIAN_POINT('Ctrl Pts',(1.72527410681298,-1.,-1.34716554820013));
#33133=CARTESIAN_POINT('Ctrl Pts',(1.72527410681298,1.,-1.34716554820013));
#33134=CARTESIAN_POINT('Ctrl Pts',(1.7188807715095,-1.,-1.34634568653586));
#33135=CARTESIAN_POINT('Ctrl Pts',(1.7188807715095,1.,-1.34634568653586));
#33136=CARTESIAN_POINT('Ctrl Pts',(1.71250340687011,-1.,-1.34549029589563));
#33137=CARTESIAN_POINT('Ctrl Pts',(1.71250340687011,1.,-1.34549029589563));
#33138=CARTESIAN_POINT('Ctrl Pts',(1.70614212266676,-1.,-1.34459924533783));
#33139=CARTESIAN_POINT('Ctrl Pts',(1.70614212266676,1.,-1.34459924533783));
#33140=CARTESIAN_POINT('Ctrl Pts',(1.69979707754221,-1.,-1.34367237124322));
#33141=CARTESIAN_POINT('Ctrl Pts',(1.69979707754221,1.,-1.34367237124322));
#33142=CARTESIAN_POINT('Ctrl Pts',(1.6934684849664,-1.,-1.34270948206139));
#33143=CARTESIAN_POINT('Ctrl Pts',(1.6934684849664,1.,-1.34270948206139));
#33144=CARTESIAN_POINT('Ctrl Pts',(1.68715660868602,-1.,-1.34171037484673));
#33145=CARTESIAN_POINT('Ctrl Pts',(1.68715660868602,1.,-1.34171037484673));
#33146=CARTESIAN_POINT('Ctrl Pts',(1.68086176030308,-1.,-1.3406748518516));
#33147=CARTESIAN_POINT('Ctrl Pts',(1.68086176030308,1.,-1.3406748518516));
#33148=CARTESIAN_POINT('Ctrl Pts',(1.67458429426126,-1.,-1.33960273470372));
#33149=CARTESIAN_POINT('Ctrl Pts',(1.67458429426126,1.,-1.33960273470372));
#33150=CARTESIAN_POINT('Ctrl Pts',(1.66832460784078,-1.,-1.33849388654458));
#33151=CARTESIAN_POINT('Ctrl Pts',(1.66832460784078,1.,-1.33849388654458));
#33152=CARTESIAN_POINT('Ctrl Pts',(1.66208312542073,-1.,-1.33734820885331));
#33153=CARTESIAN_POINT('Ctrl Pts',(1.66208312542073,1.,-1.33734820885331));
#33154=CARTESIAN_POINT('Ctrl Pts',(1.65586025952651,-1.,-1.33616559745217));
#33155=CARTESIAN_POINT('Ctrl Pts',(1.65586025952651,1.,-1.33616559745217));
#33156=CARTESIAN_POINT('Ctrl Pts',(1.64965637286843,-1.,-1.33494590468003));
#33157=CARTESIAN_POINT('Ctrl Pts',(1.64965637286843,1.,-1.33494590468003));
#33158=CARTESIAN_POINT('Ctrl Pts',(1.64347174856007,-1.,-1.33368890676554));
#33159=CARTESIAN_POINT('Ctrl Pts',(1.64347174856007,1.,-1.33368890676554));
#33160=CARTESIAN_POINT('Ctrl Pts',(1.63730653475049,-1.,-1.33239425103694));
#33161=CARTESIAN_POINT('Ctrl Pts',(1.63730653475049,1.,-1.33239425103694));
#33162=CARTESIAN_POINT('Ctrl Pts',(1.63116079730887,-1.,-1.33106149345618));
#33163=CARTESIAN_POINT('Ctrl Pts',(1.63116079730887,1.,-1.33106149345618));
#33164=CARTESIAN_POINT('Ctrl Pts',(1.62503464209777,-1.,-1.32969019505665));
#33165=CARTESIAN_POINT('Ctrl Pts',(1.62503464209777,1.,-1.32969019505665));
#33166=CARTESIAN_POINT('Ctrl Pts',(1.61892832270723,-1.,-1.32828000610448));
#33167=CARTESIAN_POINT('Ctrl Pts',(1.61892832270723,1.,-1.32828000610448));
#33168=CARTESIAN_POINT('Ctrl Pts',(1.61284234015762,-1.,-1.32683074483365));
#33169=CARTESIAN_POINT('Ctrl Pts',(1.61284234015762,1.,-1.32683074483365));
#33170=CARTESIAN_POINT('Ctrl Pts',(1.6067775829097,-1.,-1.32534250785794));
#33171=CARTESIAN_POINT('Ctrl Pts',(1.6067775829097,1.,-1.32534250785794));
#33172=CARTESIAN_POINT('Ctrl Pts',(1.600735118587,-1.,-1.32381550858266));
#33173=CARTESIAN_POINT('Ctrl Pts',(1.600735118587,1.,-1.32381550858266));
#33174=CARTESIAN_POINT('Ctrl Pts',(1.59471591079408,-1.,-1.32224985747686));
#33175=CARTESIAN_POINT('Ctrl Pts',(1.59471591079408,1.,-1.32224985747686));
#33176=CARTESIAN_POINT('Ctrl Pts',(1.58872057258244,-1.,-1.32064537110891));
#33177=CARTESIAN_POINT('Ctrl Pts',(1.58872057258244,1.,-1.32064537110891));
#33178=CARTESIAN_POINT('Ctrl Pts',(1.58274907898829,-1.,-1.31900135021428));
#33179=CARTESIAN_POINT('Ctrl Pts',(1.58274907898829,1.,-1.31900135021428));
#33180=CARTESIAN_POINT('Ctrl Pts',(1.57680056505585,-1.,-1.31731642317183));
#33181=CARTESIAN_POINT('Ctrl Pts',(1.57680056505585,1.,-1.31731642317183));
#33182=CARTESIAN_POINT('Ctrl Pts',(1.57087397835721,-1.,-1.31558903860015));
#33183=CARTESIAN_POINT('Ctrl Pts',(1.57087397835721,1.,-1.31558903860015));
#33184=CARTESIAN_POINT('Ctrl Pts',(1.56496872402352,-1.,-1.31381795281002));
#33185=CARTESIAN_POINT('Ctrl Pts',(1.56496872402352,1.,-1.31381795281002));
#33186=CARTESIAN_POINT('Ctrl Pts',(1.55908521254822,-1.,-1.31200264341696));
#33187=CARTESIAN_POINT('Ctrl Pts',(1.55908521254822,1.,-1.31200264341696));
#33188=CARTESIAN_POINT('Ctrl Pts',(1.55322568759481,-1.,-1.31014393684221));
#33189=CARTESIAN_POINT('Ctrl Pts',(1.55322568759481,1.,-1.31014393684221));
#33190=CARTESIAN_POINT('Ctrl Pts',(1.54739413957183,-1.,-1.30824393907471));
#33191=CARTESIAN_POINT('Ctrl Pts',(1.54739413957183,1.,-1.30824393907471));
#33192=CARTESIAN_POINT('Ctrl Pts',(1.54159462645428,-1.,-1.30630475189553));
#33193=CARTESIAN_POINT('Ctrl Pts',(1.54159462645428,1.,-1.30630475189553));
#33194=CARTESIAN_POINT('Ctrl Pts',(1.53582981268976,-1.,-1.30432735639487));
#33195=CARTESIAN_POINT('Ctrl Pts',(1.53582981268976,1.,-1.30432735639487));
#33196=CARTESIAN_POINT('Ctrl Pts',(1.53009970283893,-1.,-1.3023106439557));
#33197=CARTESIAN_POINT('Ctrl Pts',(1.53009970283893,1.,-1.3023106439557));
#33198=CARTESIAN_POINT('Ctrl Pts',(1.5243995786107,-1.,-1.30024984366334));
#33199=CARTESIAN_POINT('Ctrl Pts',(1.5243995786107,1.,-1.30024984366334));
#33200=CARTESIAN_POINT('Ctrl Pts',(1.51872184912735,-1.,-1.29813791800757));
#33201=CARTESIAN_POINT('Ctrl Pts',(1.51872184912735,1.,-1.29813791800757));
#33202=CARTESIAN_POINT('Ctrl Pts',(1.51305994241412,-1.,-1.29596850710518));
#33203=CARTESIAN_POINT('Ctrl Pts',(1.51305994241412,1.,-1.29596850710518));
#33204=CARTESIAN_POINT('Ctrl Pts',(1.50741159078367,-1.,-1.29373841372843));
#33205=CARTESIAN_POINT('Ctrl Pts',(1.50741159078367,1.,-1.29373841372843));
#33206=CARTESIAN_POINT('Ctrl Pts',(1.50178230149764,-1.,-1.29145022885171));
#33207=CARTESIAN_POINT('Ctrl Pts',(1.50178230149764,1.,-1.29145022885171));
#33208=CARTESIAN_POINT('Ctrl Pts',(1.49618896881729,-1.,-1.28911506584232));
#33209=CARTESIAN_POINT('Ctrl Pts',(1.49618896881729,1.,-1.28911506584232));
#33210=CARTESIAN_POINT('Ctrl Pts',(1.4906522831275,-1.,-1.28674676116415));
#33211=CARTESIAN_POINT('Ctrl Pts',(1.4906522831275,1.,-1.28674676116415));
#33212=CARTESIAN_POINT('Ctrl Pts',(1.48518817118891,-1.,-1.28435533880184));
#33213=CARTESIAN_POINT('Ctrl Pts',(1.48518817118891,1.,-1.28435533880184));
#33214=CARTESIAN_POINT('Ctrl Pts',(1.47980070347102,-1.,-1.28194158939522));
#33215=CARTESIAN_POINT('Ctrl Pts',(1.47980070347102,1.,-1.28194158939522));
#33216=CARTESIAN_POINT('Ctrl Pts',(1.4744717526711,-1.,-1.27948918248524));
#33217=CARTESIAN_POINT('Ctrl Pts',(1.4744717526711,1.,-1.27948918248524));
#33218=CARTESIAN_POINT('Ctrl Pts',(1.46916035917197,-1.,-1.27696414831144));
#33219=CARTESIAN_POINT('Ctrl Pts',(1.46916035917197,1.,-1.27696414831144));
#33220=CARTESIAN_POINT('Ctrl Pts',(1.4638243133254,-1.,-1.27433119897877));
#33221=CARTESIAN_POINT('Ctrl Pts',(1.4638243133254,1.,-1.27433119897877));
#33222=CARTESIAN_POINT('Ctrl Pts',(1.45843906294725,-1.,-1.27156805265312));
#33223=CARTESIAN_POINT('Ctrl Pts',(1.45843906294725,1.,-1.27156805265312));
#33224=CARTESIAN_POINT('Ctrl Pts',(1.45301422764205,-1.,-1.26867786804854));
#33225=CARTESIAN_POINT('Ctrl Pts',(1.45301422764205,1.,-1.26867786804854));
#33226=CARTESIAN_POINT('Ctrl Pts',(1.44761985001544,-1.,-1.26570925118767));
#33227=CARTESIAN_POINT('Ctrl Pts',(1.44761985001544,1.,-1.26570925118767));
#33228=CARTESIAN_POINT('Ctrl Pts',(1.44236470511145,-1.,-1.26273903323723));
#33229=CARTESIAN_POINT('Ctrl Pts',(1.44236470511145,1.,-1.26273903323723));
#33230=CARTESIAN_POINT('Ctrl Pts',(1.43734919180719,-1.,-1.25983531011894));
#33231=CARTESIAN_POINT('Ctrl Pts',(1.43734919180719,1.,-1.25983531011894));
#33232=CARTESIAN_POINT('Ctrl Pts',(1.43262645609679,-1.,-1.25702687965744));
#33233=CARTESIAN_POINT('Ctrl Pts',(1.43262645609679,1.,-1.25702687965744));
#33234=CARTESIAN_POINT('Ctrl Pts',(1.42815938799555,-1.,-1.25426945222783));
#33235=CARTESIAN_POINT('Ctrl Pts',(1.42815938799555,1.,-1.25426945222783));
#33236=CARTESIAN_POINT('Ctrl Pts',(1.42378102115911,-1.,-1.25141455570299));
#33237=CARTESIAN_POINT('Ctrl Pts',(1.42378102115911,1.,-1.25141455570299));
#33238=CARTESIAN_POINT('Ctrl Pts',(1.41923722596421,-1.,-1.24824430986911));
#33239=CARTESIAN_POINT('Ctrl Pts',(1.41923722596421,1.,-1.24824430986911));
#33240=CARTESIAN_POINT('Ctrl Pts',(1.41422913175437,-1.,-1.24450600513278));
#33241=CARTESIAN_POINT('Ctrl Pts',(1.41422913175437,1.,-1.24450600513278));
#33242=CARTESIAN_POINT('Ctrl Pts',(1.40845295531151,-1.,-1.23994455029421));
#33243=CARTESIAN_POINT('Ctrl Pts',(1.40845295531151,1.,-1.23994455029421));
#33244=CARTESIAN_POINT('Ctrl Pts',(1.40164708205345,-1.,-1.23434087289768));
#33245=CARTESIAN_POINT('Ctrl Pts',(1.40164708205345,1.,-1.23434087289768));
#33246=CARTESIAN_POINT('Ctrl Pts',(1.39361389567257,-1.,-1.22752961898063));
#33247=CARTESIAN_POINT('Ctrl Pts',(1.39361389567257,1.,-1.22752961898063));
#33248=CARTESIAN_POINT('Ctrl Pts',(1.38420564525391,-1.,-1.21938737278853));
#33249=CARTESIAN_POINT('Ctrl Pts',(1.38420564525391,1.,-1.21938737278853));
#33250=CARTESIAN_POINT('Ctrl Pts',(1.37331915604962,-1.,-1.20982812923113));
#33251=CARTESIAN_POINT('Ctrl Pts',(1.37331915604962,1.,-1.20982812923113));
#33252=CARTESIAN_POINT('Ctrl Pts',(1.36088705040677,-1.,-1.1987959077656));
#33253=CARTESIAN_POINT('Ctrl Pts',(1.36088705040677,1.,-1.1987959077656));
#33254=CARTESIAN_POINT('Ctrl Pts',(1.34687053998157,-1.,-1.18625865664915));
#33255=CARTESIAN_POINT('Ctrl Pts',(1.34687053998157,1.,-1.18625865664915));
#33256=CARTESIAN_POINT('Ctrl Pts',(1.33437539344842,-1.,-1.17501305787994));
#33257=CARTESIAN_POINT('Ctrl Pts',(1.33437539344842,1.,-1.17501305787994));
#33258=CARTESIAN_POINT('Ctrl Pts',(1.32428080720544,-1.,-1.16589330092532));
#33259=CARTESIAN_POINT('Ctrl Pts',(1.32428080720544,1.,-1.16589330092532));
#33260=CARTESIAN_POINT('Ctrl Pts',(1.3172297721596,-1.,-1.15950888730433));
#33261=CARTESIAN_POINT('Ctrl Pts',(1.3172297721596,1.,-1.15950888730433));
#33262=CARTESIAN_POINT('Ctrl Pts',(1.31362392696032,-1.,-1.15624053661742));
#33263=CARTESIAN_POINT('Ctrl Pts',(1.31362392696032,1.,-1.15624053661742));
#33264=CARTESIAN_POINT('',(1.73811241238545,1.,-1.34869019493419));
#33265=CARTESIAN_POINT('Ctrl Pts',(1.73811241238545,1.,-1.34869019493419));
#33266=CARTESIAN_POINT('Ctrl Pts',(1.73682580585819,1.,-1.34854391898145));
#33267=CARTESIAN_POINT('Ctrl Pts',(1.73425417886254,1.,-1.34824783113158));
#33268=CARTESIAN_POINT('Ctrl Pts',(1.73040149654497,1.,-1.3477930915247));
#33269=CARTESIAN_POINT('Ctrl Pts',(1.72527410681298,1.,-1.34716554820013));
#33270=CARTESIAN_POINT('Ctrl Pts',(1.7188807715095,1.,-1.34634568653586));
#33271=CARTESIAN_POINT('Ctrl Pts',(1.71250340687011,1.,-1.34549029589563));
#33272=CARTESIAN_POINT('Ctrl Pts',(1.70614212266676,1.,-1.34459924533783));
#33273=CARTESIAN_POINT('Ctrl Pts',(1.69979707754221,1.,-1.34367237124322));
#33274=CARTESIAN_POINT('Ctrl Pts',(1.6934684849664,1.,-1.34270948206139));
#33275=CARTESIAN_POINT('Ctrl Pts',(1.68715660868602,1.,-1.34171037484673));
#33276=CARTESIAN_POINT('Ctrl Pts',(1.68086176030308,1.,-1.3406748518516));
#33277=CARTESIAN_POINT('Ctrl Pts',(1.67458429426126,1.,-1.33960273470372));
#33278=CARTESIAN_POINT('Ctrl Pts',(1.66832460784078,1.,-1.33849388654458));
#33279=CARTESIAN_POINT('Ctrl Pts',(1.66208312542073,1.,-1.33734820885331));
#33280=CARTESIAN_POINT('Ctrl Pts',(1.65586025952651,1.,-1.33616559745217));
#33281=CARTESIAN_POINT('Ctrl Pts',(1.64965637286843,1.,-1.33494590468003));
#33282=CARTESIAN_POINT('Ctrl Pts',(1.64347174856007,1.,-1.33368890676554));
#33283=CARTESIAN_POINT('Ctrl Pts',(1.63730653475049,1.,-1.33239425103694));
#33284=CARTESIAN_POINT('Ctrl Pts',(1.63116079730887,1.,-1.33106149345618));
#33285=CARTESIAN_POINT('Ctrl Pts',(1.62503464209777,1.,-1.32969019505665));
#33286=CARTESIAN_POINT('Ctrl Pts',(1.61892832270723,1.,-1.32828000610448));
#33287=CARTESIAN_POINT('Ctrl Pts',(1.61284234015762,1.,-1.32683074483365));
#33288=CARTESIAN_POINT('Ctrl Pts',(1.6067775829097,1.,-1.32534250785794));
#33289=CARTESIAN_POINT('Ctrl Pts',(1.600735118587,1.,-1.32381550858266));
#33290=CARTESIAN_POINT('Ctrl Pts',(1.59471591079408,1.,-1.32224985747686));
#33291=CARTESIAN_POINT('Ctrl Pts',(1.58872057258244,1.,-1.32064537110891));
#33292=CARTESIAN_POINT('Ctrl Pts',(1.58274907898829,1.,-1.31900135021428));
#33293=CARTESIAN_POINT('Ctrl Pts',(1.57680056505585,1.,-1.31731642317183));
#33294=CARTESIAN_POINT('Ctrl Pts',(1.57087397835721,1.,-1.31558903860015));
#33295=CARTESIAN_POINT('Ctrl Pts',(1.56496872402352,1.,-1.31381795281002));
#33296=CARTESIAN_POINT('Ctrl Pts',(1.55908521254822,1.,-1.31200264341696));
#33297=CARTESIAN_POINT('Ctrl Pts',(1.55322568759481,1.,-1.31014393684221));
#33298=CARTESIAN_POINT('Ctrl Pts',(1.54739413957183,1.,-1.30824393907471));
#33299=CARTESIAN_POINT('Ctrl Pts',(1.54159462645428,1.,-1.30630475189553));
#33300=CARTESIAN_POINT('Ctrl Pts',(1.53582981268976,1.,-1.30432735639487));
#33301=CARTESIAN_POINT('Ctrl Pts',(1.53009970283893,1.,-1.3023106439557));
#33302=CARTESIAN_POINT('Ctrl Pts',(1.5243995786107,1.,-1.30024984366334));
#33303=CARTESIAN_POINT('Ctrl Pts',(1.51872184912735,1.,-1.29813791800757));
#33304=CARTESIAN_POINT('Ctrl Pts',(1.51305994241412,1.,-1.29596850710518));
#33305=CARTESIAN_POINT('Ctrl Pts',(1.50741159078367,1.,-1.29373841372843));
#33306=CARTESIAN_POINT('Ctrl Pts',(1.50178230149764,1.,-1.29145022885171));
#33307=CARTESIAN_POINT('Ctrl Pts',(1.49618896881729,1.,-1.28911506584232));
#33308=CARTESIAN_POINT('Ctrl Pts',(1.4906522831275,1.,-1.28674676116415));
#33309=CARTESIAN_POINT('Ctrl Pts',(1.48518817118891,1.,-1.28435533880184));
#33310=CARTESIAN_POINT('Ctrl Pts',(1.47980070347102,1.,-1.28194158939522));
#33311=CARTESIAN_POINT('Ctrl Pts',(1.4744717526711,1.,-1.27948918248524));
#33312=CARTESIAN_POINT('Ctrl Pts',(1.46916035917197,1.,-1.27696414831144));
#33313=CARTESIAN_POINT('Ctrl Pts',(1.4638243133254,1.,-1.27433119897877));
#33314=CARTESIAN_POINT('Ctrl Pts',(1.45843906294725,1.,-1.27156805265312));
#33315=CARTESIAN_POINT('Ctrl Pts',(1.45301422764205,1.,-1.26867786804854));
#33316=CARTESIAN_POINT('Ctrl Pts',(1.44761985001544,1.,-1.26570925118767));
#33317=CARTESIAN_POINT('Ctrl Pts',(1.44236470511145,1.,-1.26273903323723));
#33318=CARTESIAN_POINT('Ctrl Pts',(1.43734919180719,1.,-1.25983531011894));
#33319=CARTESIAN_POINT('Ctrl Pts',(1.43262645609679,1.,-1.25702687965744));
#33320=CARTESIAN_POINT('Ctrl Pts',(1.42815938799555,1.,-1.25426945222783));
#33321=CARTESIAN_POINT('Ctrl Pts',(1.42378102115911,1.,-1.25141455570299));
#33322=CARTESIAN_POINT('Ctrl Pts',(1.41923722596421,1.,-1.24824430986911));
#33323=CARTESIAN_POINT('Ctrl Pts',(1.41422913175437,1.,-1.24450600513278));
#33324=CARTESIAN_POINT('Ctrl Pts',(1.40845295531151,1.,-1.23994455029421));
#33325=CARTESIAN_POINT('Ctrl Pts',(1.40164708205345,1.,-1.23434087289768));
#33326=CARTESIAN_POINT('Ctrl Pts',(1.39361389567257,1.,-1.22752961898063));
#33327=CARTESIAN_POINT('Ctrl Pts',(1.38420564525391,1.,-1.21938737278853));
#33328=CARTESIAN_POINT('Ctrl Pts',(1.37331915604962,1.,-1.20982812923113));
#33329=CARTESIAN_POINT('Ctrl Pts',(1.36088705040677,1.,-1.1987959077656));
#33330=CARTESIAN_POINT('Ctrl Pts',(1.34687053998157,1.,-1.18625865664915));
#33331=CARTESIAN_POINT('Ctrl Pts',(1.33437539344842,1.,-1.17501305787994));
#33332=CARTESIAN_POINT('Ctrl Pts',(1.32428080720544,1.,-1.16589330092532));
#33333=CARTESIAN_POINT('Ctrl Pts',(1.3172297721596,1.,-1.15950888730433));
#33334=CARTESIAN_POINT('Ctrl Pts',(1.31362392696032,1.,-1.15624053661742));
#33335=CARTESIAN_POINT('',(1.73811241238545,0.,-1.34869019493419));
#33336=CARTESIAN_POINT('Origin',(1.81978687191668,0.,-1.23627494547115));
#33337=CARTESIAN_POINT('',(1.81978687191668,1.,-1.23627494547115));
#33338=CARTESIAN_POINT('',(1.73811241238545,1.,-1.34869019493419));
#33339=CARTESIAN_POINT('',(1.81978687191668,0.,-1.23627494547115));
#33340=CARTESIAN_POINT('Ctrl Pts',(1.5055822144029,-1.,-0.892032620296855));
#33341=CARTESIAN_POINT('Ctrl Pts',(1.5055822144029,1.,-0.892032620296855));
#33342=CARTESIAN_POINT('Ctrl Pts',(1.50980486807181,-1.,-0.894452006967538));
#33343=CARTESIAN_POINT('Ctrl Pts',(1.50980486807181,1.,-0.894452006967538));
#33344=CARTESIAN_POINT('Ctrl Pts',(1.51805569591479,-1.,-0.89918504749193));
#33345=CARTESIAN_POINT('Ctrl Pts',(1.51805569591479,1.,-0.89918504749193));
#33346=CARTESIAN_POINT('Ctrl Pts',(1.52984849890434,-1.,-0.905967409640499));
#33347=CARTESIAN_POINT('Ctrl Pts',(1.52984849890434,1.,-0.905967409640499));
#33348=CARTESIAN_POINT('Ctrl Pts',(1.54440491152807,-1.,-0.91437591904658));
#33349=CARTESIAN_POINT('Ctrl Pts',(1.54440491152807,1.,-0.91437591904658));
#33350=CARTESIAN_POINT('Ctrl Pts',(1.56065988582509,-1.,-0.923832188966322));
#33351=CARTESIAN_POINT('Ctrl Pts',(1.56065988582509,1.,-0.923832188966322));
#33352=CARTESIAN_POINT('Ctrl Pts',(1.57499388385561,-1.,-0.932246680128849));
#33353=CARTESIAN_POINT('Ctrl Pts',(1.57499388385561,1.,-0.932246680128849));
#33354=CARTESIAN_POINT('Ctrl Pts',(1.58744937489796,-1.,-0.939646377909319));
#33355=CARTESIAN_POINT('Ctrl Pts',(1.58744937489796,1.,-0.939646377909319));
#33356=CARTESIAN_POINT('Ctrl Pts',(1.59810042045408,-1.,-0.946078063325796));
#33357=CARTESIAN_POINT('Ctrl Pts',(1.59810042045408,1.,-0.946078063325796));
#33358=CARTESIAN_POINT('Ctrl Pts',(1.60706069897794,-1.,-0.951613284361248));
#33359=CARTESIAN_POINT('Ctrl Pts',(1.60706069897794,1.,-0.951613284361248));
#33360=CARTESIAN_POINT('Ctrl Pts',(1.61449324337233,-1.,-0.956354422921573));
#33361=CARTESIAN_POINT('Ctrl Pts',(1.61449324337233,1.,-0.956354422921573));
#33362=CARTESIAN_POINT('Ctrl Pts',(1.62061638139929,-1.,-0.960438326099958));
#33363=CARTESIAN_POINT('Ctrl Pts',(1.62061638139929,1.,-0.960438326099958));
#33364=CARTESIAN_POINT('Ctrl Pts',(1.6257193066974,-1.,-0.964046107037821));
#33365=CARTESIAN_POINT('Ctrl Pts',(1.6257193066974,1.,-0.964046107037821));
#33366=CARTESIAN_POINT('Ctrl Pts',(1.63013849959083,-1.,-0.967387853228041));
#33367=CARTESIAN_POINT('Ctrl Pts',(1.63013849959083,1.,-0.967387853228041));
#33368=CARTESIAN_POINT('Ctrl Pts',(1.63420665729609,-1.,-0.970669715996356));
#33369=CARTESIAN_POINT('Ctrl Pts',(1.63420665729609,1.,-0.970669715996356));
#33370=CARTESIAN_POINT('Ctrl Pts',(1.63820952658157,-1.,-0.974066058287501));
#33371=CARTESIAN_POINT('Ctrl Pts',(1.63820952658157,1.,-0.974066058287501));
#33372=CARTESIAN_POINT('Ctrl Pts',(1.64233990826831,-1.,-0.977689794120297));
#33373=CARTESIAN_POINT('Ctrl Pts',(1.64233990826831,1.,-0.977689794120297));
#33374=CARTESIAN_POINT('Ctrl Pts',(1.64665139190834,-1.,-0.981562530940574));
#33375=CARTESIAN_POINT('Ctrl Pts',(1.64665139190834,1.,-0.981562530940574));
#33376=CARTESIAN_POINT('Ctrl Pts',(1.6511001661277,-1.,-0.985642622921626));
#33377=CARTESIAN_POINT('Ctrl Pts',(1.6511001661277,1.,-0.985642622921626));
#33378=CARTESIAN_POINT('Ctrl Pts',(1.65559044289746,-1.,-0.98985562785445));
#33379=CARTESIAN_POINT('Ctrl Pts',(1.65559044289746,1.,-0.98985562785445));
#33380=CARTESIAN_POINT('Ctrl Pts',(1.66001553809916,-1.,-0.994121836661116));
#33381=CARTESIAN_POINT('Ctrl Pts',(1.66001553809916,1.,-0.994121836661116));
#33382=CARTESIAN_POINT('Ctrl Pts',(1.66430758030304,-1.,-0.998389654952317));
#33383=CARTESIAN_POINT('Ctrl Pts',(1.66430758030304,1.,-0.998389654952317));
#33384=CARTESIAN_POINT('Ctrl Pts',(1.66846059277231,-1.,-1.00265091003682));
#33385=CARTESIAN_POINT('Ctrl Pts',(1.66846059277231,1.,-1.00265091003682));
#33386=CARTESIAN_POINT('Ctrl Pts',(1.67250335383248,-1.,-1.00692206696387));
#33387=CARTESIAN_POINT('Ctrl Pts',(1.67250335383248,1.,-1.00692206696387));
#33388=CARTESIAN_POINT('Ctrl Pts',(1.67648246776457,-1.,-1.01123236493507));
#33389=CARTESIAN_POINT('Ctrl Pts',(1.67648246776457,1.,-1.01123236493507));
#33390=CARTESIAN_POINT('Ctrl Pts',(1.6804428989482,-1.,-1.01561026162787));
#33391=CARTESIAN_POINT('Ctrl Pts',(1.6804428989482,1.,-1.01561026162787));
#33392=CARTESIAN_POINT('Ctrl Pts',(1.68440578021739,-1.,-1.02006795074222));
#33393=CARTESIAN_POINT('Ctrl Pts',(1.68440578021739,1.,-1.02006795074222));
#33394=CARTESIAN_POINT('Ctrl Pts',(1.68836910178475,-1.,-1.02460180535272));
#33395=CARTESIAN_POINT('Ctrl Pts',(1.68836910178475,1.,-1.02460180535272));
#33396=CARTESIAN_POINT('Ctrl Pts',(1.69231840863471,-1.,-1.02919977579155));
#33397=CARTESIAN_POINT('Ctrl Pts',(1.69231840863471,1.,-1.02919977579155));
#33398=CARTESIAN_POINT('Ctrl Pts',(1.69623414782769,-1.,-1.03384646003587));
#33399=CARTESIAN_POINT('Ctrl Pts',(1.69623414782769,1.,-1.03384646003587));
#33400=CARTESIAN_POINT('Ctrl Pts',(1.70010052930951,-1.,-1.03852922490782));
#33401=CARTESIAN_POINT('Ctrl Pts',(1.70010052930951,1.,-1.03852922490782));
#33402=CARTESIAN_POINT('Ctrl Pts',(1.70391338707969,-1.,-1.04324363334546));
#33403=CARTESIAN_POINT('Ctrl Pts',(1.70391338707969,1.,-1.04324363334546));
#33404=CARTESIAN_POINT('Ctrl Pts',(1.70767646263641,-1.,-1.0479908540499));
#33405=CARTESIAN_POINT('Ctrl Pts',(1.70767646263641,1.,-1.0479908540499));
#33406=CARTESIAN_POINT('Ctrl Pts',(1.71139783543986,-1.,-1.05277517202854));
#33407=CARTESIAN_POINT('Ctrl Pts',(1.71139783543986,1.,-1.05277517202854));
#33408=CARTESIAN_POINT('Ctrl Pts',(1.71508654427022,-1.,-1.05760163192481));
#33409=CARTESIAN_POINT('Ctrl Pts',(1.71508654427022,1.,-1.05760163192481));
#33410=CARTESIAN_POINT('Ctrl Pts',(1.71874858456908,-1.,-1.0624732468065));
#33411=CARTESIAN_POINT('Ctrl Pts',(1.71874858456908,1.,-1.0624732468065));
#33412=CARTESIAN_POINT('Ctrl Pts',(1.72238500928456,-1.,-1.06738966975463));
#33413=CARTESIAN_POINT('Ctrl Pts',(1.72238500928456,1.,-1.06738966975463));
#33414=CARTESIAN_POINT('Ctrl Pts',(1.72599406198489,-1.,-1.07234866990252));
#33415=CARTESIAN_POINT('Ctrl Pts',(1.72599406198489,1.,-1.07234866990252));
#33416=CARTESIAN_POINT('Ctrl Pts',(1.72957248977424,-1.,-1.0773470373727));
#33417=CARTESIAN_POINT('Ctrl Pts',(1.72957248977424,1.,-1.0773470373727));
#33418=CARTESIAN_POINT('Ctrl Pts',(1.73311705663407,-1.,-1.08238162784749));
#33419=CARTESIAN_POINT('Ctrl Pts',(1.73311705663407,1.,-1.08238162784749));
#33420=CARTESIAN_POINT('Ctrl Pts',(1.73662628326093,-1.,-1.08745056285429));
#33421=CARTESIAN_POINT('Ctrl Pts',(1.73662628326093,1.,-1.08745056285429));
#33422=CARTESIAN_POINT('Ctrl Pts',(1.74010053962252,-1.,-1.09255329056496));
#33423=CARTESIAN_POINT('Ctrl Pts',(1.74010053962252,1.,-1.09255329056496));
#33424=CARTESIAN_POINT('Ctrl Pts',(1.74354119236212,-1.,-1.09768999241229));
#33425=CARTESIAN_POINT('Ctrl Pts',(1.74354119236212,1.,-1.09768999241229));
#33426=CARTESIAN_POINT('Ctrl Pts',(1.74695004214924,-1.,-1.10286118991144));
#33427=CARTESIAN_POINT('Ctrl Pts',(1.74695004214924,1.,-1.10286118991144));
#33428=CARTESIAN_POINT('Ctrl Pts',(1.75032866075914,-1.,-1.10806728183003));
#33429=CARTESIAN_POINT('Ctrl Pts',(1.75032866075914,1.,-1.10806728183003));
#33430=CARTESIAN_POINT('Ctrl Pts',(1.75367772094617,-1.,-1.11330807582542));
#33431=CARTESIAN_POINT('Ctrl Pts',(1.75367772094617,1.,-1.11330807582542));
#33432=CARTESIAN_POINT('Ctrl Pts',(1.75699720772089,-1.,-1.11858293216752));
#33433=CARTESIAN_POINT('Ctrl Pts',(1.75699720772089,1.,-1.11858293216752));
#33434=CARTESIAN_POINT('Ctrl Pts',(1.76028671825084,-1.,-1.12389096855078));
#33435=CARTESIAN_POINT('Ctrl Pts',(1.76028671825084,1.,-1.12389096855078));
#33436=CARTESIAN_POINT('Ctrl Pts',(1.76354571966171,-1.,-1.12923123555076));
#33437=CARTESIAN_POINT('Ctrl Pts',(1.76354571966171,1.,-1.12923123555076));
#33438=CARTESIAN_POINT('Ctrl Pts',(1.76677384551883,-1.,-1.13460291804635));
#33439=CARTESIAN_POINT('Ctrl Pts',(1.76677384551883,1.,-1.13460291804635));
#33440=CARTESIAN_POINT('Ctrl Pts',(1.76997111386806,-1.,-1.14000548337));
#33441=CARTESIAN_POINT('Ctrl Pts',(1.76997111386806,1.,-1.14000548337));
#33442=CARTESIAN_POINT('Ctrl Pts',(1.77313777896234,-1.,-1.14543858226948));
#33443=CARTESIAN_POINT('Ctrl Pts',(1.77313777896234,1.,-1.14543858226948));
#33444=CARTESIAN_POINT('Ctrl Pts',(1.77627422557034,-1.,-1.15090197841531));
#33445=CARTESIAN_POINT('Ctrl Pts',(1.77627422557034,1.,-1.15090197841531));
#33446=CARTESIAN_POINT('Ctrl Pts',(1.77938085564261,-1.,-1.15639547194689));
#33447=CARTESIAN_POINT('Ctrl Pts',(1.77938085564261,1.,-1.15639547194689));
#33448=CARTESIAN_POINT('Ctrl Pts',(1.78245795880949,-1.,-1.16191881298458));
#33449=CARTESIAN_POINT('Ctrl Pts',(1.78245795880949,1.,-1.16191881298458));
#33450=CARTESIAN_POINT('Ctrl Pts',(1.78550566040349,-1.,-1.16747166312239));
#33451=CARTESIAN_POINT('Ctrl Pts',(1.78550566040349,1.,-1.16747166312239));
#33452=CARTESIAN_POINT('Ctrl Pts',(1.78852398877523,-1.,-1.17305363177265));
#33453=CARTESIAN_POINT('Ctrl Pts',(1.78852398877523,1.,-1.17305363177265));
#33454=CARTESIAN_POINT('Ctrl Pts',(1.79151291552646,-1.,-1.17866429440781));
#33455=CARTESIAN_POINT('Ctrl Pts',(1.79151291552646,1.,-1.17866429440781));
#33456=CARTESIAN_POINT('Ctrl Pts',(1.79447240321572,-1.,-1.18430321697471));
#33457=CARTESIAN_POINT('Ctrl Pts',(1.79447240321572,1.,-1.18430321697471));
#33458=CARTESIAN_POINT('Ctrl Pts',(1.79740245923649,-1.,-1.1899699793456));
#33459=CARTESIAN_POINT('Ctrl Pts',(1.79740245923649,1.,-1.1899699793456));
#33460=CARTESIAN_POINT('Ctrl Pts',(1.80030314370121,-1.,-1.19566418930405));
#33461=CARTESIAN_POINT('Ctrl Pts',(1.80030314370121,1.,-1.19566418930405));
#33462=CARTESIAN_POINT('Ctrl Pts',(1.8031745483882,-1.,-1.2013854893912));
#33463=CARTESIAN_POINT('Ctrl Pts',(1.8031745483882,1.,-1.2013854893912));
#33464=CARTESIAN_POINT('Ctrl Pts',(1.80601678480772,-1.,-1.20713356605519));
#33465=CARTESIAN_POINT('Ctrl Pts',(1.80601678480772,1.,-1.20713356605519));
#33466=CARTESIAN_POINT('Ctrl Pts',(1.80882996916931,-1.,-1.2129081570818));
#33467=CARTESIAN_POINT('Ctrl Pts',(1.80882996916931,1.,-1.2129081570818));
#33468=CARTESIAN_POINT('Ctrl Pts',(1.81161420806172,-1.,-1.2187090610323));
#33469=CARTESIAN_POINT('Ctrl Pts',(1.81161420806172,1.,-1.2187090610323));
#33470=CARTESIAN_POINT('Ctrl Pts',(1.81436959209778,-1.,-1.22453613304507));
#33471=CARTESIAN_POINT('Ctrl Pts',(1.81436959209778,1.,-1.22453613304507));
#33472=CARTESIAN_POINT('Ctrl Pts',(1.81655087183054,-1.,-1.22921864890975));
#33473=CARTESIAN_POINT('Ctrl Pts',(1.81655087183054,1.,-1.22921864890975));
#33474=CARTESIAN_POINT('Ctrl Pts',(1.81817389920914,-1.,-1.23274224526804));
#33475=CARTESIAN_POINT('Ctrl Pts',(1.81817389920914,1.,-1.23274224526804));
#33476=CARTESIAN_POINT('Ctrl Pts',(1.81925017193531,-1.,-1.23509651170384));
#33477=CARTESIAN_POINT('Ctrl Pts',(1.81925017193531,1.,-1.23509651170384));
#33478=CARTESIAN_POINT('Ctrl Pts',(1.81978687191668,-1.,-1.23627494547115));
#33479=CARTESIAN_POINT('Ctrl Pts',(1.81978687191668,1.,-1.23627494547115));
#33480=CARTESIAN_POINT('',(1.5055822144029,1.,-0.892032620296855));
#33481=CARTESIAN_POINT('Ctrl Pts',(1.5055822144029,1.,-0.892032620296855));
#33482=CARTESIAN_POINT('Ctrl Pts',(1.50980486807181,1.,-0.894452006967538));
#33483=CARTESIAN_POINT('Ctrl Pts',(1.51805569591479,1.,-0.89918504749193));
#33484=CARTESIAN_POINT('Ctrl Pts',(1.52984849890434,1.,-0.905967409640499));
#33485=CARTESIAN_POINT('Ctrl Pts',(1.54440491152807,1.,-0.91437591904658));
#33486=CARTESIAN_POINT('Ctrl Pts',(1.56065988582509,1.,-0.923832188966322));
#33487=CARTESIAN_POINT('Ctrl Pts',(1.57499388385561,1.,-0.932246680128849));
#33488=CARTESIAN_POINT('Ctrl Pts',(1.58744937489796,1.,-0.939646377909319));
#33489=CARTESIAN_POINT('Ctrl Pts',(1.59810042045408,1.,-0.946078063325796));
#33490=CARTESIAN_POINT('Ctrl Pts',(1.60706069897794,1.,-0.951613284361248));
#33491=CARTESIAN_POINT('Ctrl Pts',(1.61449324337233,1.,-0.956354422921573));
#33492=CARTESIAN_POINT('Ctrl Pts',(1.62061638139929,1.,-0.960438326099958));
#33493=CARTESIAN_POINT('Ctrl Pts',(1.6257193066974,1.,-0.964046107037821));
#33494=CARTESIAN_POINT('Ctrl Pts',(1.63013849959083,1.,-0.967387853228041));
#33495=CARTESIAN_POINT('Ctrl Pts',(1.63420665729609,1.,-0.970669715996356));
#33496=CARTESIAN_POINT('Ctrl Pts',(1.63820952658157,1.,-0.974066058287501));
#33497=CARTESIAN_POINT('Ctrl Pts',(1.64233990826831,1.,-0.977689794120297));
#33498=CARTESIAN_POINT('Ctrl Pts',(1.64665139190834,1.,-0.981562530940574));
#33499=CARTESIAN_POINT('Ctrl Pts',(1.6511001661277,1.,-0.985642622921626));
#33500=CARTESIAN_POINT('Ctrl Pts',(1.65559044289746,1.,-0.98985562785445));
#33501=CARTESIAN_POINT('Ctrl Pts',(1.66001553809916,1.,-0.994121836661116));
#33502=CARTESIAN_POINT('Ctrl Pts',(1.66430758030304,1.,-0.998389654952317));
#33503=CARTESIAN_POINT('Ctrl Pts',(1.66846059277231,1.,-1.00265091003682));
#33504=CARTESIAN_POINT('Ctrl Pts',(1.67250335383248,1.,-1.00692206696387));
#33505=CARTESIAN_POINT('Ctrl Pts',(1.67648246776457,1.,-1.01123236493507));
#33506=CARTESIAN_POINT('Ctrl Pts',(1.6804428989482,1.,-1.01561026162787));
#33507=CARTESIAN_POINT('Ctrl Pts',(1.68440578021739,1.,-1.02006795074222));
#33508=CARTESIAN_POINT('Ctrl Pts',(1.68836910178475,1.,-1.02460180535272));
#33509=CARTESIAN_POINT('Ctrl Pts',(1.69231840863471,1.,-1.02919977579155));
#33510=CARTESIAN_POINT('Ctrl Pts',(1.69623414782769,1.,-1.03384646003587));
#33511=CARTESIAN_POINT('Ctrl Pts',(1.70010052930951,1.,-1.03852922490782));
#33512=CARTESIAN_POINT('Ctrl Pts',(1.70391338707969,1.,-1.04324363334546));
#33513=CARTESIAN_POINT('Ctrl Pts',(1.70767646263641,1.,-1.0479908540499));
#33514=CARTESIAN_POINT('Ctrl Pts',(1.71139783543986,1.,-1.05277517202854));
#33515=CARTESIAN_POINT('Ctrl Pts',(1.71508654427022,1.,-1.05760163192481));
#33516=CARTESIAN_POINT('Ctrl Pts',(1.71874858456908,1.,-1.0624732468065));
#33517=CARTESIAN_POINT('Ctrl Pts',(1.72238500928456,1.,-1.06738966975463));
#33518=CARTESIAN_POINT('Ctrl Pts',(1.72599406198489,1.,-1.07234866990252));
#33519=CARTESIAN_POINT('Ctrl Pts',(1.72957248977424,1.,-1.0773470373727));
#33520=CARTESIAN_POINT('Ctrl Pts',(1.73311705663407,1.,-1.08238162784749));
#33521=CARTESIAN_POINT('Ctrl Pts',(1.73662628326093,1.,-1.08745056285429));
#33522=CARTESIAN_POINT('Ctrl Pts',(1.74010053962252,1.,-1.09255329056496));
#33523=CARTESIAN_POINT('Ctrl Pts',(1.74354119236212,1.,-1.09768999241229));
#33524=CARTESIAN_POINT('Ctrl Pts',(1.74695004214924,1.,-1.10286118991144));
#33525=CARTESIAN_POINT('Ctrl Pts',(1.75032866075914,1.,-1.10806728183003));
#33526=CARTESIAN_POINT('Ctrl Pts',(1.75367772094617,1.,-1.11330807582542));
#33527=CARTESIAN_POINT('Ctrl Pts',(1.75699720772089,1.,-1.11858293216752));
#33528=CARTESIAN_POINT('Ctrl Pts',(1.76028671825084,1.,-1.12389096855078));
#33529=CARTESIAN_POINT('Ctrl Pts',(1.76354571966171,1.,-1.12923123555076));
#33530=CARTESIAN_POINT('Ctrl Pts',(1.76677384551883,1.,-1.13460291804635));
#33531=CARTESIAN_POINT('Ctrl Pts',(1.76997111386806,1.,-1.14000548337));
#33532=CARTESIAN_POINT('Ctrl Pts',(1.77313777896234,1.,-1.14543858226948));
#33533=CARTESIAN_POINT('Ctrl Pts',(1.77627422557034,1.,-1.15090197841531));
#33534=CARTESIAN_POINT('Ctrl Pts',(1.77938085564261,1.,-1.15639547194689));
#33535=CARTESIAN_POINT('Ctrl Pts',(1.78245795880949,1.,-1.16191881298458));
#33536=CARTESIAN_POINT('Ctrl Pts',(1.78550566040349,1.,-1.16747166312239));
#33537=CARTESIAN_POINT('Ctrl Pts',(1.78852398877523,1.,-1.17305363177265));
#33538=CARTESIAN_POINT('Ctrl Pts',(1.79151291552646,1.,-1.17866429440781));
#33539=CARTESIAN_POINT('Ctrl Pts',(1.79447240321572,1.,-1.18430321697471));
#33540=CARTESIAN_POINT('Ctrl Pts',(1.79740245923649,1.,-1.1899699793456));
#33541=CARTESIAN_POINT('Ctrl Pts',(1.80030314370121,1.,-1.19566418930405));
#33542=CARTESIAN_POINT('Ctrl Pts',(1.8031745483882,1.,-1.2013854893912));
#33543=CARTESIAN_POINT('Ctrl Pts',(1.80601678480772,1.,-1.20713356605519));
#33544=CARTESIAN_POINT('Ctrl Pts',(1.80882996916931,1.,-1.2129081570818));
#33545=CARTESIAN_POINT('Ctrl Pts',(1.81161420806172,1.,-1.2187090610323));
#33546=CARTESIAN_POINT('Ctrl Pts',(1.81436959209778,1.,-1.22453613304507));
#33547=CARTESIAN_POINT('Ctrl Pts',(1.81655087183054,1.,-1.22921864890975));
#33548=CARTESIAN_POINT('Ctrl Pts',(1.81817389920914,1.,-1.23274224526804));
#33549=CARTESIAN_POINT('Ctrl Pts',(1.81925017193531,1.,-1.23509651170384));
#33550=CARTESIAN_POINT('Ctrl Pts',(1.81978687191668,1.,-1.23627494547115));
#33551=CARTESIAN_POINT('',(1.5055822144029,0.,-0.892032620296855));
#33552=CARTESIAN_POINT('Origin',(0.,0.,0.));
#33553=CARTESIAN_POINT('',(1.60662857109684,1.,-0.693717979106306));
#33554=CARTESIAN_POINT('Origin',(0.,1.,0.));
#33555=CARTESIAN_POINT('',(1.60662857109684,0.,-0.693717979106308));
#33556=CARTESIAN_POINT('Ctrl Pts',(2.0698113262342,-1.,-0.745574324794401));
#33557=CARTESIAN_POINT('Ctrl Pts',(2.0698113262342,1.,-0.745574324794401));
#33558=CARTESIAN_POINT('Ctrl Pts',(2.06854248895728,-1.,-0.745832791378367));
#33559=CARTESIAN_POINT('Ctrl Pts',(2.06854248895728,1.,-0.745832791378367));
#33560=CARTESIAN_POINT('Ctrl Pts',(2.06600523016815,-1.,-0.746345871544201));
#33561=CARTESIAN_POINT('Ctrl Pts',(2.06600523016815,1.,-0.746345871544201));
#33562=CARTESIAN_POINT('Ctrl Pts',(2.06220058927826,-1.,-0.74710393278792));
#33563=CARTESIAN_POINT('Ctrl Pts',(2.06220058927826,1.,-0.74710393278792));
#33564=CARTESIAN_POINT('Ctrl Pts',(2.05713023031006,-1.,-0.748091554183803));
#33565=CARTESIAN_POINT('Ctrl Pts',(2.05713023031006,1.,-0.748091554183803));
#33566=CARTESIAN_POINT('Ctrl Pts',(2.05079645592154,-1.,-0.749287468665046));
#33567=CARTESIAN_POINT('Ctrl Pts',(2.05079645592154,1.,-0.749287468665046));
#33568=CARTESIAN_POINT('Ctrl Pts',(2.04446689147979,-1.,-0.750444657875576));
#33569=CARTESIAN_POINT('Ctrl Pts',(2.04446689147979,1.,-0.750444657875576));
#33570=CARTESIAN_POINT('Ctrl Pts',(2.03814160092099,-1.,-0.751562963361115));
#33571=CARTESIAN_POINT('Ctrl Pts',(2.03814160092099,1.,-0.751562963361115));
#33572=CARTESIAN_POINT('Ctrl Pts',(2.03182068456221,-1.,-0.752642180487211));
#33573=CARTESIAN_POINT('Ctrl Pts',(2.03182068456221,1.,-0.752642180487211));
#33574=CARTESIAN_POINT('Ctrl Pts',(2.02550428623313,-1.,-0.753682061112768));
#33575=CARTESIAN_POINT('Ctrl Pts',(2.02550428623313,1.,-0.753682061112768));
#33576=CARTESIAN_POINT('Ctrl Pts',(2.01919259405809,-1.,-0.754682330722816));
#33577=CARTESIAN_POINT('Ctrl Pts',(2.01919259405809,1.,-0.754682330722816));
#33578=CARTESIAN_POINT('Ctrl Pts',(2.01288584328084,-1.,-0.755642704957865));
#33579=CARTESIAN_POINT('Ctrl Pts',(2.01288584328084,1.,-0.755642704957865));
#33580=CARTESIAN_POINT('Ctrl Pts',(2.0065843158773,-1.,-0.756562904646671));
#33581=CARTESIAN_POINT('Ctrl Pts',(2.0065843158773,1.,-0.756562904646671));
#33582=CARTESIAN_POINT('Ctrl Pts',(2.00028834739178,-1.,-0.757442676862724));
#33583=CARTESIAN_POINT('Ctrl Pts',(2.00028834739178,1.,-0.757442676862724));
#33584=CARTESIAN_POINT('Ctrl Pts',(1.99399831098817,-1.,-0.758281796766761));
#33585=CARTESIAN_POINT('Ctrl Pts',(1.99399831098817,1.,-0.758281796766761));
#33586=CARTESIAN_POINT('Ctrl Pts',(1.98771456680874,-1.,-0.759080037802488));
#33587=CARTESIAN_POINT('Ctrl Pts',(1.98771456680874,1.,-0.759080037802488));
#33588=CARTESIAN_POINT('Ctrl Pts',(1.98143741418172,-1.,-0.75983714745219));
#33589=CARTESIAN_POINT('Ctrl Pts',(1.98143741418172,1.,-0.75983714745219));
#33590=CARTESIAN_POINT('Ctrl Pts',(1.97516705321494,-1.,-0.760552825409757));
#33591=CARTESIAN_POINT('Ctrl Pts',(1.97516705321494,1.,-0.760552825409757));
#33592=CARTESIAN_POINT('Ctrl Pts',(1.96890351582499,-1.,-0.761226690483821));
#33593=CARTESIAN_POINT('Ctrl Pts',(1.96890351582499,1.,-0.761226690483821));
#33594=CARTESIAN_POINT('Ctrl Pts',(1.96264672744186,-1.,-0.761858300014424));
#33595=CARTESIAN_POINT('Ctrl Pts',(1.96264672744186,1.,-0.761858300014424));
#33596=CARTESIAN_POINT('Ctrl Pts',(1.95639665309869,-1.,-0.762447203806179));
#33597=CARTESIAN_POINT('Ctrl Pts',(1.95639665309869,1.,-0.762447203806179));
#33598=CARTESIAN_POINT('Ctrl Pts',(1.95015342590024,-1.,-0.762992990878769));
#33599=CARTESIAN_POINT('Ctrl Pts',(1.95015342590024,1.,-0.762992990878769));
#33600=CARTESIAN_POINT('Ctrl Pts',(1.9439174661764,-1.,-0.763495333538629));
#33601=CARTESIAN_POINT('Ctrl Pts',(1.9439174661764,1.,-0.763495333538629));
#33602=CARTESIAN_POINT('Ctrl Pts',(1.93768964875886,-1.,-0.763954049121459));
#33603=CARTESIAN_POINT('Ctrl Pts',(1.93768964875886,1.,-0.763954049121459));
#33604=CARTESIAN_POINT('Ctrl Pts',(1.93147105496382,-1.,-0.764369010673941));
#33605=CARTESIAN_POINT('Ctrl Pts',(1.93147105496382,1.,-0.764369010673941));
#33606=CARTESIAN_POINT('Ctrl Pts',(1.92526263537048,-1.,-0.764740025488212));
#33607=CARTESIAN_POINT('Ctrl Pts',(1.92526263537048,1.,-0.764740025488212));
#33608=CARTESIAN_POINT('Ctrl Pts',(1.91906491634196,-1.,-0.765066729667089));
#33609=CARTESIAN_POINT('Ctrl Pts',(1.91906491634196,1.,-0.765066729667089));
#33610=CARTESIAN_POINT('Ctrl Pts',(1.91287765805169,-1.,-0.765348465884722));
#33611=CARTESIAN_POINT('Ctrl Pts',(1.91287765805169,1.,-0.765348465884722));
#33612=CARTESIAN_POINT('Ctrl Pts',(1.90669961402356,-1.,-0.765584196937919));
#33613=CARTESIAN_POINT('Ctrl Pts',(1.90669961402356,1.,-0.765584196937919));
#33614=CARTESIAN_POINT('Ctrl Pts',(1.90052930393596,-1.,-0.765772772593386));
#33615=CARTESIAN_POINT('Ctrl Pts',(1.90052930393596,1.,-0.765772772593386));
#33616=CARTESIAN_POINT('Ctrl Pts',(1.89436577771388,-1.,-0.765913193856978));
#33617=CARTESIAN_POINT('Ctrl Pts',(1.89436577771388,1.,-0.765913193856978));
#33618=CARTESIAN_POINT('Ctrl Pts',(1.88820926433409,-1.,-0.766004837062091));
#33619=CARTESIAN_POINT('Ctrl Pts',(1.88820926433409,1.,-0.766004837062091));
#33620=CARTESIAN_POINT('Ctrl Pts',(1.88206215302561,-1.,-0.766047794851865));
#33621=CARTESIAN_POINT('Ctrl Pts',(1.88206215302561,1.,-0.766047794851865));
#33622=CARTESIAN_POINT('Ctrl Pts',(1.87592888967883,-1.,-0.766042837036744));
#33623=CARTESIAN_POINT('Ctrl Pts',(1.87592888967883,1.,-0.766042837036744));
#33624=CARTESIAN_POINT('Ctrl Pts',(1.86981398314341,-1.,-0.765990708546091));
#33625=CARTESIAN_POINT('Ctrl Pts',(1.86981398314341,1.,-0.765990708546091));
#33626=CARTESIAN_POINT('Ctrl Pts',(1.86372027063312,-1.,-0.765891519092547));
#33627=CARTESIAN_POINT('Ctrl Pts',(1.86372027063312,1.,-0.765891519092547));
#33628=CARTESIAN_POINT('Ctrl Pts',(1.85764741390394,-1.,-0.765744212909319));
#33629=CARTESIAN_POINT('Ctrl Pts',(1.85764741390394,1.,-0.765744212909319));
#33630=CARTESIAN_POINT('Ctrl Pts',(1.85158945130063,-1.,-0.765545710619063));
#33631=CARTESIAN_POINT('Ctrl Pts',(1.85158945130063,1.,-0.765545710619063));
#33632=CARTESIAN_POINT('Ctrl Pts',(1.84553698875924,-1.,-0.765291664862029));
#33633=CARTESIAN_POINT('Ctrl Pts',(1.84553698875924,1.,-0.765291664862029));
#33634=CARTESIAN_POINT('Ctrl Pts',(1.83948181064835,-1.,-0.764978057881738));
#33635=CARTESIAN_POINT('Ctrl Pts',(1.83948181064835,1.,-0.764978057881738));
#33636=CARTESIAN_POINT('Ctrl Pts',(1.83342077227142,-1.,-0.764602549687853));
#33637=CARTESIAN_POINT('Ctrl Pts',(1.83342077227142,1.,-0.764602549687853));
#33638=CARTESIAN_POINT('Ctrl Pts',(1.82735991200065,-1.,-0.764165902605995));
#33639=CARTESIAN_POINT('Ctrl Pts',(1.82735991200065,1.,-0.764165902605995));
#33640=CARTESIAN_POINT('Ctrl Pts',(1.82131873145266,-1.,-0.763673465462727));
#33641=CARTESIAN_POINT('Ctrl Pts',(1.82131873145266,1.,-0.763673465462727));
#33642=CARTESIAN_POINT('Ctrl Pts',(1.8153211840553,-1.,-0.763132003836634));
#33643=CARTESIAN_POINT('Ctrl Pts',(1.8153211840553,1.,-0.763132003836634));
#33644=CARTESIAN_POINT('Ctrl Pts',(1.80938551463965,-1.,-0.762546129463938));
#33645=CARTESIAN_POINT('Ctrl Pts',(1.80938551463965,1.,-0.762546129463938));
#33646=CARTESIAN_POINT('Ctrl Pts',(1.80351583877342,-1.,-0.761915336443547));
#33647=CARTESIAN_POINT('Ctrl Pts',(1.80351583877342,1.,-0.761915336443547));
#33648=CARTESIAN_POINT('Ctrl Pts',(1.79768986997783,-1.,-0.761229695230558));
#33649=CARTESIAN_POINT('Ctrl Pts',(1.79768986997783,1.,-0.761229695230558));
#33650=CARTESIAN_POINT('Ctrl Pts',(1.7918581561088,-1.,-0.760469555880749));
#33651=CARTESIAN_POINT('Ctrl Pts',(1.7918581561088,1.,-0.760469555880749));
#33652=CARTESIAN_POINT('Ctrl Pts',(1.78596964884604,-1.,-0.75961440111019));
#33653=CARTESIAN_POINT('Ctrl Pts',(1.78596964884604,1.,-0.75961440111019));
#33654=CARTESIAN_POINT('Ctrl Pts',(1.77999411220945,-1.,-0.758650626677519));
#33655=CARTESIAN_POINT('Ctrl Pts',(1.77999411220945,1.,-0.758650626677519));
#33656=CARTESIAN_POINT('Ctrl Pts',(1.77394167108292,-1.,-0.757578264077029));
#33657=CARTESIAN_POINT('Ctrl Pts',(1.77394167108292,1.,-0.757578264077029));
#33658=CARTESIAN_POINT('Ctrl Pts',(1.76789396002998,-1.,-0.75642189602781));
#33659=CARTESIAN_POINT('Ctrl Pts',(1.76789396002998,1.,-0.75642189602781));
#33660=CARTESIAN_POINT('Ctrl Pts',(1.76197817240128,-1.,-0.755220979974462));
#33661=CARTESIAN_POINT('Ctrl Pts',(1.76197817240128,1.,-0.755220979974462));
#33662=CARTESIAN_POINT('Ctrl Pts',(1.75631083600019,-1.,-0.754009254027829));
#33663=CARTESIAN_POINT('Ctrl Pts',(1.75631083600019,1.,-0.754009254027829));
#33664=CARTESIAN_POINT('Ctrl Pts',(1.75095139468794,-1.,-0.752797683531314));
#33665=CARTESIAN_POINT('Ctrl Pts',(1.75095139468794,1.,-0.752797683531314));
#33666=CARTESIAN_POINT('Ctrl Pts',(1.74585086852502,-1.,-0.751555614164483));
#33667=CARTESIAN_POINT('Ctrl Pts',(1.74585086852502,1.,-0.751555614164483));
#33668=CARTESIAN_POINT('Ctrl Pts',(1.74080458267114,-1.,-0.75019343598125));
#33669=CARTESIAN_POINT('Ctrl Pts',(1.74080458267114,1.,-0.75019343598125));
#33670=CARTESIAN_POINT('Ctrl Pts',(1.7355035168033,-1.,-0.74858246295687));
#33671=CARTESIAN_POINT('Ctrl Pts',(1.7355035168033,1.,-0.74858246295687));
#33672=CARTESIAN_POINT('Ctrl Pts',(1.72958533647714,-1.,-0.746574710097752));
#33673=CARTESIAN_POINT('Ctrl Pts',(1.72958533647714,1.,-0.746574710097752));
#33674=CARTESIAN_POINT('Ctrl Pts',(1.72268229916769,-1.,-0.744021445433094));
#33675=CARTESIAN_POINT('Ctrl Pts',(1.72268229916769,1.,-0.744021445433094));
#33676=CARTESIAN_POINT('Ctrl Pts',(1.71447789751001,-1.,-0.74079516202821));
#33677=CARTESIAN_POINT('Ctrl Pts',(1.71447789751001,1.,-0.74079516202821));
#33678=CARTESIAN_POINT('Ctrl Pts',(1.70473309004249,-1.,-0.736799665716932));
#33679=CARTESIAN_POINT('Ctrl Pts',(1.70473309004249,1.,-0.736799665716932));
#33680=CARTESIAN_POINT('Ctrl Pts',(1.69326921972915,-1.,-0.731963238685357));
#33681=CARTESIAN_POINT('Ctrl Pts',(1.69326921972915,1.,-0.731963238685357));
#33682=CARTESIAN_POINT('Ctrl Pts',(1.67996158451922,-1.,-0.726235967982445));
#33683=CARTESIAN_POINT('Ctrl Pts',(1.67996158451922,1.,-0.726235967982445));
#33684=CARTESIAN_POINT('Ctrl Pts',(1.66472880551777,-1.,-0.71958543378795));
#33685=CARTESIAN_POINT('Ctrl Pts',(1.66472880551777,1.,-0.71958543378795));
#33686=CARTESIAN_POINT('Ctrl Pts',(1.64752408828442,-1.,-0.711993139340448));
#33687=CARTESIAN_POINT('Ctrl Pts',(1.64752408828442,1.,-0.711993139340448));
#33688=CARTESIAN_POINT('Ctrl Pts',(1.6321654166204,-1.,-0.705159151977294));
#33689=CARTESIAN_POINT('Ctrl Pts',(1.6321654166204,1.,-0.705159151977294));
#33690=CARTESIAN_POINT('Ctrl Pts',(1.61974673471117,-1.,-0.699605146398837));
#33691=CARTESIAN_POINT('Ctrl Pts',(1.61974673471117,1.,-0.699605146398837));
#33692=CARTESIAN_POINT('Ctrl Pts',(1.61106790957619,-1.,-0.69571209787897));
#33693=CARTESIAN_POINT('Ctrl Pts',(1.61106790957619,1.,-0.69571209787897));
#33694=CARTESIAN_POINT('Ctrl Pts',(1.60662857109684,-1.,-0.693717979106306));
#33695=CARTESIAN_POINT('Ctrl Pts',(1.60662857109684,1.,-0.693717979106306));
#33696=CARTESIAN_POINT('',(2.0698113262342,1.,-0.745574324794401));
#33697=CARTESIAN_POINT('Ctrl Pts',(2.0698113262342,1.,-0.745574324794401));
#33698=CARTESIAN_POINT('Ctrl Pts',(2.06854248895728,1.,-0.745832791378367));
#33699=CARTESIAN_POINT('Ctrl Pts',(2.06600523016815,1.,-0.746345871544201));
#33700=CARTESIAN_POINT('Ctrl Pts',(2.06220058927826,1.,-0.74710393278792));
#33701=CARTESIAN_POINT('Ctrl Pts',(2.05713023031006,1.,-0.748091554183803));
#33702=CARTESIAN_POINT('Ctrl Pts',(2.05079645592154,1.,-0.749287468665046));
#33703=CARTESIAN_POINT('Ctrl Pts',(2.04446689147979,1.,-0.750444657875576));
#33704=CARTESIAN_POINT('Ctrl Pts',(2.03814160092099,1.,-0.751562963361115));
#33705=CARTESIAN_POINT('Ctrl Pts',(2.03182068456221,1.,-0.752642180487211));
#33706=CARTESIAN_POINT('Ctrl Pts',(2.02550428623313,1.,-0.753682061112768));
#33707=CARTESIAN_POINT('Ctrl Pts',(2.01919259405809,1.,-0.754682330722816));
#33708=CARTESIAN_POINT('Ctrl Pts',(2.01288584328084,1.,-0.755642704957865));
#33709=CARTESIAN_POINT('Ctrl Pts',(2.0065843158773,1.,-0.756562904646671));
#33710=CARTESIAN_POINT('Ctrl Pts',(2.00028834739178,1.,-0.757442676862724));
#33711=CARTESIAN_POINT('Ctrl Pts',(1.99399831098817,1.,-0.758281796766761));
#33712=CARTESIAN_POINT('Ctrl Pts',(1.98771456680874,1.,-0.759080037802488));
#33713=CARTESIAN_POINT('Ctrl Pts',(1.98143741418172,1.,-0.75983714745219));
#33714=CARTESIAN_POINT('Ctrl Pts',(1.97516705321494,1.,-0.760552825409757));
#33715=CARTESIAN_POINT('Ctrl Pts',(1.96890351582499,1.,-0.761226690483821));
#33716=CARTESIAN_POINT('Ctrl Pts',(1.96264672744186,1.,-0.761858300014424));
#33717=CARTESIAN_POINT('Ctrl Pts',(1.95639665309869,1.,-0.762447203806179));
#33718=CARTESIAN_POINT('Ctrl Pts',(1.95015342590024,1.,-0.762992990878769));
#33719=CARTESIAN_POINT('Ctrl Pts',(1.9439174661764,1.,-0.763495333538629));
#33720=CARTESIAN_POINT('Ctrl Pts',(1.93768964875886,1.,-0.763954049121459));
#33721=CARTESIAN_POINT('Ctrl Pts',(1.93147105496382,1.,-0.764369010673941));
#33722=CARTESIAN_POINT('Ctrl Pts',(1.92526263537048,1.,-0.764740025488212));
#33723=CARTESIAN_POINT('Ctrl Pts',(1.91906491634196,1.,-0.765066729667089));
#33724=CARTESIAN_POINT('Ctrl Pts',(1.91287765805169,1.,-0.765348465884722));
#33725=CARTESIAN_POINT('Ctrl Pts',(1.90669961402356,1.,-0.765584196937919));
#33726=CARTESIAN_POINT('Ctrl Pts',(1.90052930393596,1.,-0.765772772593386));
#33727=CARTESIAN_POINT('Ctrl Pts',(1.89436577771388,1.,-0.765913193856978));
#33728=CARTESIAN_POINT('Ctrl Pts',(1.88820926433409,1.,-0.766004837062091));
#33729=CARTESIAN_POINT('Ctrl Pts',(1.88206215302561,1.,-0.766047794851865));
#33730=CARTESIAN_POINT('Ctrl Pts',(1.87592888967883,1.,-0.766042837036744));
#33731=CARTESIAN_POINT('Ctrl Pts',(1.86981398314341,1.,-0.765990708546091));
#33732=CARTESIAN_POINT('Ctrl Pts',(1.86372027063312,1.,-0.765891519092547));
#33733=CARTESIAN_POINT('Ctrl Pts',(1.85764741390394,1.,-0.765744212909319));
#33734=CARTESIAN_POINT('Ctrl Pts',(1.85158945130063,1.,-0.765545710619063));
#33735=CARTESIAN_POINT('Ctrl Pts',(1.84553698875924,1.,-0.765291664862029));
#33736=CARTESIAN_POINT('Ctrl Pts',(1.83948181064835,1.,-0.764978057881738));
#33737=CARTESIAN_POINT('Ctrl Pts',(1.83342077227142,1.,-0.764602549687853));
#33738=CARTESIAN_POINT('Ctrl Pts',(1.82735991200065,1.,-0.764165902605995));
#33739=CARTESIAN_POINT('Ctrl Pts',(1.82131873145266,1.,-0.763673465462727));
#33740=CARTESIAN_POINT('Ctrl Pts',(1.8153211840553,1.,-0.763132003836634));
#33741=CARTESIAN_POINT('Ctrl Pts',(1.80938551463965,1.,-0.762546129463938));
#33742=CARTESIAN_POINT('Ctrl Pts',(1.80351583877342,1.,-0.761915336443547));
#33743=CARTESIAN_POINT('Ctrl Pts',(1.79768986997783,1.,-0.761229695230558));
#33744=CARTESIAN_POINT('Ctrl Pts',(1.7918581561088,1.,-0.760469555880749));
#33745=CARTESIAN_POINT('Ctrl Pts',(1.78596964884604,1.,-0.75961440111019));
#33746=CARTESIAN_POINT('Ctrl Pts',(1.77999411220945,1.,-0.758650626677519));
#33747=CARTESIAN_POINT('Ctrl Pts',(1.77394167108292,1.,-0.757578264077029));
#33748=CARTESIAN_POINT('Ctrl Pts',(1.76789396002998,1.,-0.75642189602781));
#33749=CARTESIAN_POINT('Ctrl Pts',(1.76197817240128,1.,-0.755220979974462));
#33750=CARTESIAN_POINT('Ctrl Pts',(1.75631083600019,1.,-0.754009254027829));
#33751=CARTESIAN_POINT('Ctrl Pts',(1.75095139468794,1.,-0.752797683531314));
#33752=CARTESIAN_POINT('Ctrl Pts',(1.74585086852502,1.,-0.751555614164483));
#33753=CARTESIAN_POINT('Ctrl Pts',(1.74080458267114,1.,-0.75019343598125));
#33754=CARTESIAN_POINT('Ctrl Pts',(1.7355035168033,1.,-0.74858246295687));
#33755=CARTESIAN_POINT('Ctrl Pts',(1.72958533647714,1.,-0.746574710097752));
#33756=CARTESIAN_POINT('Ctrl Pts',(1.72268229916769,1.,-0.744021445433094));
#33757=CARTESIAN_POINT('Ctrl Pts',(1.71447789751001,1.,-0.74079516202821));
#33758=CARTESIAN_POINT('Ctrl Pts',(1.70473309004249,1.,-0.736799665716932));
#33759=CARTESIAN_POINT('Ctrl Pts',(1.69326921972915,1.,-0.731963238685357));
#33760=CARTESIAN_POINT('Ctrl Pts',(1.67996158451922,1.,-0.726235967982445));
#33761=CARTESIAN_POINT('Ctrl Pts',(1.66472880551777,1.,-0.71958543378795));
#33762=CARTESIAN_POINT('Ctrl Pts',(1.64752408828442,1.,-0.711993139340448));
#33763=CARTESIAN_POINT('Ctrl Pts',(1.6321654166204,1.,-0.705159151977294));
#33764=CARTESIAN_POINT('Ctrl Pts',(1.61974673471117,1.,-0.699605146398837));
#33765=CARTESIAN_POINT('Ctrl Pts',(1.61106790957619,1.,-0.69571209787897));
#33766=CARTESIAN_POINT('Ctrl Pts',(1.60662857109684,1.,-0.693717979106306));
#33767=CARTESIAN_POINT('',(2.0698113262342,0.,-0.745574324794401));
#33768=CARTESIAN_POINT('Origin',(2.11275013067528,0.,-0.61342227326009));
#33769=CARTESIAN_POINT('',(2.11275013067528,1.,-0.61342227326009));
#33770=CARTESIAN_POINT('',(2.0698113262342,1.,-0.745574324794401));
#33771=CARTESIAN_POINT('',(2.11275013067528,0.,-0.61342227326009));
#33772=CARTESIAN_POINT('Ctrl Pts',(1.7075470150345,-1.,-0.383122945602004));
#33773=CARTESIAN_POINT('Ctrl Pts',(1.7075470150345,1.,-0.383122945602004));
#33774=CARTESIAN_POINT('Ctrl Pts',(1.71231062891958,-1.,-0.384119047315542));
#33775=CARTESIAN_POINT('Ctrl Pts',(1.71231062891958,1.,-0.384119047315542));
#33776=CARTESIAN_POINT('Ctrl Pts',(1.72162022246158,-1.,-0.38607079032701));
#33777=CARTESIAN_POINT('Ctrl Pts',(1.72162022246158,1.,-0.38607079032701));
#33778=CARTESIAN_POINT('Ctrl Pts',(1.7349317097561,-1.,-0.388877023509192));
#33779=CARTESIAN_POINT('Ctrl Pts',(1.7349317097561,1.,-0.388877023509192));
#33780=CARTESIAN_POINT('Ctrl Pts',(1.75137405313962,-1.,-0.392375812294307));
#33781=CARTESIAN_POINT('Ctrl Pts',(1.75137405313962,1.,-0.392375812294307));
#33782=CARTESIAN_POINT('Ctrl Pts',(1.7697556004756,-1.,-0.39634619612042));
#33783=CARTESIAN_POINT('Ctrl Pts',(1.7697556004756,1.,-0.39634619612042));
#33784=CARTESIAN_POINT('Ctrl Pts',(1.78598826347533,-1.,-0.399919403783081));
#33785=CARTESIAN_POINT('Ctrl Pts',(1.78598826347533,1.,-0.399919403783081));
#33786=CARTESIAN_POINT('Ctrl Pts',(1.80012077176221,-1.,-0.403107976170441));
#33787=CARTESIAN_POINT('Ctrl Pts',(1.80012077176221,1.,-0.403107976170441));
#33788=CARTESIAN_POINT('Ctrl Pts',(1.81223801813988,-1.,-0.405933518411838));
#33789=CARTESIAN_POINT('Ctrl Pts',(1.81223801813988,1.,-0.405933518411838));
#33790=CARTESIAN_POINT('Ctrl Pts',(1.8224702267854,-1.,-0.408428948108534));
#33791=CARTESIAN_POINT('Ctrl Pts',(1.8224702267854,1.,-0.408428948108534));
#33792=CARTESIAN_POINT('Ctrl Pts',(1.83100408895216,-1.,-0.410641256301675));
#33793=CARTESIAN_POINT('Ctrl Pts',(1.83100408895216,1.,-0.410641256301675));
#33794=CARTESIAN_POINT('Ctrl Pts',(1.83808953475839,-1.,-0.412633125322162));
#33795=CARTESIAN_POINT('Ctrl Pts',(1.83808953475839,1.,-0.412633125322162));
#33796=CARTESIAN_POINT('Ctrl Pts',(1.8440575707371,-1.,-0.41448743825434));
#33797=CARTESIAN_POINT('Ctrl Pts',(1.8440575707371,1.,-0.41448743825434));
#33798=CARTESIAN_POINT('Ctrl Pts',(1.84929312929882,-1.,-0.416300022038864));
#33799=CARTESIAN_POINT('Ctrl Pts',(1.84929312929882,1.,-0.416300022038864));
#33800=CARTESIAN_POINT('Ctrl Pts',(1.85417632856234,-1.,-0.418164129143534));
#33801=CARTESIAN_POINT('Ctrl Pts',(1.85417632856234,1.,-0.418164129143534));
#33802=CARTESIAN_POINT('Ctrl Pts',(1.85903281096686,-1.,-0.42015728797562));
#33803=CARTESIAN_POINT('Ctrl Pts',(1.85903281096686,1.,-0.42015728797562));
#33804=CARTESIAN_POINT('Ctrl Pts',(1.86408083334028,-1.,-0.422327307418275));
#33805=CARTESIAN_POINT('Ctrl Pts',(1.86408083334028,1.,-0.422327307418275));
#33806=CARTESIAN_POINT('Ctrl Pts',(1.86937803944323,-1.,-0.424678177291359));
#33807=CARTESIAN_POINT('Ctrl Pts',(1.86937803944323,1.,-0.424678177291359));
#33808=CARTESIAN_POINT('Ctrl Pts',(1.87486989291484,-1.,-0.427183828519102));
#33809=CARTESIAN_POINT('Ctrl Pts',(1.87486989291484,1.,-0.427183828519102));
#33810=CARTESIAN_POINT('Ctrl Pts',(1.88044229001832,-1.,-0.429803062482345));
#33811=CARTESIAN_POINT('Ctrl Pts',(1.88044229001832,1.,-0.429803062482345));
#33812=CARTESIAN_POINT('Ctrl Pts',(1.88596913666793,-1.,-0.432493038548748));
#33813=CARTESIAN_POINT('Ctrl Pts',(1.88596913666793,1.,-0.432493038548748));
#33814=CARTESIAN_POINT('Ctrl Pts',(1.89136993975504,-1.,-0.435225660963383));
#33815=CARTESIAN_POINT('Ctrl Pts',(1.89136993975504,1.,-0.435225660963383));
#33816=CARTESIAN_POINT('Ctrl Pts',(1.89663648956466,-1.,-0.437995003948244));
#33817=CARTESIAN_POINT('Ctrl Pts',(1.89663648956466,1.,-0.437995003948244));
#33818=CARTESIAN_POINT('Ctrl Pts',(1.90180124389086,-1.,-0.440807833704038));
#33819=CARTESIAN_POINT('Ctrl Pts',(1.90180124389086,1.,-0.440807833704038));
#33820=CARTESIAN_POINT('Ctrl Pts',(1.90691756144898,-1.,-0.443677556849151));
#33821=CARTESIAN_POINT('Ctrl Pts',(1.90691756144898,1.,-0.443677556849151));
#33822=CARTESIAN_POINT('Ctrl Pts',(1.9120369998112,-1.,-0.446617343485711));
#33823=CARTESIAN_POINT('Ctrl Pts',(1.9120369998112,1.,-0.446617343485711));
#33824=CARTESIAN_POINT('Ctrl Pts',(1.91718342555755,-1.,-0.449632260106662));
#33825=CARTESIAN_POINT('Ctrl Pts',(1.91718342555755,1.,-0.449632260106662));
#33826=CARTESIAN_POINT('Ctrl Pts',(1.92235380648502,-1.,-0.452719478359433));
#33827=CARTESIAN_POINT('Ctrl Pts',(1.92235380648502,1.,-0.452719478359433));
#33828=CARTESIAN_POINT('Ctrl Pts',(1.92753067150476,-1.,-0.455872005174371));
#33829=CARTESIAN_POINT('Ctrl Pts',(1.92753067150476,1.,-0.455872005174371));
#33830=CARTESIAN_POINT('Ctrl Pts',(1.93269066517934,-1.,-0.459081234547926));
#33831=CARTESIAN_POINT('Ctrl Pts',(1.93269066517934,1.,-0.459081234547926));
#33832=CARTESIAN_POINT('Ctrl Pts',(1.93781486640821,-1.,-0.462340031009057));
#33833=CARTESIAN_POINT('Ctrl Pts',(1.93781486640821,1.,-0.462340031009057));
#33834=CARTESIAN_POINT('Ctrl Pts',(1.9428979419619,-1.,-0.46564546202603));
#33835=CARTESIAN_POINT('Ctrl Pts',(1.9428979419619,1.,-0.46564546202603));
#33836=CARTESIAN_POINT('Ctrl Pts',(1.94794381136514,-1.,-0.468997482913135));
#33837=CARTESIAN_POINT('Ctrl Pts',(1.94794381136514,1.,-0.468997482913135));
#33838=CARTESIAN_POINT('Ctrl Pts',(1.95296148278133,-1.,-0.472397672264072));
#33839=CARTESIAN_POINT('Ctrl Pts',(1.95296148278133,1.,-0.472397672264072));
#33840=CARTESIAN_POINT('Ctrl Pts',(1.95796111148177,-1.,-0.475848034683176));
#33841=CARTESIAN_POINT('Ctrl Pts',(1.95796111148177,1.,-0.475848034683176));
#33842=CARTESIAN_POINT('Ctrl Pts',(1.96294933055943,-1.,-0.479349583074855));
#33843=CARTESIAN_POINT('Ctrl Pts',(1.96294933055943,1.,-0.479349583074855));
#33844=CARTESIAN_POINT('Ctrl Pts',(1.96792703422362,-1.,-0.482901662120691));
#33845=CARTESIAN_POINT('Ctrl Pts',(1.96792703422362,1.,-0.482901662120691));
#33846=CARTESIAN_POINT('Ctrl Pts',(1.97289186263272,-1.,-0.486502692907659));
#33847=CARTESIAN_POINT('Ctrl Pts',(1.97289186263272,1.,-0.486502692907659));
#33848=CARTESIAN_POINT('Ctrl Pts',(1.97783973019229,-1.,-0.490150627860953));
#33849=CARTESIAN_POINT('Ctrl Pts',(1.97783973019229,1.,-0.490150627860953));
#33850=CARTESIAN_POINT('Ctrl Pts',(1.98276658761821,-1.,-0.493843476541495));
#33851=CARTESIAN_POINT('Ctrl Pts',(1.98276658761821,1.,-0.493843476541495));
#33852=CARTESIAN_POINT('Ctrl Pts',(1.98767044752932,-1.,-0.497579909545574));
#33853=CARTESIAN_POINT('Ctrl Pts',(1.98767044752932,1.,-0.497579909545574));
#33854=CARTESIAN_POINT('Ctrl Pts',(1.99255149126155,-1.,-0.501359287727146));
#33855=CARTESIAN_POINT('Ctrl Pts',(1.99255149126155,1.,-0.501359287727146));
#33856=CARTESIAN_POINT('Ctrl Pts',(1.99741107463572,-1.,-0.505181361323026));
#33857=CARTESIAN_POINT('Ctrl Pts',(1.99741107463572,1.,-0.505181361323026));
#33858=CARTESIAN_POINT('Ctrl Pts',(2.00225107134734,-1.,-0.509046069886157));
#33859=CARTESIAN_POINT('Ctrl Pts',(2.00225107134734,1.,-0.509046069886157));
#33860=CARTESIAN_POINT('Ctrl Pts',(2.00707309946949,-1.,-0.512953306961793));
#33861=CARTESIAN_POINT('Ctrl Pts',(2.00707309946949,1.,-0.512953306961793));
#33862=CARTESIAN_POINT('Ctrl Pts',(2.01187773939242,-1.,-0.516902681728687));
#33863=CARTESIAN_POINT('Ctrl Pts',(2.01187773939242,1.,-0.516902681728687));
#33864=CARTESIAN_POINT('Ctrl Pts',(2.01666477917286,-1.,-0.520893590399371));
#33865=CARTESIAN_POINT('Ctrl Pts',(2.01666477917286,1.,-0.520893590399371));
#33866=CARTESIAN_POINT('Ctrl Pts',(2.02143356304698,-1.,-0.524925318333476));
#33867=CARTESIAN_POINT('Ctrl Pts',(2.02143356304698,1.,-0.524925318333476));
#33868=CARTESIAN_POINT('Ctrl Pts',(2.0261832908329,-1.,-0.528997127241914));
#33869=CARTESIAN_POINT('Ctrl Pts',(2.0261832908329,1.,-0.528997127241914));
#33870=CARTESIAN_POINT('Ctrl Pts',(2.03091336214426,-1.,-0.533108355132977));
#33871=CARTESIAN_POINT('Ctrl Pts',(2.03091336214426,1.,-0.533108355132977));
#33872=CARTESIAN_POINT('Ctrl Pts',(2.03562362954037,-1.,-0.537258489833262));
#33873=CARTESIAN_POINT('Ctrl Pts',(2.03562362954037,1.,-0.537258489833262));
#33874=CARTESIAN_POINT('Ctrl Pts',(2.04031422690527,-1.,-0.541447120615659));
#33875=CARTESIAN_POINT('Ctrl Pts',(2.04031422690527,1.,-0.541447120615659));
#33876=CARTESIAN_POINT('Ctrl Pts',(2.04498544714588,-1.,-0.54567390381743));
#33877=CARTESIAN_POINT('Ctrl Pts',(2.04498544714588,1.,-0.54567390381743));
#33878=CARTESIAN_POINT('Ctrl Pts',(2.04963761077958,-1.,-0.549938525150295));
#33879=CARTESIAN_POINT('Ctrl Pts',(2.04963761077958,1.,-0.549938525150295));
#33880=CARTESIAN_POINT('Ctrl Pts',(2.05427091604413,-1.,-0.554240657463906));
#33881=CARTESIAN_POINT('Ctrl Pts',(2.05427091604413,1.,-0.554240657463906));
#33882=CARTESIAN_POINT('Ctrl Pts',(2.05888537756462,-1.,-0.558579940185152));
#33883=CARTESIAN_POINT('Ctrl Pts',(2.05888537756462,1.,-0.558579940185152));
#33884=CARTESIAN_POINT('Ctrl Pts',(2.06348090160589,-1.,-0.562955993082262));
#33885=CARTESIAN_POINT('Ctrl Pts',(2.06348090160589,1.,-0.562955993082262));
#33886=CARTESIAN_POINT('Ctrl Pts',(2.06805732997334,-1.,-0.567368421181087));
#33887=CARTESIAN_POINT('Ctrl Pts',(2.06805732997334,1.,-0.567368421181087));
#33888=CARTESIAN_POINT('Ctrl Pts',(2.07261449292824,-1.,-0.571816823242603));
#33889=CARTESIAN_POINT('Ctrl Pts',(2.07261449292824,1.,-0.571816823242603));
#33890=CARTESIAN_POINT('Ctrl Pts',(2.07715226767559,-1.,-0.576300797416845));
#33891=CARTESIAN_POINT('Ctrl Pts',(2.07715226767559,1.,-0.576300797416845));
#33892=CARTESIAN_POINT('Ctrl Pts',(2.08167059018418,-1.,-0.580819952108064));
#33893=CARTESIAN_POINT('Ctrl Pts',(2.08167059018418,1.,-0.580819952108064));
#33894=CARTESIAN_POINT('Ctrl Pts',(2.08616943727951,-1.,-0.585373918991617));
#33895=CARTESIAN_POINT('Ctrl Pts',(2.08616943727951,1.,-0.585373918991617));
#33896=CARTESIAN_POINT('Ctrl Pts',(2.09064881812129,-1.,-0.589962365403406));
#33897=CARTESIAN_POINT('Ctrl Pts',(2.09064881812129,1.,-0.589962365403406));
#33898=CARTESIAN_POINT('Ctrl Pts',(2.0951087622027,-1.,-0.594585006052162));
#33899=CARTESIAN_POINT('Ctrl Pts',(2.0951087622027,1.,-0.594585006052162));
#33900=CARTESIAN_POINT('Ctrl Pts',(2.0995493086477,-1.,-0.599241616420534));
#33901=CARTESIAN_POINT('Ctrl Pts',(2.0995493086477,1.,-0.599241616420534));
#33902=CARTESIAN_POINT('Ctrl Pts',(2.10397049886949,-1.,-0.60393203073603));
#33903=CARTESIAN_POINT('Ctrl Pts',(2.10397049886949,1.,-0.60393203073603));
#33904=CARTESIAN_POINT('Ctrl Pts',(2.1074919961518,-1.,-0.607711315454876));
#33905=CARTESIAN_POINT('Ctrl Pts',(2.1074919961518,1.,-0.607711315454876));
#33906=CARTESIAN_POINT('Ctrl Pts',(2.11012443807238,-1.,-0.610560911689899));
#33907=CARTESIAN_POINT('Ctrl Pts',(2.11012443807238,1.,-0.610560911689899));
#33908=CARTESIAN_POINT('Ctrl Pts',(2.11187554259986,-1.,-0.6124673655618));
#33909=CARTESIAN_POINT('Ctrl Pts',(2.11187554259986,1.,-0.6124673655618));
#33910=CARTESIAN_POINT('Ctrl Pts',(2.11275013067528,-1.,-0.61342227326009));
#33911=CARTESIAN_POINT('Ctrl Pts',(2.11275013067528,1.,-0.61342227326009));
#33912=CARTESIAN_POINT('',(1.7075470150345,1.,-0.383122945602004));
#33913=CARTESIAN_POINT('Ctrl Pts',(1.7075470150345,1.,-0.383122945602004));
#33914=CARTESIAN_POINT('Ctrl Pts',(1.71231062891958,1.,-0.384119047315542));
#33915=CARTESIAN_POINT('Ctrl Pts',(1.72162022246158,1.,-0.38607079032701));
#33916=CARTESIAN_POINT('Ctrl Pts',(1.7349317097561,1.,-0.388877023509192));
#33917=CARTESIAN_POINT('Ctrl Pts',(1.75137405313962,1.,-0.392375812294307));
#33918=CARTESIAN_POINT('Ctrl Pts',(1.7697556004756,1.,-0.39634619612042));
#33919=CARTESIAN_POINT('Ctrl Pts',(1.78598826347533,1.,-0.399919403783081));
#33920=CARTESIAN_POINT('Ctrl Pts',(1.80012077176221,1.,-0.403107976170441));
#33921=CARTESIAN_POINT('Ctrl Pts',(1.81223801813988,1.,-0.405933518411838));
#33922=CARTESIAN_POINT('Ctrl Pts',(1.8224702267854,1.,-0.408428948108534));
#33923=CARTESIAN_POINT('Ctrl Pts',(1.83100408895216,1.,-0.410641256301675));
#33924=CARTESIAN_POINT('Ctrl Pts',(1.83808953475839,1.,-0.412633125322162));
#33925=CARTESIAN_POINT('Ctrl Pts',(1.8440575707371,1.,-0.41448743825434));
#33926=CARTESIAN_POINT('Ctrl Pts',(1.84929312929882,1.,-0.416300022038864));
#33927=CARTESIAN_POINT('Ctrl Pts',(1.85417632856234,1.,-0.418164129143534));
#33928=CARTESIAN_POINT('Ctrl Pts',(1.85903281096686,1.,-0.42015728797562));
#33929=CARTESIAN_POINT('Ctrl Pts',(1.86408083334028,1.,-0.422327307418275));
#33930=CARTESIAN_POINT('Ctrl Pts',(1.86937803944323,1.,-0.424678177291359));
#33931=CARTESIAN_POINT('Ctrl Pts',(1.87486989291484,1.,-0.427183828519102));
#33932=CARTESIAN_POINT('Ctrl Pts',(1.88044229001832,1.,-0.429803062482345));
#33933=CARTESIAN_POINT('Ctrl Pts',(1.88596913666793,1.,-0.432493038548748));
#33934=CARTESIAN_POINT('Ctrl Pts',(1.89136993975504,1.,-0.435225660963383));
#33935=CARTESIAN_POINT('Ctrl Pts',(1.89663648956466,1.,-0.437995003948244));
#33936=CARTESIAN_POINT('Ctrl Pts',(1.90180124389086,1.,-0.440807833704038));
#33937=CARTESIAN_POINT('Ctrl Pts',(1.90691756144898,1.,-0.443677556849151));
#33938=CARTESIAN_POINT('Ctrl Pts',(1.9120369998112,1.,-0.446617343485711));
#33939=CARTESIAN_POINT('Ctrl Pts',(1.91718342555755,1.,-0.449632260106662));
#33940=CARTESIAN_POINT('Ctrl Pts',(1.92235380648502,1.,-0.452719478359433));
#33941=CARTESIAN_POINT('Ctrl Pts',(1.92753067150476,1.,-0.455872005174371));
#33942=CARTESIAN_POINT('Ctrl Pts',(1.93269066517934,1.,-0.459081234547926));
#33943=CARTESIAN_POINT('Ctrl Pts',(1.93781486640821,1.,-0.462340031009057));
#33944=CARTESIAN_POINT('Ctrl Pts',(1.9428979419619,1.,-0.46564546202603));
#33945=CARTESIAN_POINT('Ctrl Pts',(1.94794381136514,1.,-0.468997482913135));
#33946=CARTESIAN_POINT('Ctrl Pts',(1.95296148278133,1.,-0.472397672264072));
#33947=CARTESIAN_POINT('Ctrl Pts',(1.95796111148177,1.,-0.475848034683176));
#33948=CARTESIAN_POINT('Ctrl Pts',(1.96294933055943,1.,-0.479349583074855));
#33949=CARTESIAN_POINT('Ctrl Pts',(1.96792703422362,1.,-0.482901662120691));
#33950=CARTESIAN_POINT('Ctrl Pts',(1.97289186263272,1.,-0.486502692907659));
#33951=CARTESIAN_POINT('Ctrl Pts',(1.97783973019229,1.,-0.490150627860953));
#33952=CARTESIAN_POINT('Ctrl Pts',(1.98276658761821,1.,-0.493843476541495));
#33953=CARTESIAN_POINT('Ctrl Pts',(1.98767044752932,1.,-0.497579909545574));
#33954=CARTESIAN_POINT('Ctrl Pts',(1.99255149126155,1.,-0.501359287727146));
#33955=CARTESIAN_POINT('Ctrl Pts',(1.99741107463572,1.,-0.505181361323026));
#33956=CARTESIAN_POINT('Ctrl Pts',(2.00225107134734,1.,-0.509046069886157));
#33957=CARTESIAN_POINT('Ctrl Pts',(2.00707309946949,1.,-0.512953306961793));
#33958=CARTESIAN_POINT('Ctrl Pts',(2.01187773939242,1.,-0.516902681728687));
#33959=CARTESIAN_POINT('Ctrl Pts',(2.01666477917286,1.,-0.520893590399371));
#33960=CARTESIAN_POINT('Ctrl Pts',(2.02143356304698,1.,-0.524925318333476));
#33961=CARTESIAN_POINT('Ctrl Pts',(2.0261832908329,1.,-0.528997127241914));
#33962=CARTESIAN_POINT('Ctrl Pts',(2.03091336214426,1.,-0.533108355132977));
#33963=CARTESIAN_POINT('Ctrl Pts',(2.03562362954037,1.,-0.537258489833262));
#33964=CARTESIAN_POINT('Ctrl Pts',(2.04031422690527,1.,-0.541447120615659));
#33965=CARTESIAN_POINT('Ctrl Pts',(2.04498544714588,1.,-0.54567390381743));
#33966=CARTESIAN_POINT('Ctrl Pts',(2.04963761077958,1.,-0.549938525150295));
#33967=CARTESIAN_POINT('Ctrl Pts',(2.05427091604413,1.,-0.554240657463906));
#33968=CARTESIAN_POINT('Ctrl Pts',(2.05888537756462,1.,-0.558579940185152));
#33969=CARTESIAN_POINT('Ctrl Pts',(2.06348090160589,1.,-0.562955993082262));
#33970=CARTESIAN_POINT('Ctrl Pts',(2.06805732997334,1.,-0.567368421181087));
#33971=CARTESIAN_POINT('Ctrl Pts',(2.07261449292824,1.,-0.571816823242603));
#33972=CARTESIAN_POINT('Ctrl Pts',(2.07715226767559,1.,-0.576300797416845));
#33973=CARTESIAN_POINT('Ctrl Pts',(2.08167059018418,1.,-0.580819952108064));
#33974=CARTESIAN_POINT('Ctrl Pts',(2.08616943727951,1.,-0.585373918991617));
#33975=CARTESIAN_POINT('Ctrl Pts',(2.09064881812129,1.,-0.589962365403406));
#33976=CARTESIAN_POINT('Ctrl Pts',(2.0951087622027,1.,-0.594585006052162));
#33977=CARTESIAN_POINT('Ctrl Pts',(2.0995493086477,1.,-0.599241616420534));
#33978=CARTESIAN_POINT('Ctrl Pts',(2.10397049886949,1.,-0.60393203073603));
#33979=CARTESIAN_POINT('Ctrl Pts',(2.1074919961518,1.,-0.607711315454876));
#33980=CARTESIAN_POINT('Ctrl Pts',(2.11012443807238,1.,-0.610560911689899));
#33981=CARTESIAN_POINT('Ctrl Pts',(2.11187554259986,1.,-0.6124673655618));
#33982=CARTESIAN_POINT('Ctrl Pts',(2.11275013067528,1.,-0.61342227326009));
#33983=CARTESIAN_POINT('',(1.7075470150345,0.,-0.383122945602001));
#33984=CARTESIAN_POINT('Origin',(0.,0.,0.));
#33985=CARTESIAN_POINT('',(1.74236521665491,1.,-0.163289472382896));
#33986=CARTESIAN_POINT('Origin',(0.,1.,0.));
#33987=CARTESIAN_POINT('',(1.74236521665491,0.,-0.163289472382896));
#33988=CARTESIAN_POINT('Ctrl Pts',(2.19890268624765,-1.,-0.0694764450219582));
#33989=CARTESIAN_POINT('Ctrl Pts',(2.19890268624765,1.,-0.0694764450219582));
#33990=CARTESIAN_POINT('Ctrl Pts',(2.19777582085423,-1.,-0.0701143536325491));
#33991=CARTESIAN_POINT('Ctrl Pts',(2.19777582085423,1.,-0.0701143536325491));
#33992=CARTESIAN_POINT('Ctrl Pts',(2.19552129484002,-1.,-0.0713863779526155));
#33993=CARTESIAN_POINT('Ctrl Pts',(2.19552129484002,1.,-0.0713863779526155));
#33994=CARTESIAN_POINT('Ctrl Pts',(2.19213712013662,-1.,-0.0732830357306726));
#33995=CARTESIAN_POINT('Ctrl Pts',(2.19213712013662,1.,-0.0732830357306726));
#33996=CARTESIAN_POINT('Ctrl Pts',(2.1876201139953,-1.,-0.0757891465836149));
#33997=CARTESIAN_POINT('Ctrl Pts',(2.1876201139953,1.,-0.0757891465836149));
#33998=CARTESIAN_POINT('Ctrl Pts',(2.18196589448887,-1.,-0.0788837727685244));
#33999=CARTESIAN_POINT('Ctrl Pts',(2.18196589448887,1.,-0.0788837727685244));
#34000=CARTESIAN_POINT('Ctrl Pts',(2.176303712113,-1.,-0.0819402680872767));
#34001=CARTESIAN_POINT('Ctrl Pts',(2.176303712113,1.,-0.0819402680872767));
#34002=CARTESIAN_POINT('Ctrl Pts',(2.17063357870952,-1.,-0.0849584620835374));
#34003=CARTESIAN_POINT('Ctrl Pts',(2.17063357870952,1.,-0.0849584620835374));
#34004=CARTESIAN_POINT('Ctrl Pts',(2.16495552645014,-1.,-0.0879381291386924));
#34005=CARTESIAN_POINT('Ctrl Pts',(2.16495552645014,1.,-0.0879381291386924));
#34006=CARTESIAN_POINT('Ctrl Pts',(2.15926961544516,-1.,-0.0908789888107267));
#34007=CARTESIAN_POINT('Ctrl Pts',(2.15926961544516,1.,-0.0908789888107267));
#34008=CARTESIAN_POINT('Ctrl Pts',(2.1535759397817,-1.,-0.0937807218867645));
#34009=CARTESIAN_POINT('Ctrl Pts',(2.1535759397817,1.,-0.0937807218867645));
#34010=CARTESIAN_POINT('Ctrl Pts',(2.14787463531795,-1.,-0.096642985230546));
#34011=CARTESIAN_POINT('Ctrl Pts',(2.14787463531795,1.,-0.096642985230546));
#34012=CARTESIAN_POINT('Ctrl Pts',(2.14216588396025,-1.,-0.0994654261990917));
#34013=CARTESIAN_POINT('Ctrl Pts',(2.14216588396025,1.,-0.0994654261990917));
#34014=CARTESIAN_POINT('Ctrl Pts',(2.13644992667165,-1.,-0.102247700556101));
#34015=CARTESIAN_POINT('Ctrl Pts',(2.13644992667165,1.,-0.102247700556101));
#34016=CARTESIAN_POINT('Ctrl Pts',(2.13072704887293,-1.,-0.10498947915274));
#34017=CARTESIAN_POINT('Ctrl Pts',(2.13072704887293,1.,-0.10498947915274));
#34018=CARTESIAN_POINT('Ctrl Pts',(2.12499752307,-1.,-0.10769043523109));
#34019=CARTESIAN_POINT('Ctrl Pts',(2.12499752307,1.,-0.10769043523109));
#34020=CARTESIAN_POINT('Ctrl Pts',(2.11926155590865,-1.,-0.110350236135025));
#34021=CARTESIAN_POINT('Ctrl Pts',(2.11926155590865,1.,-0.110350236135025));
#34022=CARTESIAN_POINT('Ctrl Pts',(2.11351924490306,-1.,-0.112968534419737));
#34023=CARTESIAN_POINT('Ctrl Pts',(2.11351924490306,1.,-0.112968534419737));
#34024=CARTESIAN_POINT('Ctrl Pts',(2.10777050261309,-1.,-0.115544957687927));
#34025=CARTESIAN_POINT('Ctrl Pts',(2.10777050261309,1.,-0.115544957687927));
#34026=CARTESIAN_POINT('Ctrl Pts',(2.102015121329,-1.,-0.118079107988356));
#34027=CARTESIAN_POINT('Ctrl Pts',(2.102015121329,1.,-0.118079107988356));
#34028=CARTESIAN_POINT('Ctrl Pts',(2.0962529286773,-1.,-0.120570567965122));
#34029=CARTESIAN_POINT('Ctrl Pts',(2.0962529286773,1.,-0.120570567965122));
#34030=CARTESIAN_POINT('Ctrl Pts',(2.09048392424825,-1.,-0.123018905621083));
#34031=CARTESIAN_POINT('Ctrl Pts',(2.09048392424825,1.,-0.123018905621083));
#34032=CARTESIAN_POINT('Ctrl Pts',(2.08470840653643,-1.,-0.125423679412062));
#34033=CARTESIAN_POINT('Ctrl Pts',(2.08470840653643,1.,-0.125423679412062));
#34034=CARTESIAN_POINT('Ctrl Pts',(2.07892715110987,-1.,-0.12778444527612));
#34035=CARTESIAN_POINT('Ctrl Pts',(2.07892715110987,1.,-0.12778444527612));
#34036=CARTESIAN_POINT('Ctrl Pts',(2.07314114713063,-1.,-0.130100748328404));
#34037=CARTESIAN_POINT('Ctrl Pts',(2.07314114713063,1.,-0.130100748328404));
#34038=CARTESIAN_POINT('Ctrl Pts',(2.06735123910326,-1.,-0.132372111547711));
#34039=CARTESIAN_POINT('Ctrl Pts',(2.06735123910326,1.,-0.132372111547711));
#34040=CARTESIAN_POINT('Ctrl Pts',(2.06155781517842,-1.,-0.134598026192106));
#34041=CARTESIAN_POINT('Ctrl Pts',(2.06155781517842,1.,-0.134598026192106));
#34042=CARTESIAN_POINT('Ctrl Pts',(2.05576044414264,-1.,-0.136777941218044));
#34043=CARTESIAN_POINT('Ctrl Pts',(2.05576044414264,1.,-0.136777941218044));
#34044=CARTESIAN_POINT('Ctrl Pts',(2.04995762001328,-1.,-0.138911255368966));
#34045=CARTESIAN_POINT('Ctrl Pts',(2.04995762001328,1.,-0.138911255368966));
#34046=CARTESIAN_POINT('Ctrl Pts',(2.04414757947916,-1.,-0.140997332152546));
#34047=CARTESIAN_POINT('Ctrl Pts',(2.04414757947916,1.,-0.140997332152546));
#34048=CARTESIAN_POINT('Ctrl Pts',(2.03832911025912,-1.,-0.143035515058209));
#34049=CARTESIAN_POINT('Ctrl Pts',(2.03832911025912,1.,-0.143035515058209));
#34050=CARTESIAN_POINT('Ctrl Pts',(2.03250223739942,-1.,-0.145025140186058));
#34051=CARTESIAN_POINT('Ctrl Pts',(2.03250223739942,1.,-0.145025140186058));
#34052=CARTESIAN_POINT('Ctrl Pts',(2.02666926182017,-1.,-0.146965557332583));
#34053=CARTESIAN_POINT('Ctrl Pts',(2.02666926182017,1.,-0.146965557332583));
#34054=CARTESIAN_POINT('Ctrl Pts',(2.02083464969894,-1.,-0.148856124775337));
#34055=CARTESIAN_POINT('Ctrl Pts',(2.02083464969894,1.,-0.148856124775337));
#34056=CARTESIAN_POINT('Ctrl Pts',(2.01500291940238,-1.,-0.150696157673078));
#34057=CARTESIAN_POINT('Ctrl Pts',(2.01500291940238,1.,-0.150696157673078));
#34058=CARTESIAN_POINT('Ctrl Pts',(2.00917680318424,-1.,-0.15248488362145));
#34059=CARTESIAN_POINT('Ctrl Pts',(2.00917680318424,1.,-0.15248488362145));
#34060=CARTESIAN_POINT('Ctrl Pts',(2.00335565310543,-1.,-0.154221403049722));
#34061=CARTESIAN_POINT('Ctrl Pts',(2.00335565310543,1.,-0.154221403049722));
#34062=CARTESIAN_POINT('Ctrl Pts',(1.99753284771497,-1.,-0.155904629548784));
#34063=CARTESIAN_POINT('Ctrl Pts',(1.99753284771497,1.,-0.155904629548784));
#34064=CARTESIAN_POINT('Ctrl Pts',(1.99169810931908,-1.,-0.157533331459227));
#34065=CARTESIAN_POINT('Ctrl Pts',(1.99169810931908,1.,-0.157533331459227));
#34066=CARTESIAN_POINT('Ctrl Pts',(1.98584238283292,-1.,-0.159106226437299));
#34067=CARTESIAN_POINT('Ctrl Pts',(1.98584238283292,1.,-0.159106226437299));
#34068=CARTESIAN_POINT('Ctrl Pts',(1.97996195437559,-1.,-0.160622060784611));
#34069=CARTESIAN_POINT('Ctrl Pts',(1.97996195437559,1.,-0.160622060784611));
#34070=CARTESIAN_POINT('Ctrl Pts',(1.97406280235188,-1.,-0.162079693556289));
#34071=CARTESIAN_POINT('Ctrl Pts',(1.97406280235188,1.,-0.162079693556289));
#34072=CARTESIAN_POINT('Ctrl Pts',(1.96816512677967,-1.,-0.163478185457734));
#34073=CARTESIAN_POINT('Ctrl Pts',(1.96816512677967,1.,-0.163478185457734));
#34074=CARTESIAN_POINT('Ctrl Pts',(1.96229379940136,-1.,-0.164816568920269));
#34075=CARTESIAN_POINT('Ctrl Pts',(1.96229379940136,1.,-0.164816568920269));
#34076=CARTESIAN_POINT('Ctrl Pts',(1.9564675971873,-1.,-0.166093592002813));
#34077=CARTESIAN_POINT('Ctrl Pts',(1.9564675971873,1.,-0.166093592002813));
#34078=CARTESIAN_POINT('Ctrl Pts',(1.95069027794294,-1.,-0.167307501784476));
#34079=CARTESIAN_POINT('Ctrl Pts',(1.95069027794294,1.,-0.167307501784476));
#34080=CARTESIAN_POINT('Ctrl Pts',(1.94493757756931,-1.,-0.168455741607556));
#34081=CARTESIAN_POINT('Ctrl Pts',(1.94493757756931,1.,-0.168455741607556));
#34082=CARTESIAN_POINT('Ctrl Pts',(1.93915639211581,-1.,-0.169534904817491));
#34083=CARTESIAN_POINT('Ctrl Pts',(1.93915639211581,1.,-0.169534904817491));
#34084=CARTESIAN_POINT('Ctrl Pts',(1.93329183155539,-1.,-0.170541253116202));
#34085=CARTESIAN_POINT('Ctrl Pts',(1.93329183155539,1.,-0.170541253116202));
#34086=CARTESIAN_POINT('Ctrl Pts',(1.92731093582036,-1.,-0.171471191532988));
#34087=CARTESIAN_POINT('Ctrl Pts',(1.92731093582036,1.,-0.171471191532988));
#34088=CARTESIAN_POINT('Ctrl Pts',(1.9212233439798,-1.,-0.172321621259514));
#34089=CARTESIAN_POINT('Ctrl Pts',(1.9212233439798,1.,-0.172321621259514));
#34090=CARTESIAN_POINT('Ctrl Pts',(1.91511429159527,-1.,-0.173090695383496));
#34091=CARTESIAN_POINT('Ctrl Pts',(1.91511429159527,1.,-0.173090695383496));
#34092=CARTESIAN_POINT('Ctrl Pts',(1.90911693975267,-1.,-0.173776635257817));
#34093=CARTESIAN_POINT('Ctrl Pts',(1.90911693975267,1.,-0.173776635257817));
#34094=CARTESIAN_POINT('Ctrl Pts',(1.90335253862834,-1.,-0.174375518661085));
#34095=CARTESIAN_POINT('Ctrl Pts',(1.90335253862834,1.,-0.174375518661085));
#34096=CARTESIAN_POINT('Ctrl Pts',(1.89788101117132,-1.,-0.174879405091263));
#34097=CARTESIAN_POINT('Ctrl Pts',(1.89788101117132,1.,-0.174879405091263));
#34098=CARTESIAN_POINT('Ctrl Pts',(1.892646301985,-1.,-0.175274276190844));
#34099=CARTESIAN_POINT('Ctrl Pts',(1.892646301985,1.,-0.175274276190844));
#34100=CARTESIAN_POINT('Ctrl Pts',(1.88742606273259,-1.,-0.175538155840648));
#34101=CARTESIAN_POINT('Ctrl Pts',(1.88742606273259,1.,-0.175538155840648));
#34102=CARTESIAN_POINT('Ctrl Pts',(1.88188663145367,-1.,-0.175644148889699));
#34103=CARTESIAN_POINT('Ctrl Pts',(1.88188663145367,1.,-0.175644148889699));
#34104=CARTESIAN_POINT('Ctrl Pts',(1.87563767773588,-1.,-0.175563480746485));
#34105=CARTESIAN_POINT('Ctrl Pts',(1.87563767773588,1.,-0.175563480746485));
#34106=CARTESIAN_POINT('Ctrl Pts',(1.86828349694799,-1.,-0.175268337590758));
#34107=CARTESIAN_POINT('Ctrl Pts',(1.86828349694799,1.,-0.175268337590758));
#34108=CARTESIAN_POINT('Ctrl Pts',(1.85948367088837,-1.,-0.17473525927603));
#34109=CARTESIAN_POINT('Ctrl Pts',(1.85948367088837,1.,-0.17473525927603));
#34110=CARTESIAN_POINT('Ctrl Pts',(1.8489811319852,-1.,-0.173946627587732));
#34111=CARTESIAN_POINT('Ctrl Pts',(1.8489811319852,1.,-0.173946627587732));
#34112=CARTESIAN_POINT('Ctrl Pts',(1.83658380527692,-1.,-0.1728894428919));
#34113=CARTESIAN_POINT('Ctrl Pts',(1.83658380527692,1.,-0.1728894428919));
#34114=CARTESIAN_POINT('Ctrl Pts',(1.82215766811545,-1.,-0.171554770204119));
#34115=CARTESIAN_POINT('Ctrl Pts',(1.82215766811545,1.,-0.171554770204119));
#34116=CARTESIAN_POINT('Ctrl Pts',(1.80561530629706,-1.,-0.169936923904608));
#34117=CARTESIAN_POINT('Ctrl Pts',(1.80561530629706,1.,-0.169936923904608));
#34118=CARTESIAN_POINT('Ctrl Pts',(1.7869064998507,-1.,-0.168032772805197));
#34119=CARTESIAN_POINT('Ctrl Pts',(1.7869064998507,1.,-0.168032772805197));
#34120=CARTESIAN_POINT('Ctrl Pts',(1.77018771684844,-1.,-0.1662793551464));
#34121=CARTESIAN_POINT('Ctrl Pts',(1.77018771684844,1.,-0.1662793551464));
#34122=CARTESIAN_POINT('Ctrl Pts',(1.75666056638427,-1.,-0.164834765707159));
#34123=CARTESIAN_POINT('Ctrl Pts',(1.75666056638427,1.,-0.164834765707159));
#34124=CARTESIAN_POINT('Ctrl Pts',(1.7472034950333,-1.,-0.163814161002002));
#34125=CARTESIAN_POINT('Ctrl Pts',(1.7472034950333,1.,-0.163814161002002));
#34126=CARTESIAN_POINT('Ctrl Pts',(1.74236521665491,-1.,-0.163289472382896));
#34127=CARTESIAN_POINT('Ctrl Pts',(1.74236521665491,1.,-0.163289472382896));
#34128=CARTESIAN_POINT('',(2.19890268624765,1.,-0.0694764450219582));
#34129=CARTESIAN_POINT('Ctrl Pts',(2.19890268624765,1.,-0.0694764450219582));
#34130=CARTESIAN_POINT('Ctrl Pts',(2.19777582085423,1.,-0.0701143536325491));
#34131=CARTESIAN_POINT('Ctrl Pts',(2.19552129484002,1.,-0.0713863779526155));
#34132=CARTESIAN_POINT('Ctrl Pts',(2.19213712013662,1.,-0.0732830357306726));
#34133=CARTESIAN_POINT('Ctrl Pts',(2.1876201139953,1.,-0.0757891465836149));
#34134=CARTESIAN_POINT('Ctrl Pts',(2.18196589448887,1.,-0.0788837727685244));
#34135=CARTESIAN_POINT('Ctrl Pts',(2.176303712113,1.,-0.0819402680872767));
#34136=CARTESIAN_POINT('Ctrl Pts',(2.17063357870952,1.,-0.0849584620835374));
#34137=CARTESIAN_POINT('Ctrl Pts',(2.16495552645014,1.,-0.0879381291386924));
#34138=CARTESIAN_POINT('Ctrl Pts',(2.15926961544516,1.,-0.0908789888107267));
#34139=CARTESIAN_POINT('Ctrl Pts',(2.1535759397817,1.,-0.0937807218867645));
#34140=CARTESIAN_POINT('Ctrl Pts',(2.14787463531795,1.,-0.096642985230546));
#34141=CARTESIAN_POINT('Ctrl Pts',(2.14216588396025,1.,-0.0994654261990917));
#34142=CARTESIAN_POINT('Ctrl Pts',(2.13644992667165,1.,-0.102247700556101));
#34143=CARTESIAN_POINT('Ctrl Pts',(2.13072704887293,1.,-0.10498947915274));
#34144=CARTESIAN_POINT('Ctrl Pts',(2.12499752307,1.,-0.10769043523109));
#34145=CARTESIAN_POINT('Ctrl Pts',(2.11926155590865,1.,-0.110350236135025));
#34146=CARTESIAN_POINT('Ctrl Pts',(2.11351924490306,1.,-0.112968534419737));
#34147=CARTESIAN_POINT('Ctrl Pts',(2.10777050261309,1.,-0.115544957687927));
#34148=CARTESIAN_POINT('Ctrl Pts',(2.102015121329,1.,-0.118079107988356));
#34149=CARTESIAN_POINT('Ctrl Pts',(2.0962529286773,1.,-0.120570567965122));
#34150=CARTESIAN_POINT('Ctrl Pts',(2.09048392424825,1.,-0.123018905621083));
#34151=CARTESIAN_POINT('Ctrl Pts',(2.08470840653643,1.,-0.125423679412062));
#34152=CARTESIAN_POINT('Ctrl Pts',(2.07892715110987,1.,-0.12778444527612));
#34153=CARTESIAN_POINT('Ctrl Pts',(2.07314114713063,1.,-0.130100748328404));
#34154=CARTESIAN_POINT('Ctrl Pts',(2.06735123910326,1.,-0.132372111547711));
#34155=CARTESIAN_POINT('Ctrl Pts',(2.06155781517842,1.,-0.134598026192106));
#34156=CARTESIAN_POINT('Ctrl Pts',(2.05576044414264,1.,-0.136777941218044));
#34157=CARTESIAN_POINT('Ctrl Pts',(2.04995762001328,1.,-0.138911255368966));
#34158=CARTESIAN_POINT('Ctrl Pts',(2.04414757947916,1.,-0.140997332152546));
#34159=CARTESIAN_POINT('Ctrl Pts',(2.03832911025912,1.,-0.143035515058209));
#34160=CARTESIAN_POINT('Ctrl Pts',(2.03250223739942,1.,-0.145025140186058));
#34161=CARTESIAN_POINT('Ctrl Pts',(2.02666926182017,1.,-0.146965557332583));
#34162=CARTESIAN_POINT('Ctrl Pts',(2.02083464969894,1.,-0.148856124775337));
#34163=CARTESIAN_POINT('Ctrl Pts',(2.01500291940238,1.,-0.150696157673078));
#34164=CARTESIAN_POINT('Ctrl Pts',(2.00917680318424,1.,-0.15248488362145));
#34165=CARTESIAN_POINT('Ctrl Pts',(2.00335565310543,1.,-0.154221403049722));
#34166=CARTESIAN_POINT('Ctrl Pts',(1.99753284771497,1.,-0.155904629548784));
#34167=CARTESIAN_POINT('Ctrl Pts',(1.99169810931908,1.,-0.157533331459227));
#34168=CARTESIAN_POINT('Ctrl Pts',(1.98584238283292,1.,-0.159106226437299));
#34169=CARTESIAN_POINT('Ctrl Pts',(1.97996195437559,1.,-0.160622060784611));
#34170=CARTESIAN_POINT('Ctrl Pts',(1.97406280235188,1.,-0.162079693556289));
#34171=CARTESIAN_POINT('Ctrl Pts',(1.96816512677967,1.,-0.163478185457734));
#34172=CARTESIAN_POINT('Ctrl Pts',(1.96229379940136,1.,-0.164816568920269));
#34173=CARTESIAN_POINT('Ctrl Pts',(1.9564675971873,1.,-0.166093592002813));
#34174=CARTESIAN_POINT('Ctrl Pts',(1.95069027794294,1.,-0.167307501784476));
#34175=CARTESIAN_POINT('Ctrl Pts',(1.94493757756931,1.,-0.168455741607556));
#34176=CARTESIAN_POINT('Ctrl Pts',(1.93915639211581,1.,-0.169534904817491));
#34177=CARTESIAN_POINT('Ctrl Pts',(1.93329183155539,1.,-0.170541253116202));
#34178=CARTESIAN_POINT('Ctrl Pts',(1.92731093582036,1.,-0.171471191532988));
#34179=CARTESIAN_POINT('Ctrl Pts',(1.9212233439798,1.,-0.172321621259514));
#34180=CARTESIAN_POINT('Ctrl Pts',(1.91511429159527,1.,-0.173090695383496));
#34181=CARTESIAN_POINT('Ctrl Pts',(1.90911693975267,1.,-0.173776635257817));
#34182=CARTESIAN_POINT('Ctrl Pts',(1.90335253862834,1.,-0.174375518661085));
#34183=CARTESIAN_POINT('Ctrl Pts',(1.89788101117132,1.,-0.174879405091263));
#34184=CARTESIAN_POINT('Ctrl Pts',(1.892646301985,1.,-0.175274276190844));
#34185=CARTESIAN_POINT('Ctrl Pts',(1.88742606273259,1.,-0.175538155840648));
#34186=CARTESIAN_POINT('Ctrl Pts',(1.88188663145367,1.,-0.175644148889699));
#34187=CARTESIAN_POINT('Ctrl Pts',(1.87563767773588,1.,-0.175563480746485));
#34188=CARTESIAN_POINT('Ctrl Pts',(1.86828349694799,1.,-0.175268337590758));
#34189=CARTESIAN_POINT('Ctrl Pts',(1.85948367088837,1.,-0.17473525927603));
#34190=CARTESIAN_POINT('Ctrl Pts',(1.8489811319852,1.,-0.173946627587732));
#34191=CARTESIAN_POINT('Ctrl Pts',(1.83658380527692,1.,-0.1728894428919));
#34192=CARTESIAN_POINT('Ctrl Pts',(1.82215766811545,1.,-0.171554770204119));
#34193=CARTESIAN_POINT('Ctrl Pts',(1.80561530629706,1.,-0.169936923904608));
#34194=CARTESIAN_POINT('Ctrl Pts',(1.7869064998507,1.,-0.168032772805197));
#34195=CARTESIAN_POINT('Ctrl Pts',(1.77018771684844,1.,-0.1662793551464));
#34196=CARTESIAN_POINT('Ctrl Pts',(1.75666056638427,1.,-0.164834765707159));
#34197=CARTESIAN_POINT('Ctrl Pts',(1.7472034950333,1.,-0.163814161002002));
#34198=CARTESIAN_POINT('Ctrl Pts',(1.74236521665491,1.,-0.163289472382896));
#34199=CARTESIAN_POINT('',(2.19890268624765,0.,-0.0694764450219582));
#34200=CARTESIAN_POINT('Origin',(2.19890268624765,0.,0.0694764450219582));
#34201=CARTESIAN_POINT('',(2.19890268624765,1.,0.0694764450219582));
#34202=CARTESIAN_POINT('',(2.19890268624765,1.,-0.0694764450219582));
#34203=CARTESIAN_POINT('',(2.19890268624765,0.,0.0694764450219582));
#34204=CARTESIAN_POINT('Ctrl Pts',(1.74236521665491,-1.,0.163289472382896));
#34205=CARTESIAN_POINT('Ctrl Pts',(1.74236521665491,1.,0.163289472382896));
#34206=CARTESIAN_POINT('Ctrl Pts',(1.74720349503904,-1.,0.163814161002474));
#34207=CARTESIAN_POINT('Ctrl Pts',(1.74720349503904,1.,0.163814161002474));
#34208=CARTESIAN_POINT('Ctrl Pts',(1.75666056640041,-1.,0.164834765708484));
#34209=CARTESIAN_POINT('Ctrl Pts',(1.75666056640041,1.,0.164834765708484));
#34210=CARTESIAN_POINT('Ctrl Pts',(1.77018771687692,-1.,0.166279355148738));
#34211=CARTESIAN_POINT('Ctrl Pts',(1.77018771687692,1.,0.166279355148738));
#34212=CARTESIAN_POINT('Ctrl Pts',(1.78690649988931,-1.,0.16803277280837));
#34213=CARTESIAN_POINT('Ctrl Pts',(1.78690649988931,1.,0.16803277280837));
#34214=CARTESIAN_POINT('Ctrl Pts',(1.80561530633924,-1.,0.169936923908078));
#34215=CARTESIAN_POINT('Ctrl Pts',(1.80561530633924,1.,0.169936923908078));
#34216=CARTESIAN_POINT('Ctrl Pts',(1.82215766815414,-1.,0.171554770207306));
#34217=CARTESIAN_POINT('Ctrl Pts',(1.82215766815414,1.,0.171554770207306));
#34218=CARTESIAN_POINT('Ctrl Pts',(1.83658380530747,-1.,0.17288944289442));
#34219=CARTESIAN_POINT('Ctrl Pts',(1.83658380530747,1.,0.17288944289442));
#34220=CARTESIAN_POINT('Ctrl Pts',(1.84898113200543,-1.,0.173946627589401));
#34221=CARTESIAN_POINT('Ctrl Pts',(1.84898113200543,1.,0.173946627589401));
#34222=CARTESIAN_POINT('Ctrl Pts',(1.85948367089838,-1.,0.174735259276856));
#34223=CARTESIAN_POINT('Ctrl Pts',(1.85948367089838,1.,0.174735259276856));
#34224=CARTESIAN_POINT('Ctrl Pts',(1.86828349694972,-1.,0.1752683375909));
#34225=CARTESIAN_POINT('Ctrl Pts',(1.86828349694972,1.,0.1752683375909));
#34226=CARTESIAN_POINT('Ctrl Pts',(1.87563767773249,-1.,0.175563480746205));
#34227=CARTESIAN_POINT('Ctrl Pts',(1.87563767773249,1.,0.175563480746205));
#34228=CARTESIAN_POINT('Ctrl Pts',(1.88188663144846,-1.,0.175644148889271));
#34229=CARTESIAN_POINT('Ctrl Pts',(1.88188663144846,1.,0.175644148889271));
#34230=CARTESIAN_POINT('Ctrl Pts',(1.88742606272818,-1.,0.175538155840286));
#34231=CARTESIAN_POINT('Ctrl Pts',(1.88742606272818,1.,0.175538155840286));
#34232=CARTESIAN_POINT('Ctrl Pts',(1.89264630198279,-1.,0.175274276190664));
#34233=CARTESIAN_POINT('Ctrl Pts',(1.89264630198279,1.,0.175274276190664));
#34234=CARTESIAN_POINT('Ctrl Pts',(1.89788101117148,-1.,0.174879405091277));
#34235=CARTESIAN_POINT('Ctrl Pts',(1.89788101117148,1.,0.174879405091277));
#34236=CARTESIAN_POINT('Ctrl Pts',(1.90335253863003,-1.,0.174375518661222));
#34237=CARTESIAN_POINT('Ctrl Pts',(1.90335253863003,1.,0.174375518661222));
#34238=CARTESIAN_POINT('Ctrl Pts',(1.90911693975475,-1.,0.173776635257983));
#34239=CARTESIAN_POINT('Ctrl Pts',(1.90911693975475,1.,0.173776635257983));
#34240=CARTESIAN_POINT('Ctrl Pts',(1.91511429159681,-1.,0.173090695383619));
#34241=CARTESIAN_POINT('Ctrl Pts',(1.91511429159681,1.,0.173090695383619));
#34242=CARTESIAN_POINT('Ctrl Pts',(1.92122334398034,-1.,0.172321621259556));
#34243=CARTESIAN_POINT('Ctrl Pts',(1.92122334398034,1.,0.172321621259556));
#34244=CARTESIAN_POINT('Ctrl Pts',(1.92731093582,-1.,0.17147119153296));
#34245=CARTESIAN_POINT('Ctrl Pts',(1.92731093582,1.,0.17147119153296));
#34246=CARTESIAN_POINT('Ctrl Pts',(1.93329183155455,-1.,0.170541253116136));
#34247=CARTESIAN_POINT('Ctrl Pts',(1.93329183155455,1.,0.170541253116136));
#34248=CARTESIAN_POINT('Ctrl Pts',(1.93915639211497,-1.,0.169534904817425));
#34249=CARTESIAN_POINT('Ctrl Pts',(1.93915639211497,1.,0.169534904817425));
#34250=CARTESIAN_POINT('Ctrl Pts',(1.94493757756879,-1.,0.168455741607515));
#34251=CARTESIAN_POINT('Ctrl Pts',(1.94493757756879,1.,0.168455741607515));
#34252=CARTESIAN_POINT('Ctrl Pts',(1.95069027794286,-1.,0.167307501784469));
#34253=CARTESIAN_POINT('Ctrl Pts',(1.95069027794286,1.,0.167307501784469));
#34254=CARTESIAN_POINT('Ctrl Pts',(1.95646759718755,-1.,0.166093592002832));
#34255=CARTESIAN_POINT('Ctrl Pts',(1.95646759718755,1.,0.166093592002832));
#34256=CARTESIAN_POINT('Ctrl Pts',(1.96229379940174,-1.,0.1648165689203));
#34257=CARTESIAN_POINT('Ctrl Pts',(1.96229379940174,1.,0.1648165689203));
#34258=CARTESIAN_POINT('Ctrl Pts',(1.96816512678,-1.,0.16347818545776));
#34259=CARTESIAN_POINT('Ctrl Pts',(1.96816512678,1.,0.16347818545776));
#34260=CARTESIAN_POINT('Ctrl Pts',(1.97406280235204,-1.,0.162079693556302));
#34261=CARTESIAN_POINT('Ctrl Pts',(1.97406280235204,1.,0.162079693556302));
#34262=CARTESIAN_POINT('Ctrl Pts',(1.97996195437557,-1.,0.16062206078461));
#34263=CARTESIAN_POINT('Ctrl Pts',(1.97996195437557,1.,0.16062206078461));
#34264=CARTESIAN_POINT('Ctrl Pts',(1.98584238283279,-1.,0.159106226437288));
#34265=CARTESIAN_POINT('Ctrl Pts',(1.98584238283279,1.,0.159106226437288));
#34266=CARTESIAN_POINT('Ctrl Pts',(1.99169810931893,-1.,0.157533331459215));
#34267=CARTESIAN_POINT('Ctrl Pts',(1.99169810931893,1.,0.157533331459215));
#34268=CARTESIAN_POINT('Ctrl Pts',(1.99753284771487,-1.,0.155904629548774));
#34269=CARTESIAN_POINT('Ctrl Pts',(1.99753284771487,1.,0.155904629548774));
#34270=CARTESIAN_POINT('Ctrl Pts',(2.00335565310539,-1.,0.154221403049719));
#34271=CARTESIAN_POINT('Ctrl Pts',(2.00335565310539,1.,0.154221403049719));
#34272=CARTESIAN_POINT('Ctrl Pts',(2.00917680318426,-1.,0.152484883621452));
#34273=CARTESIAN_POINT('Ctrl Pts',(2.00917680318426,1.,0.152484883621452));
#34274=CARTESIAN_POINT('Ctrl Pts',(2.01500291940243,-1.,0.150696157673084));
#34275=CARTESIAN_POINT('Ctrl Pts',(2.01500291940243,1.,0.150696157673084));
#34276=CARTESIAN_POINT('Ctrl Pts',(2.02083464969897,-1.,0.148856124775342));
#34277=CARTESIAN_POINT('Ctrl Pts',(2.02083464969897,1.,0.148856124775342));
#34278=CARTESIAN_POINT('Ctrl Pts',(2.02666926182017,-1.,0.146965557332586));
#34279=CARTESIAN_POINT('Ctrl Pts',(2.02666926182017,1.,0.146965557332586));
#34280=CARTESIAN_POINT('Ctrl Pts',(2.03250223739941,-1.,0.145025140186058));
#34281=CARTESIAN_POINT('Ctrl Pts',(2.03250223739941,1.,0.145025140186058));
#34282=CARTESIAN_POINT('Ctrl Pts',(2.03832911025913,-1.,0.143035515058208));
#34283=CARTESIAN_POINT('Ctrl Pts',(2.03832911025913,1.,0.143035515058208));
#34284=CARTESIAN_POINT('Ctrl Pts',(2.04414757947919,-1.,0.140997332152545));
#34285=CARTESIAN_POINT('Ctrl Pts',(2.04414757947919,1.,0.140997332152545));
#34286=CARTESIAN_POINT('Ctrl Pts',(2.04995762001333,-1.,0.138911255368966));
#34287=CARTESIAN_POINT('Ctrl Pts',(2.04995762001333,1.,0.138911255368966));
#34288=CARTESIAN_POINT('Ctrl Pts',(2.0557604441427,-1.,0.136777941218044));
#34289=CARTESIAN_POINT('Ctrl Pts',(2.0557604441427,1.,0.136777941218044));
#34290=CARTESIAN_POINT('Ctrl Pts',(2.06155781517844,-1.,0.134598026192107));
#34291=CARTESIAN_POINT('Ctrl Pts',(2.06155781517844,1.,0.134598026192107));
#34292=CARTESIAN_POINT('Ctrl Pts',(2.06735123910319,-1.,0.132372111547709));
#34293=CARTESIAN_POINT('Ctrl Pts',(2.06735123910319,1.,0.132372111547709));
#34294=CARTESIAN_POINT('Ctrl Pts',(2.07314114713047,-1.,0.1301007483284));
#34295=CARTESIAN_POINT('Ctrl Pts',(2.07314114713047,1.,0.1301007483284));
#34296=CARTESIAN_POINT('Ctrl Pts',(2.07892715110967,-1.,0.127784445276116));
#34297=CARTESIAN_POINT('Ctrl Pts',(2.07892715110967,1.,0.127784445276116));
#34298=CARTESIAN_POINT('Ctrl Pts',(2.08470840653628,-1.,0.125423679412058));
#34299=CARTESIAN_POINT('Ctrl Pts',(2.08470840653628,1.,0.125423679412058));
#34300=CARTESIAN_POINT('Ctrl Pts',(2.09048392424826,-1.,0.123018905621083));
#34301=CARTESIAN_POINT('Ctrl Pts',(2.09048392424826,1.,0.123018905621083));
#34302=CARTESIAN_POINT('Ctrl Pts',(2.09625292867756,-1.,0.120570567965129));
#34303=CARTESIAN_POINT('Ctrl Pts',(2.09625292867756,1.,0.120570567965129));
#34304=CARTESIAN_POINT('Ctrl Pts',(2.10201512132945,-1.,0.118079107988368));
#34305=CARTESIAN_POINT('Ctrl Pts',(2.10201512132945,1.,0.118079107988368));
#34306=CARTESIAN_POINT('Ctrl Pts',(2.10777050261359,-1.,0.11554495768794));
#34307=CARTESIAN_POINT('Ctrl Pts',(2.10777050261359,1.,0.11554495768794));
#34308=CARTESIAN_POINT('Ctrl Pts',(2.11351924490335,-1.,0.112968534419746));
#34309=CARTESIAN_POINT('Ctrl Pts',(2.11351924490335,1.,0.112968534419746));
#34310=CARTESIAN_POINT('Ctrl Pts',(2.11926155590849,-1.,0.11035023613502));
#34311=CARTESIAN_POINT('Ctrl Pts',(2.11926155590849,1.,0.11035023613502));
#34312=CARTESIAN_POINT('Ctrl Pts',(2.12499752306927,-1.,0.107690435231068));
#34313=CARTESIAN_POINT('Ctrl Pts',(2.12499752306927,1.,0.107690435231068));
#34314=CARTESIAN_POINT('Ctrl Pts',(2.1307270488718,-1.,0.104989479152703));
#34315=CARTESIAN_POINT('Ctrl Pts',(2.1307270488718,1.,0.104989479152703));
#34316=CARTESIAN_POINT('Ctrl Pts',(2.13644992667052,-1.,0.102247700556063));
#34317=CARTESIAN_POINT('Ctrl Pts',(2.13644992667052,1.,0.102247700556063));
#34318=CARTESIAN_POINT('Ctrl Pts',(2.14216588395974,-1.,0.0994654261990741));
#34319=CARTESIAN_POINT('Ctrl Pts',(2.14216588395974,1.,0.0994654261990741));
#34320=CARTESIAN_POINT('Ctrl Pts',(2.14787463531864,-1.,0.0966429852305688));
#34321=CARTESIAN_POINT('Ctrl Pts',(2.14787463531864,1.,0.0966429852305688));
#34322=CARTESIAN_POINT('Ctrl Pts',(2.15357593978377,-1.,0.0937807218868344));
#34323=CARTESIAN_POINT('Ctrl Pts',(2.15357593978377,1.,0.0937807218868344));
#34324=CARTESIAN_POINT('Ctrl Pts',(2.15926961544808,-1.,0.0908789888108265));
#34325=CARTESIAN_POINT('Ctrl Pts',(2.15926961544808,1.,0.0908789888108265));
#34326=CARTESIAN_POINT('Ctrl Pts',(2.16495552645275,-1.,0.0879381291387821));
#34327=CARTESIAN_POINT('Ctrl Pts',(2.16495552645275,1.,0.0879381291387821));
#34328=CARTESIAN_POINT('Ctrl Pts',(2.17063357871031,-1.,0.0849584620835642));
#34329=CARTESIAN_POINT('Ctrl Pts',(2.17063357871031,1.,0.0849584620835642));
#34330=CARTESIAN_POINT('Ctrl Pts',(2.1763037121106,-1.,0.0819402680871938));
#34331=CARTESIAN_POINT('Ctrl Pts',(2.1763037121106,1.,0.0819402680871938));
#34332=CARTESIAN_POINT('Ctrl Pts',(2.18196589448304,-1.,0.0788837727683226));
#34333=CARTESIAN_POINT('Ctrl Pts',(2.18196589448304,1.,0.0788837727683226));
#34334=CARTESIAN_POINT('Ctrl Pts',(2.1876201139874,-1.,0.075789146583341));
#34335=CARTESIAN_POINT('Ctrl Pts',(2.1876201139874,1.,0.075789146583341));
#34336=CARTESIAN_POINT('Ctrl Pts',(2.19213712012956,-1.,0.0732830357304275));
#34337=CARTESIAN_POINT('Ctrl Pts',(2.19213712012956,1.,0.0732830357304275));
#34338=CARTESIAN_POINT('Ctrl Pts',(2.19552129483562,-1.,0.0713863779524626));
#34339=CARTESIAN_POINT('Ctrl Pts',(2.19552129483562,1.,0.0713863779524626));
#34340=CARTESIAN_POINT('Ctrl Pts',(2.19777582085261,-1.,0.0701143536324925));
#34341=CARTESIAN_POINT('Ctrl Pts',(2.19777582085261,1.,0.0701143536324925));
#34342=CARTESIAN_POINT('Ctrl Pts',(2.19890268624765,-1.,0.0694764450219582));
#34343=CARTESIAN_POINT('Ctrl Pts',(2.19890268624765,1.,0.0694764450219582));
#34344=CARTESIAN_POINT('',(1.74236521665491,1.,0.163289472382896));
#34345=CARTESIAN_POINT('Ctrl Pts',(1.74236521665491,1.,0.163289472382896));
#34346=CARTESIAN_POINT('Ctrl Pts',(1.74720349503904,1.,0.163814161002474));
#34347=CARTESIAN_POINT('Ctrl Pts',(1.75666056640041,1.,0.164834765708484));
#34348=CARTESIAN_POINT('Ctrl Pts',(1.77018771687692,1.,0.166279355148738));
#34349=CARTESIAN_POINT('Ctrl Pts',(1.78690649988931,1.,0.16803277280837));
#34350=CARTESIAN_POINT('Ctrl Pts',(1.80561530633924,1.,0.169936923908078));
#34351=CARTESIAN_POINT('Ctrl Pts',(1.82215766815414,1.,0.171554770207306));
#34352=CARTESIAN_POINT('Ctrl Pts',(1.83658380530747,1.,0.17288944289442));
#34353=CARTESIAN_POINT('Ctrl Pts',(1.84898113200543,1.,0.173946627589401));
#34354=CARTESIAN_POINT('Ctrl Pts',(1.85948367089838,1.,0.174735259276856));
#34355=CARTESIAN_POINT('Ctrl Pts',(1.86828349694972,1.,0.1752683375909));
#34356=CARTESIAN_POINT('Ctrl Pts',(1.87563767773249,1.,0.175563480746205));
#34357=CARTESIAN_POINT('Ctrl Pts',(1.88188663144846,1.,0.175644148889271));
#34358=CARTESIAN_POINT('Ctrl Pts',(1.88742606272818,1.,0.175538155840286));
#34359=CARTESIAN_POINT('Ctrl Pts',(1.89264630198279,1.,0.175274276190664));
#34360=CARTESIAN_POINT('Ctrl Pts',(1.89788101117148,1.,0.174879405091277));
#34361=CARTESIAN_POINT('Ctrl Pts',(1.90335253863003,1.,0.174375518661222));
#34362=CARTESIAN_POINT('Ctrl Pts',(1.90911693975475,1.,0.173776635257983));
#34363=CARTESIAN_POINT('Ctrl Pts',(1.91511429159681,1.,0.173090695383619));
#34364=CARTESIAN_POINT('Ctrl Pts',(1.92122334398034,1.,0.172321621259556));
#34365=CARTESIAN_POINT('Ctrl Pts',(1.92731093582,1.,0.17147119153296));
#34366=CARTESIAN_POINT('Ctrl Pts',(1.93329183155455,1.,0.170541253116136));
#34367=CARTESIAN_POINT('Ctrl Pts',(1.93915639211497,1.,0.169534904817425));
#34368=CARTESIAN_POINT('Ctrl Pts',(1.94493757756879,1.,0.168455741607515));
#34369=CARTESIAN_POINT('Ctrl Pts',(1.95069027794286,1.,0.167307501784469));
#34370=CARTESIAN_POINT('Ctrl Pts',(1.95646759718755,1.,0.166093592002832));
#34371=CARTESIAN_POINT('Ctrl Pts',(1.96229379940174,1.,0.1648165689203));
#34372=CARTESIAN_POINT('Ctrl Pts',(1.96816512678,1.,0.16347818545776));
#34373=CARTESIAN_POINT('Ctrl Pts',(1.97406280235204,1.,0.162079693556302));
#34374=CARTESIAN_POINT('Ctrl Pts',(1.97996195437557,1.,0.16062206078461));
#34375=CARTESIAN_POINT('Ctrl Pts',(1.98584238283279,1.,0.159106226437288));
#34376=CARTESIAN_POINT('Ctrl Pts',(1.99169810931893,1.,0.157533331459215));
#34377=CARTESIAN_POINT('Ctrl Pts',(1.99753284771487,1.,0.155904629548774));
#34378=CARTESIAN_POINT('Ctrl Pts',(2.00335565310539,1.,0.154221403049719));
#34379=CARTESIAN_POINT('Ctrl Pts',(2.00917680318426,1.,0.152484883621452));
#34380=CARTESIAN_POINT('Ctrl Pts',(2.01500291940243,1.,0.150696157673084));
#34381=CARTESIAN_POINT('Ctrl Pts',(2.02083464969897,1.,0.148856124775342));
#34382=CARTESIAN_POINT('Ctrl Pts',(2.02666926182017,1.,0.146965557332586));
#34383=CARTESIAN_POINT('Ctrl Pts',(2.03250223739941,1.,0.145025140186058));
#34384=CARTESIAN_POINT('Ctrl Pts',(2.03832911025913,1.,0.143035515058208));
#34385=CARTESIAN_POINT('Ctrl Pts',(2.04414757947919,1.,0.140997332152545));
#34386=CARTESIAN_POINT('Ctrl Pts',(2.04995762001333,1.,0.138911255368966));
#34387=CARTESIAN_POINT('Ctrl Pts',(2.0557604441427,1.,0.136777941218044));
#34388=CARTESIAN_POINT('Ctrl Pts',(2.06155781517844,1.,0.134598026192107));
#34389=CARTESIAN_POINT('Ctrl Pts',(2.06735123910319,1.,0.132372111547709));
#34390=CARTESIAN_POINT('Ctrl Pts',(2.07314114713047,1.,0.1301007483284));
#34391=CARTESIAN_POINT('Ctrl Pts',(2.07892715110967,1.,0.127784445276116));
#34392=CARTESIAN_POINT('Ctrl Pts',(2.08470840653628,1.,0.125423679412058));
#34393=CARTESIAN_POINT('Ctrl Pts',(2.09048392424826,1.,0.123018905621083));
#34394=CARTESIAN_POINT('Ctrl Pts',(2.09625292867756,1.,0.120570567965129));
#34395=CARTESIAN_POINT('Ctrl Pts',(2.10201512132945,1.,0.118079107988368));
#34396=CARTESIAN_POINT('Ctrl Pts',(2.10777050261359,1.,0.11554495768794));
#34397=CARTESIAN_POINT('Ctrl Pts',(2.11351924490335,1.,0.112968534419746));
#34398=CARTESIAN_POINT('Ctrl Pts',(2.11926155590849,1.,0.11035023613502));
#34399=CARTESIAN_POINT('Ctrl Pts',(2.12499752306927,1.,0.107690435231068));
#34400=CARTESIAN_POINT('Ctrl Pts',(2.1307270488718,1.,0.104989479152703));
#34401=CARTESIAN_POINT('Ctrl Pts',(2.13644992667052,1.,0.102247700556063));
#34402=CARTESIAN_POINT('Ctrl Pts',(2.14216588395974,1.,0.0994654261990741));
#34403=CARTESIAN_POINT('Ctrl Pts',(2.14787463531864,1.,0.0966429852305688));
#34404=CARTESIAN_POINT('Ctrl Pts',(2.15357593978377,1.,0.0937807218868344));
#34405=CARTESIAN_POINT('Ctrl Pts',(2.15926961544808,1.,0.0908789888108265));
#34406=CARTESIAN_POINT('Ctrl Pts',(2.16495552645275,1.,0.0879381291387821));
#34407=CARTESIAN_POINT('Ctrl Pts',(2.17063357871031,1.,0.0849584620835642));
#34408=CARTESIAN_POINT('Ctrl Pts',(2.1763037121106,1.,0.0819402680871938));
#34409=CARTESIAN_POINT('Ctrl Pts',(2.18196589448304,1.,0.0788837727683226));
#34410=CARTESIAN_POINT('Ctrl Pts',(2.1876201139874,1.,0.075789146583341));
#34411=CARTESIAN_POINT('Ctrl Pts',(2.19213712012956,1.,0.0732830357304275));
#34412=CARTESIAN_POINT('Ctrl Pts',(2.19552129483562,1.,0.0713863779524626));
#34413=CARTESIAN_POINT('Ctrl Pts',(2.19777582085261,1.,0.0701143536324925));
#34414=CARTESIAN_POINT('Ctrl Pts',(2.19890268624765,1.,0.0694764450219582));
#34415=CARTESIAN_POINT('',(1.74236521665491,0.,0.163289472382896));
#34416=CARTESIAN_POINT('Origin',(0.,1.,0.));
#34417=CARTESIAN_POINT('Origin',(0.,1.,0.));
#34418=CARTESIAN_POINT('Origin',(0.,0.,0.));
#34790=UNCERTAINTY_MEASURE_WITH_UNIT(LENGTH_MEASURE(0.001),#34852,
'DISTANCE_ACCURACY_VALUE',
'Maximum model space distance between geometric entities at asserted c
onnectivities');
#34797=UNCERTAINTY_MEASURE_WITH_UNIT(LENGTH_MEASURE(0.001),#34852,
'DISTANCE_ACCURACY_VALUE',
'Maximum model space distance between geometric entities at asserted c
onnectivities');
#34844=(
GEOMETRIC_REPRESENTATION_CONTEXT(3)
GLOBAL_UNCERTAINTY_ASSIGNED_CONTEXT((#34790))
GLOBAL_UNIT_ASSIGNED_CONTEXT((#34852,#34854,#34855))
REPRESENTATION_CONTEXT('','3D')
);
#34851=(
GEOMETRIC_REPRESENTATION_CONTEXT(3)
GLOBAL_UNCERTAINTY_ASSIGNED_CONTEXT((#34797))
GLOBAL_UNIT_ASSIGNED_CONTEXT((#34852,#34854,#34855))
REPRESENTATION_CONTEXT('','3D')
);
#34852=(
LENGTH_UNIT()
NAMED_UNIT(*)
SI_UNIT(.CENTI.,.METRE.)
);
#34854=(
NAMED_UNIT(*)
PLANE_ANGLE_UNIT()
SI_UNIT($,.RADIAN.)
);
#34855=(
NAMED_UNIT(*)
SI_UNIT($,.STERADIAN.)
SOLID_ANGLE_UNIT()
);
#34902=SHAPE_DEFINITION_REPRESENTATION(#34963,#35119);
#34963=PRODUCT_DEFINITION_SHAPE('',$,#35173);
#35119=SHAPE_REPRESENTATION('',(#15322),#34844);
#35126=PRODUCT_DEFINITION_CONTEXT('part definition',#35287,'design');
#35173=PRODUCT_DEFINITION('Spur Gear - Module 2, 20 Teeth, 12 mm Bore',
'Spur Gear - Module 2, 20 Teeth, 12 mm Bore',#35226,#35126);
#35226=PRODUCT_DEFINITION_FORMATION('',$,#35335);
#35287=APPLICATION_CONTEXT(
'Core Data for Automotive Mechanical Design Process');
#35288=PRODUCT_CONTEXT('part definition',#35287,'mechanical');
#35335=PRODUCT('Spur Gear - Module 2, 20 Teeth, 12 mm Bore',
'Spur Gear - Module 2, 20 Teeth, 12 mm Bore',
'Spur Gear - Module 2, 20 Teeth, 12 mm Bore',(#35288));
#35419=COLOUR_RGB('Off White',0.89,0.88,0.83);
#35420=FILL_AREA_STYLE_COLOUR('',#35419);
#35421=FILL_AREA_STYLE('',(#35420));
#35422=SURFACE_STYLE_FILL_AREA(#35421);
#35423=SURFACE_SIDE_STYLE('',(#35422));
#35424=SURFACE_STYLE_USAGE(.BOTH.,#35423);
#35425=PRESENTATION_STYLE_ASSIGNMENT((#35424));
ENDSEC;
END-ISO-10303-21;
